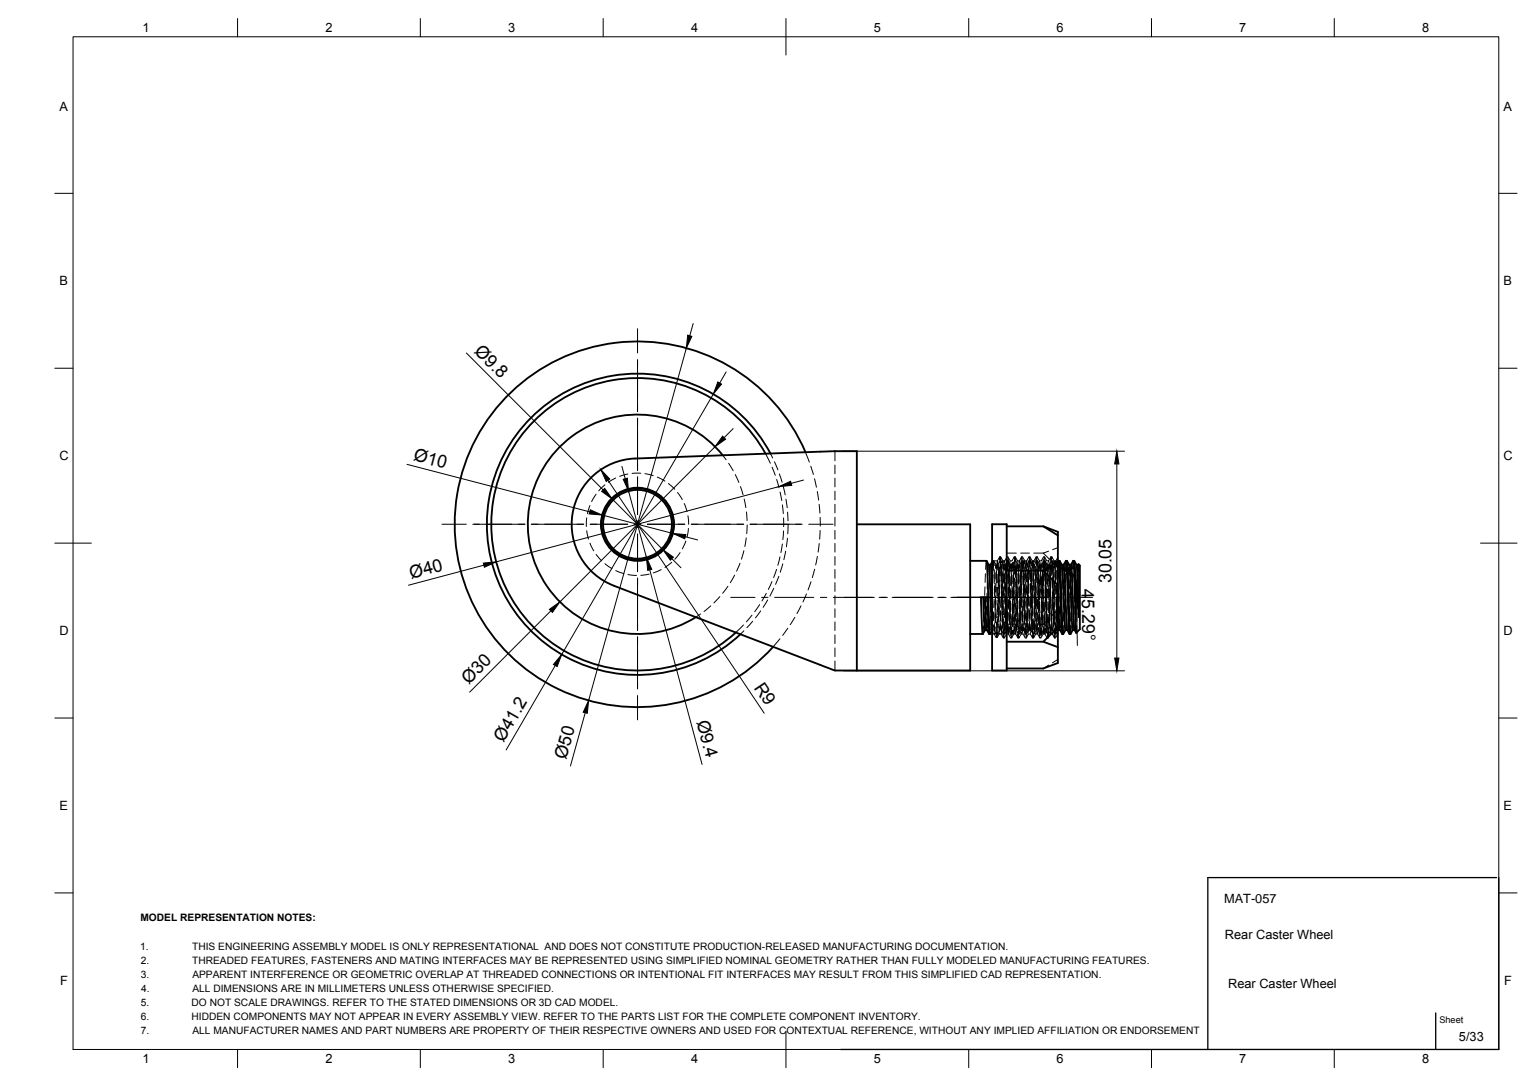
ISO-10303-21;
HEADER;
/* Generated by software containing ST-Developer
 * from STEP Tools, Inc. (www.steptools.com) 
 */

FILE_DESCRIPTION(
/* description */ ('STEP AP214', 'CAx-IF Rec.Pracs.---Representation and Presentation of Product Manufa
cturing Information (PMI)---4.0---2014-10-13'),
/* implementation_level */ '2;1');

FILE_NAME(
/* name */ 'Rear Caster Wheel.step',
/* time_stamp */ '2026-10-28T23:34:22+01:00',
/* author */ (''),
/* organization */ (''),
/* preprocessor_version */ 'ST-DEVELOPER v20.2',
/* originating_system */ 'Autodesk Translation Framework v15.17.0.0',
/* authorisation */ '');

FILE_SCHEMA (('AP242_MANAGED_MODEL_BASED_3D_ENGINEERING_MIM_LF { 1 0 10303 442 2 1 4 }'));
ENDSEC;

DATA;
#10=MECHANICAL_DESIGN_GEOMETRIC_PRESENTATION_REPRESENTATION('',(#273,#274,#275,#276),#27807);
#36=(
BOUNDED_CURVE()
B_SPLINE_CURVE(2,(#23410,#23411,#23412,#23413,#23414,#23415,#23416,#23417,
#23418),.UNSPECIFIED.,.F.,.F.)
B_SPLINE_CURVE_WITH_KNOTS((3,2,2,2,3),(0.964285714285714,0.973214285714286,
0.982142857142857,0.991071428571429,1.),.UNSPECIFIED.)
CURVE()
GEOMETRIC_REPRESENTATION_ITEM()
RATIONAL_B_SPLINE_CURVE((1.,0.923879532511287,1.,0.923879532511287,1.,0.923879532511287,
1.,0.923879532511287,1.))
REPRESENTATION_ITEM('')
);
#37=(
BOUNDED_CURVE()
B_SPLINE_CURVE(2,(#23421,#23422,#23423,#23424,#23425,#23426,#23427,#23428,
#23429),.UNSPECIFIED.,.F.,.F.)
B_SPLINE_CURVE_WITH_KNOTS((3,2,2,2,3),(0.964285714285714,0.973214285714286,
0.982142857142857,0.991071428571429,1.),.UNSPECIFIED.)
CURVE()
GEOMETRIC_REPRESENTATION_ITEM()
RATIONAL_B_SPLINE_CURVE((1.,0.923879532511287,1.,0.923879532511287,1.,0.923879532511287,
1.,0.923879532511287,1.))
REPRESENTATION_ITEM('')
);
#38=(
BOUNDED_CURVE()
B_SPLINE_CURVE(2,(#23434,#23435,#23436,#23437,#23438,#23439,#23440,#23441,
#23442,#23443,#23444,#23445,#23446,#23447,#23448,#23449,#23450),
 .UNSPECIFIED.,.F.,.F.)
B_SPLINE_CURVE_WITH_KNOTS((3,2,2,2,2,2,2,2,3),(0.892857142857143,0.901785714285714,
0.910714285714286,0.919642857142857,0.928571428571429,0.9375,0.946428571428571,
0.955357142857143,0.964285714285714),.UNSPECIFIED.)
CURVE()
GEOMETRIC_REPRESENTATION_ITEM()
RATIONAL_B_SPLINE_CURVE((1.,0.923879532511287,1.,0.923879532511287,1.,0.923879532511287,
1.,0.923879532511287,1.,0.923879532511287,1.,0.923879532511287,1.,0.923879532511287,
1.,0.923879532511287,1.))
REPRESENTATION_ITEM('')
);
#39=(
BOUNDED_CURVE()
B_SPLINE_CURVE(2,(#23451,#23452,#23453,#23454,#23455,#23456,#23457,#23458,
#23459,#23460,#23461,#23462,#23463,#23464,#23465,#23466,#23467),
 .UNSPECIFIED.,.F.,.F.)
B_SPLINE_CURVE_WITH_KNOTS((3,2,2,2,2,2,2,2,3),(0.892857142857143,0.901785714285714,
0.910714285714286,0.919642857142857,0.928571428571429,0.9375,0.946428571428571,
0.955357142857143,0.964285714285714),.UNSPECIFIED.)
CURVE()
GEOMETRIC_REPRESENTATION_ITEM()
RATIONAL_B_SPLINE_CURVE((1.,0.923879532511287,1.,0.923879532511287,1.,0.923879532511287,
1.,0.923879532511287,1.,0.923879532511287,1.,0.923879532511287,1.,0.923879532511287,
1.,0.923879532511287,1.))
REPRESENTATION_ITEM('')
);
#40=(
BOUNDED_CURVE()
B_SPLINE_CURVE(2,(#23472,#23473,#23474,#23475,#23476,#23477,#23478,#23479,
#23480,#23481,#23482,#23483,#23484,#23485,#23486,#23487,#23488),
 .UNSPECIFIED.,.F.,.F.)
B_SPLINE_CURVE_WITH_KNOTS((3,2,2,2,2,2,2,2,3),(0.821428571428571,0.830357142857143,
0.839285714285714,0.848214285714286,0.857142857142857,0.866071428571429,
0.875,0.883928571428571,0.892857142857143),.UNSPECIFIED.)
CURVE()
GEOMETRIC_REPRESENTATION_ITEM()
RATIONAL_B_SPLINE_CURVE((1.,0.923879532511287,1.,0.923879532511287,1.,0.923879532511287,
1.,0.923879532511287,1.,0.923879532511287,1.,0.923879532511287,1.,0.923879532511287,
1.,0.923879532511287,1.))
REPRESENTATION_ITEM('')
);
#41=(
BOUNDED_CURVE()
B_SPLINE_CURVE(2,(#23489,#23490,#23491,#23492,#23493,#23494,#23495,#23496,
#23497,#23498,#23499,#23500,#23501,#23502,#23503,#23504,#23505),
 .UNSPECIFIED.,.F.,.F.)
B_SPLINE_CURVE_WITH_KNOTS((3,2,2,2,2,2,2,2,3),(0.821428571428571,0.830357142857143,
0.839285714285714,0.848214285714286,0.857142857142857,0.866071428571429,
0.875,0.883928571428571,0.892857142857143),.UNSPECIFIED.)
CURVE()
GEOMETRIC_REPRESENTATION_ITEM()
RATIONAL_B_SPLINE_CURVE((1.,0.923879532511287,1.,0.923879532511287,1.,0.923879532511287,
1.,0.923879532511287,1.,0.923879532511287,1.,0.923879532511287,1.,0.923879532511287,
1.,0.923879532511287,1.))
REPRESENTATION_ITEM('')
);
#42=(
BOUNDED_CURVE()
B_SPLINE_CURVE(2,(#23510,#23511,#23512,#23513,#23514,#23515,#23516,#23517,
#23518,#23519,#23520,#23521,#23522,#23523,#23524,#23525,#23526),
 .UNSPECIFIED.,.F.,.F.)
B_SPLINE_CURVE_WITH_KNOTS((3,2,2,2,2,2,2,2,3),(0.75,0.758928571428571,0.767857142857143,
0.776785714285714,0.785714285714286,0.794642857142857,0.803571428571429,
0.8125,0.821428571428571),.UNSPECIFIED.)
CURVE()
GEOMETRIC_REPRESENTATION_ITEM()
RATIONAL_B_SPLINE_CURVE((1.,0.923879532511287,1.,0.923879532511287,1.,0.923879532511287,
1.,0.923879532511287,1.,0.923879532511287,1.,0.923879532511287,1.,0.923879532511287,
1.,0.923879532511287,1.))
REPRESENTATION_ITEM('')
);
#43=(
BOUNDED_CURVE()
B_SPLINE_CURVE(2,(#23527,#23528,#23529,#23530,#23531,#23532,#23533,#23534,
#23535,#23536,#23537,#23538,#23539,#23540,#23541,#23542,#23543),
 .UNSPECIFIED.,.F.,.F.)
B_SPLINE_CURVE_WITH_KNOTS((3,2,2,2,2,2,2,2,3),(0.75,0.758928571428571,0.767857142857143,
0.776785714285714,0.785714285714286,0.794642857142857,0.803571428571429,
0.8125,0.821428571428571),.UNSPECIFIED.)
CURVE()
GEOMETRIC_REPRESENTATION_ITEM()
RATIONAL_B_SPLINE_CURVE((1.,0.923879532511287,1.,0.923879532511287,1.,0.923879532511287,
1.,0.923879532511287,1.,0.923879532511287,1.,0.923879532511287,1.,0.923879532511287,
1.,0.923879532511287,1.))
REPRESENTATION_ITEM('')
);
#44=(
BOUNDED_CURVE()
B_SPLINE_CURVE(2,(#23548,#23549,#23550,#23551,#23552,#23553,#23554,#23555,
#23556,#23557,#23558,#23559,#23560,#23561,#23562,#23563,#23564),
 .UNSPECIFIED.,.F.,.F.)
B_SPLINE_CURVE_WITH_KNOTS((3,2,2,2,2,2,2,2,3),(0.678571428571429,0.6875,
0.696428571428571,0.705357142857143,0.714285714285714,0.723214285714286,
0.732142857142857,0.741071428571429,0.75),.UNSPECIFIED.)
CURVE()
GEOMETRIC_REPRESENTATION_ITEM()
RATIONAL_B_SPLINE_CURVE((1.,0.923879532511287,1.,0.923879532511287,1.,0.923879532511287,
1.,0.923879532511287,1.,0.923879532511287,1.,0.923879532511287,1.,0.923879532511287,
1.,0.923879532511287,1.))
REPRESENTATION_ITEM('')
);
#45=(
BOUNDED_CURVE()
B_SPLINE_CURVE(2,(#23565,#23566,#23567,#23568,#23569,#23570,#23571,#23572,
#23573,#23574,#23575,#23576,#23577,#23578,#23579,#23580,#23581),
 .UNSPECIFIED.,.F.,.F.)
B_SPLINE_CURVE_WITH_KNOTS((3,2,2,2,2,2,2,2,3),(0.678571428571428,0.6875,
0.696428571428571,0.705357142857143,0.714285714285714,0.723214285714286,
0.732142857142857,0.741071428571429,0.75),.UNSPECIFIED.)
CURVE()
GEOMETRIC_REPRESENTATION_ITEM()
RATIONAL_B_SPLINE_CURVE((1.,0.923879532511287,1.,0.923879532511287,1.,0.923879532511287,
1.,0.923879532511287,1.,0.923879532511287,1.,0.923879532511287,1.,0.923879532511287,
1.,0.923879532511287,1.))
REPRESENTATION_ITEM('')
);
#46=(
BOUNDED_CURVE()
B_SPLINE_CURVE(2,(#23586,#23587,#23588,#23589,#23590,#23591,#23592,#23593,
#23594,#23595,#23596,#23597,#23598,#23599,#23600,#23601,#23602),
 .UNSPECIFIED.,.F.,.F.)
B_SPLINE_CURVE_WITH_KNOTS((3,2,2,2,2,2,2,2,3),(0.607142857142857,0.616071428571429,
0.625,0.633928571428571,0.642857142857143,0.651785714285714,0.660714285714286,
0.669642857142857,0.678571428571429),.UNSPECIFIED.)
CURVE()
GEOMETRIC_REPRESENTATION_ITEM()
RATIONAL_B_SPLINE_CURVE((1.,0.923879532511287,1.,0.923879532511287,1.,0.923879532511287,
1.,0.923879532511287,1.,0.923879532511287,1.,0.923879532511287,1.,0.923879532511287,
1.,0.923879532511287,1.))
REPRESENTATION_ITEM('')
);
#47=(
BOUNDED_CURVE()
B_SPLINE_CURVE(2,(#23603,#23604,#23605,#23606,#23607,#23608,#23609,#23610,
#23611,#23612,#23613,#23614,#23615,#23616,#23617,#23618,#23619),
 .UNSPECIFIED.,.F.,.F.)
B_SPLINE_CURVE_WITH_KNOTS((3,2,2,2,2,2,2,2,3),(0.607142857142857,0.616071428571429,
0.625,0.633928571428571,0.642857142857143,0.651785714285714,0.660714285714286,
0.669642857142857,0.678571428571428),.UNSPECIFIED.)
CURVE()
GEOMETRIC_REPRESENTATION_ITEM()
RATIONAL_B_SPLINE_CURVE((1.,0.923879532511287,1.,0.923879532511287,1.,0.923879532511287,
1.,0.923879532511287,1.,0.923879532511287,1.,0.923879532511287,1.,0.923879532511287,
1.,0.923879532511287,1.))
REPRESENTATION_ITEM('')
);
#48=(
BOUNDED_CURVE()
B_SPLINE_CURVE(2,(#23624,#23625,#23626,#23627,#23628,#23629,#23630,#23631,
#23632,#23633,#23634,#23635,#23636,#23637,#23638,#23639,#23640),
 .UNSPECIFIED.,.F.,.F.)
B_SPLINE_CURVE_WITH_KNOTS((3,2,2,2,2,2,2,2,3),(0.535714285714286,0.544642857142857,
0.553571428571429,0.5625,0.571428571428571,0.580357142857143,0.589285714285714,
0.598214285714286,0.607142857142857),.UNSPECIFIED.)
CURVE()
GEOMETRIC_REPRESENTATION_ITEM()
RATIONAL_B_SPLINE_CURVE((1.,0.923879532511287,1.,0.923879532511287,1.,0.923879532511287,
1.,0.923879532511287,1.,0.923879532511287,1.,0.923879532511287,1.,0.923879532511287,
1.,0.923879532511287,1.))
REPRESENTATION_ITEM('')
);
#49=(
BOUNDED_CURVE()
B_SPLINE_CURVE(2,(#23641,#23642,#23643,#23644,#23645,#23646,#23647,#23648,
#23649,#23650,#23651,#23652,#23653,#23654,#23655,#23656,#23657),
 .UNSPECIFIED.,.F.,.F.)
B_SPLINE_CURVE_WITH_KNOTS((3,2,2,2,2,2,2,2,3),(0.535714285714286,0.544642857142857,
0.553571428571429,0.5625,0.571428571428571,0.580357142857143,0.589285714285714,
0.598214285714286,0.607142857142857),.UNSPECIFIED.)
CURVE()
GEOMETRIC_REPRESENTATION_ITEM()
RATIONAL_B_SPLINE_CURVE((1.,0.923879532511287,1.,0.923879532511287,1.,0.923879532511287,
1.,0.923879532511287,1.,0.923879532511287,1.,0.923879532511287,1.,0.923879532511287,
1.,0.923879532511287,1.))
REPRESENTATION_ITEM('')
);
#50=(
BOUNDED_CURVE()
B_SPLINE_CURVE(2,(#23662,#23663,#23664,#23665,#23666,#23667,#23668,#23669,
#23670,#23671,#23672,#23673,#23674,#23675,#23676,#23677,#23678),
 .UNSPECIFIED.,.F.,.F.)
B_SPLINE_CURVE_WITH_KNOTS((3,2,2,2,2,2,2,2,3),(0.464285714285714,0.473214285714286,
0.482142857142857,0.491071428571429,0.5,0.508928571428571,0.517857142857143,
0.526785714285714,0.535714285714286),.UNSPECIFIED.)
CURVE()
GEOMETRIC_REPRESENTATION_ITEM()
RATIONAL_B_SPLINE_CURVE((1.,0.923879532511287,1.,0.923879532511287,1.,0.923879532511287,
1.,0.923879532511287,1.,0.923879532511287,1.,0.923879532511287,1.,0.923879532511287,
1.,0.923879532511287,1.))
REPRESENTATION_ITEM('')
);
#51=(
BOUNDED_CURVE()
B_SPLINE_CURVE(2,(#23679,#23680,#23681,#23682,#23683,#23684,#23685,#23686,
#23687,#23688,#23689,#23690,#23691,#23692,#23693,#23694,#23695),
 .UNSPECIFIED.,.F.,.F.)
B_SPLINE_CURVE_WITH_KNOTS((3,2,2,2,2,2,2,2,3),(0.464285714285714,0.473214285714286,
0.482142857142857,0.491071428571429,0.5,0.508928571428571,0.517857142857143,
0.526785714285714,0.535714285714286),.UNSPECIFIED.)
CURVE()
GEOMETRIC_REPRESENTATION_ITEM()
RATIONAL_B_SPLINE_CURVE((1.,0.923879532511287,1.,0.923879532511287,1.,0.923879532511287,
1.,0.923879532511287,1.,0.923879532511287,1.,0.923879532511287,1.,0.923879532511287,
1.,0.923879532511287,1.))
REPRESENTATION_ITEM('')
);
#52=(
BOUNDED_CURVE()
B_SPLINE_CURVE(2,(#23700,#23701,#23702,#23703,#23704,#23705,#23706,#23707,
#23708,#23709,#23710,#23711,#23712,#23713,#23714,#23715,#23716),
 .UNSPECIFIED.,.F.,.F.)
B_SPLINE_CURVE_WITH_KNOTS((3,2,2,2,2,2,2,2,3),(0.392857142857143,0.401785714285714,
0.410714285714286,0.419642857142857,0.428571428571429,0.4375,0.446428571428571,
0.455357142857143,0.464285714285714),.UNSPECIFIED.)
CURVE()
GEOMETRIC_REPRESENTATION_ITEM()
RATIONAL_B_SPLINE_CURVE((1.,0.923879532511287,1.,0.923879532511287,1.,0.923879532511287,
1.,0.923879532511287,1.,0.923879532511287,1.,0.923879532511287,1.,0.923879532511287,
1.,0.923879532511287,1.))
REPRESENTATION_ITEM('')
);
#53=(
BOUNDED_CURVE()
B_SPLINE_CURVE(2,(#23717,#23718,#23719,#23720,#23721,#23722,#23723,#23724,
#23725,#23726,#23727,#23728,#23729,#23730,#23731,#23732,#23733),
 .UNSPECIFIED.,.F.,.F.)
B_SPLINE_CURVE_WITH_KNOTS((3,2,2,2,2,2,2,2,3),(0.392857142857143,0.401785714285714,
0.410714285714286,0.419642857142857,0.428571428571429,0.4375,0.446428571428571,
0.455357142857143,0.464285714285714),.UNSPECIFIED.)
CURVE()
GEOMETRIC_REPRESENTATION_ITEM()
RATIONAL_B_SPLINE_CURVE((1.,0.923879532511287,1.,0.923879532511287,1.,0.923879532511287,
1.,0.923879532511287,1.,0.923879532511287,1.,0.923879532511287,1.,0.923879532511287,
1.,0.923879532511287,1.))
REPRESENTATION_ITEM('')
);
#54=(
BOUNDED_CURVE()
B_SPLINE_CURVE(2,(#23738,#23739,#23740,#23741,#23742,#23743,#23744,#23745,
#23746,#23747,#23748,#23749,#23750,#23751,#23752,#23753,#23754),
 .UNSPECIFIED.,.F.,.F.)
B_SPLINE_CURVE_WITH_KNOTS((3,2,2,2,2,2,2,2,3),(0.321428571428571,0.330357142857143,
0.339285714285714,0.348214285714286,0.357142857142857,0.366071428571429,
0.375,0.383928571428571,0.392857142857143),.UNSPECIFIED.)
CURVE()
GEOMETRIC_REPRESENTATION_ITEM()
RATIONAL_B_SPLINE_CURVE((1.,0.923879532511287,1.,0.923879532511287,1.,0.923879532511287,
1.,0.923879532511287,1.,0.923879532511287,1.,0.923879532511287,1.,0.923879532511287,
1.,0.923879532511287,1.))
REPRESENTATION_ITEM('')
);
#55=(
BOUNDED_CURVE()
B_SPLINE_CURVE(2,(#23755,#23756,#23757,#23758,#23759,#23760,#23761,#23762,
#23763,#23764,#23765,#23766,#23767,#23768,#23769,#23770,#23771),
 .UNSPECIFIED.,.F.,.F.)
B_SPLINE_CURVE_WITH_KNOTS((3,2,2,2,2,2,2,2,3),(0.321428571428571,0.330357142857143,
0.339285714285714,0.348214285714286,0.357142857142857,0.366071428571429,
0.375,0.383928571428571,0.392857142857143),.UNSPECIFIED.)
CURVE()
GEOMETRIC_REPRESENTATION_ITEM()
RATIONAL_B_SPLINE_CURVE((1.,0.923879532511287,1.,0.923879532511287,1.,0.923879532511287,
1.,0.923879532511287,1.,0.923879532511287,1.,0.923879532511287,1.,0.923879532511287,
1.,0.923879532511287,1.))
REPRESENTATION_ITEM('')
);
#56=(
BOUNDED_CURVE()
B_SPLINE_CURVE(2,(#23776,#23777,#23778,#23779,#23780,#23781,#23782,#23783,
#23784,#23785,#23786,#23787,#23788,#23789,#23790,#23791,#23792),
 .UNSPECIFIED.,.F.,.F.)
B_SPLINE_CURVE_WITH_KNOTS((3,2,2,2,2,2,2,2,3),(0.25,0.258928571428571,0.267857142857143,
0.276785714285714,0.285714285714286,0.294642857142857,0.303571428571429,
0.3125,0.321428571428571),.UNSPECIFIED.)
CURVE()
GEOMETRIC_REPRESENTATION_ITEM()
RATIONAL_B_SPLINE_CURVE((1.,0.923879532511287,1.,0.923879532511287,1.,0.923879532511287,
1.,0.923879532511287,1.,0.923879532511287,1.,0.923879532511287,1.,0.923879532511287,
1.,0.923879532511287,1.))
REPRESENTATION_ITEM('')
);
#57=(
BOUNDED_CURVE()
B_SPLINE_CURVE(2,(#23793,#23794,#23795,#23796,#23797,#23798,#23799,#23800,
#23801,#23802,#23803,#23804,#23805,#23806,#23807,#23808,#23809),
 .UNSPECIFIED.,.F.,.F.)
B_SPLINE_CURVE_WITH_KNOTS((3,2,2,2,2,2,2,2,3),(0.25,0.258928571428571,0.267857142857143,
0.276785714285714,0.285714285714286,0.294642857142857,0.303571428571429,
0.3125,0.321428571428571),.UNSPECIFIED.)
CURVE()
GEOMETRIC_REPRESENTATION_ITEM()
RATIONAL_B_SPLINE_CURVE((1.,0.923879532511287,1.,0.923879532511287,1.,0.923879532511287,
1.,0.923879532511287,1.,0.923879532511287,1.,0.923879532511287,1.,0.923879532511287,
1.,0.923879532511287,1.))
REPRESENTATION_ITEM('')
);
#58=(
BOUNDED_CURVE()
B_SPLINE_CURVE(2,(#23814,#23815,#23816,#23817,#23818,#23819,#23820,#23821,
#23822,#23823,#23824,#23825,#23826,#23827,#23828,#23829,#23830),
 .UNSPECIFIED.,.F.,.F.)
B_SPLINE_CURVE_WITH_KNOTS((3,2,2,2,2,2,2,2,3),(0.178571428571429,0.1875,
0.196428571428571,0.205357142857143,0.214285714285714,0.223214285714286,
0.232142857142857,0.241071428571429,0.25),.UNSPECIFIED.)
CURVE()
GEOMETRIC_REPRESENTATION_ITEM()
RATIONAL_B_SPLINE_CURVE((1.,0.923879532511287,1.,0.923879532511287,1.,0.923879532511287,
1.,0.923879532511287,1.,0.923879532511287,1.,0.923879532511287,1.,0.923879532511287,
1.,0.923879532511287,1.))
REPRESENTATION_ITEM('')
);
#59=(
BOUNDED_CURVE()
B_SPLINE_CURVE(2,(#23831,#23832,#23833,#23834,#23835,#23836,#23837,#23838,
#23839,#23840,#23841,#23842,#23843,#23844,#23845,#23846,#23847),
 .UNSPECIFIED.,.F.,.F.)
B_SPLINE_CURVE_WITH_KNOTS((3,2,2,2,2,2,2,2,3),(0.178571428571429,0.1875,
0.196428571428571,0.205357142857143,0.214285714285714,0.223214285714286,
0.232142857142857,0.241071428571429,0.25),.UNSPECIFIED.)
CURVE()
GEOMETRIC_REPRESENTATION_ITEM()
RATIONAL_B_SPLINE_CURVE((1.,0.923879532511287,1.,0.923879532511287,1.,0.923879532511287,
1.,0.923879532511287,1.,0.923879532511287,1.,0.923879532511287,1.,0.923879532511287,
1.,0.923879532511287,1.))
REPRESENTATION_ITEM('')
);
#60=(
BOUNDED_CURVE()
B_SPLINE_CURVE(2,(#23852,#23853,#23854,#23855,#23856,#23857,#23858,#23859,
#23860,#23861,#23862,#23863,#23864,#23865,#23866,#23867,#23868),
 .UNSPECIFIED.,.F.,.F.)
B_SPLINE_CURVE_WITH_KNOTS((3,2,2,2,2,2,2,2,3),(0.107142857142857,0.116071428571429,
0.125,0.133928571428571,0.142857142857143,0.151785714285714,0.160714285714286,
0.169642857142857,0.178571428571429),.UNSPECIFIED.)
CURVE()
GEOMETRIC_REPRESENTATION_ITEM()
RATIONAL_B_SPLINE_CURVE((1.,0.923879532511287,1.,0.923879532511287,1.,0.923879532511287,
1.,0.923879532511287,1.,0.923879532511287,1.,0.923879532511287,1.,0.923879532511287,
1.,0.923879532511287,1.))
REPRESENTATION_ITEM('')
);
#61=(
BOUNDED_CURVE()
B_SPLINE_CURVE(2,(#23869,#23870,#23871,#23872,#23873,#23874,#23875,#23876,
#23877,#23878,#23879,#23880,#23881,#23882,#23883,#23884,#23885),
 .UNSPECIFIED.,.F.,.F.)
B_SPLINE_CURVE_WITH_KNOTS((3,2,2,2,2,2,2,2,3),(0.107142857142857,0.116071428571429,
0.125,0.133928571428571,0.142857142857143,0.151785714285714,0.160714285714286,
0.169642857142857,0.178571428571429),.UNSPECIFIED.)
CURVE()
GEOMETRIC_REPRESENTATION_ITEM()
RATIONAL_B_SPLINE_CURVE((1.,0.923879532511287,1.,0.923879532511287,1.,0.923879532511287,
1.,0.923879532511287,1.,0.923879532511287,1.,0.923879532511287,1.,0.923879532511287,
1.,0.923879532511287,1.))
REPRESENTATION_ITEM('')
);
#62=(
BOUNDED_CURVE()
B_SPLINE_CURVE(2,(#25481,#25482,#25483,#25484,#25485,#25486,#25487),
 .UNSPECIFIED.,.F.,.F.)
B_SPLINE_CURVE_WITH_KNOTS((3,2,2,3),(0.0819392927096003,0.0892857142857143,
0.0982142857142857,0.107142857142857),.UNSPECIFIED.)
CURVE()
GEOMETRIC_REPRESENTATION_ITEM()
RATIONAL_B_SPLINE_CURVE((0.977803170316603,0.937368138988787,1.,0.923879532511287,
1.,0.923879532511287,1.))
REPRESENTATION_ITEM('')
);
#63=(
BOUNDED_CURVE()
B_SPLINE_CURVE(2,(#25489,#25490,#25491,#25492,#25493,#25494,#25495,#25496,
#25497,#25498,#25499),.UNSPECIFIED.,.F.,.F.)
B_SPLINE_CURVE_WITH_KNOTS((3,2,2,2,2,3),(0.0640821498524563,0.0714285714285714,
0.0803571428571429,0.0892857142857143,0.0982142857142857,0.107142857142857),
 .UNSPECIFIED.)
CURVE()
GEOMETRIC_REPRESENTATION_ITEM()
RATIONAL_B_SPLINE_CURVE((0.977803170316615,0.937368138988778,1.,0.923879532511287,
1.,0.923879532511287,1.,0.923879532511287,1.,0.923879532511287,1.))
REPRESENTATION_ITEM('')
);
#64=(
BOUNDED_CURVE()
B_SPLINE_CURVE(2,(#25959,#25960,#25961,#25962,#25963,#25964,#25965,#25966,
#25967,#25968,#25969,#25970,#25971,#25972,#25973),.UNSPECIFIED.,.F.,.F.)
B_SPLINE_CURVE_WITH_KNOTS((3,2,2,2,2,2,2,3),(0.168750000131362,0.175,0.1875,
0.2,0.2125,0.225,0.2375,0.25),.UNSPECIFIED.)
CURVE()
GEOMETRIC_REPRESENTATION_ITEM()
RATIONAL_B_SPLINE_CURVE((0.961939766255643,0.961939767055589,1.,0.923879532511287,
1.,0.923879532511287,1.,0.923879532511287,1.,0.923879532511287,1.,0.923879532511287,
1.,0.923879532511287,1.))
REPRESENTATION_ITEM('')
);
#65=(
BOUNDED_CURVE()
B_SPLINE_CURVE(2,(#25976,#25977,#25978,#25979,#25980,#25981,#25982,#25983,
#25984,#25985,#25986,#25987,#25988,#25989,#25990,#25991,#25992),
 .UNSPECIFIED.,.F.,.F.)
B_SPLINE_CURVE_WITH_KNOTS((3,2,2,2,2,2,2,2,3),(0.156250000131362,0.1625,
0.175,0.1875,0.2,0.2125,0.225,0.2375,0.25),.UNSPECIFIED.)
CURVE()
GEOMETRIC_REPRESENTATION_ITEM()
RATIONAL_B_SPLINE_CURVE((0.961939766255643,0.961939767055589,1.,0.923879532511287,
1.,0.923879532511287,1.,0.923879532511287,1.,0.923879532511287,1.,0.923879532511287,
1.,0.923879532511287,1.,0.923879532511287,1.))
REPRESENTATION_ITEM('')
);
#66=(
BOUNDED_CURVE()
B_SPLINE_CURVE(2,(#25997,#25998,#25999,#26000,#26001,#26002,#26003,#26004,
#26005,#26006,#26007,#26008,#26009,#26010,#26011,#26012,#26013),
 .UNSPECIFIED.,.F.,.F.)
B_SPLINE_CURVE_WITH_KNOTS((3,2,2,2,2,2,2,2,3),(0.25,0.2625,0.275,0.2875,
0.3,0.3125,0.325,0.3375,0.35),.UNSPECIFIED.)
CURVE()
GEOMETRIC_REPRESENTATION_ITEM()
RATIONAL_B_SPLINE_CURVE((1.,0.923879532511287,1.,0.923879532511287,1.,0.923879532511287,
1.,0.923879532511287,1.,0.923879532511287,1.,0.923879532511287,1.,0.923879532511287,
1.,0.923879532511287,1.))
REPRESENTATION_ITEM('')
);
#67=(
BOUNDED_CURVE()
B_SPLINE_CURVE(2,(#26014,#26015,#26016,#26017,#26018,#26019,#26020,#26021,
#26022,#26023,#26024,#26025,#26026,#26027,#26028,#26029,#26030),
 .UNSPECIFIED.,.F.,.F.)
B_SPLINE_CURVE_WITH_KNOTS((3,2,2,2,2,2,2,2,3),(0.25,0.2625,0.275,0.2875,
0.3,0.3125,0.325,0.3375,0.35),.UNSPECIFIED.)
CURVE()
GEOMETRIC_REPRESENTATION_ITEM()
RATIONAL_B_SPLINE_CURVE((1.,0.923879532511287,1.,0.923879532511287,1.,0.923879532511287,
1.,0.923879532511287,1.,0.923879532511287,1.,0.923879532511287,1.,0.923879532511287,
1.,0.923879532511287,1.))
REPRESENTATION_ITEM('')
);
#68=(
BOUNDED_CURVE()
B_SPLINE_CURVE(2,(#26035,#26036,#26037,#26038,#26039,#26040,#26041,#26042,
#26043,#26044,#26045,#26046,#26047,#26048,#26049,#26050,#26051),
 .UNSPECIFIED.,.F.,.F.)
B_SPLINE_CURVE_WITH_KNOTS((3,2,2,2,2,2,2,2,3),(0.35,0.3625,0.375,0.3875,
0.4,0.4125,0.425,0.4375,0.45),.UNSPECIFIED.)
CURVE()
GEOMETRIC_REPRESENTATION_ITEM()
RATIONAL_B_SPLINE_CURVE((1.,0.923879532511287,1.,0.923879532511287,1.,0.923879532511287,
1.,0.923879532511287,1.,0.923879532511287,1.,0.923879532511287,1.,0.923879532511287,
1.,0.923879532511287,1.))
REPRESENTATION_ITEM('')
);
#69=(
BOUNDED_CURVE()
B_SPLINE_CURVE(2,(#26052,#26053,#26054,#26055,#26056,#26057,#26058,#26059,
#26060,#26061,#26062,#26063,#26064,#26065,#26066,#26067,#26068),
 .UNSPECIFIED.,.F.,.F.)
B_SPLINE_CURVE_WITH_KNOTS((3,2,2,2,2,2,2,2,3),(0.35,0.3625,0.375,0.3875,
0.4,0.4125,0.425,0.4375,0.45),.UNSPECIFIED.)
CURVE()
GEOMETRIC_REPRESENTATION_ITEM()
RATIONAL_B_SPLINE_CURVE((1.,0.923879532511287,1.,0.923879532511287,1.,0.923879532511287,
1.,0.923879532511287,1.,0.923879532511287,1.,0.923879532511287,1.,0.923879532511287,
1.,0.923879532511287,1.))
REPRESENTATION_ITEM('')
);
#70=(
BOUNDED_CURVE()
B_SPLINE_CURVE(2,(#26073,#26074,#26075,#26076,#26077,#26078,#26079,#26080,
#26081,#26082,#26083,#26084,#26085,#26086,#26087,#26088,#26089),
 .UNSPECIFIED.,.F.,.F.)
B_SPLINE_CURVE_WITH_KNOTS((3,2,2,2,2,2,2,2,3),(0.45,0.4625,0.475,0.4875,
0.5,0.5125,0.525,0.5375,0.55),.UNSPECIFIED.)
CURVE()
GEOMETRIC_REPRESENTATION_ITEM()
RATIONAL_B_SPLINE_CURVE((1.,0.923879532511287,1.,0.923879532511287,1.,0.923879532511287,
1.,0.923879532511287,1.,0.923879532511287,1.,0.923879532511287,1.,0.923879532511287,
1.,0.923879532511287,1.))
REPRESENTATION_ITEM('')
);
#71=(
BOUNDED_CURVE()
B_SPLINE_CURVE(2,(#26090,#26091,#26092,#26093,#26094,#26095,#26096,#26097,
#26098,#26099,#26100,#26101,#26102,#26103,#26104,#26105,#26106),
 .UNSPECIFIED.,.F.,.F.)
B_SPLINE_CURVE_WITH_KNOTS((3,2,2,2,2,2,2,2,3),(0.45,0.4625,0.475,0.4875,
0.5,0.5125,0.525,0.5375,0.55),.UNSPECIFIED.)
CURVE()
GEOMETRIC_REPRESENTATION_ITEM()
RATIONAL_B_SPLINE_CURVE((1.,0.923879532511287,1.,0.923879532511287,1.,0.923879532511287,
1.,0.923879532511287,1.,0.923879532511287,1.,0.923879532511287,1.,0.923879532511287,
1.,0.923879532511287,1.))
REPRESENTATION_ITEM('')
);
#72=(
BOUNDED_CURVE()
B_SPLINE_CURVE(2,(#26111,#26112,#26113,#26114,#26115,#26116,#26117,#26118,
#26119,#26120,#26121,#26122,#26123,#26124,#26125,#26126,#26127),
 .UNSPECIFIED.,.F.,.F.)
B_SPLINE_CURVE_WITH_KNOTS((3,2,2,2,2,2,2,2,3),(0.55,0.5625,0.575,0.5875,
0.6,0.6125,0.625,0.6375,0.65),.UNSPECIFIED.)
CURVE()
GEOMETRIC_REPRESENTATION_ITEM()
RATIONAL_B_SPLINE_CURVE((1.,0.923879532511287,1.,0.923879532511287,1.,0.923879532511287,
1.,0.923879532511287,1.,0.923879532511287,1.,0.923879532511287,1.,0.923879532511287,
1.,0.923879532511287,1.))
REPRESENTATION_ITEM('')
);
#73=(
BOUNDED_CURVE()
B_SPLINE_CURVE(2,(#26128,#26129,#26130,#26131,#26132,#26133,#26134,#26135,
#26136,#26137,#26138,#26139,#26140,#26141,#26142,#26143,#26144),
 .UNSPECIFIED.,.F.,.F.)
B_SPLINE_CURVE_WITH_KNOTS((3,2,2,2,2,2,2,2,3),(0.55,0.5625,0.575,0.5875,
0.6,0.6125,0.625,0.6375,0.65),.UNSPECIFIED.)
CURVE()
GEOMETRIC_REPRESENTATION_ITEM()
RATIONAL_B_SPLINE_CURVE((1.,0.923879532511287,1.,0.923879532511287,1.,0.923879532511287,
1.,0.923879532511287,1.,0.923879532511287,1.,0.923879532511287,1.,0.923879532511287,
1.,0.923879532511287,1.))
REPRESENTATION_ITEM('')
);
#74=(
BOUNDED_CURVE()
B_SPLINE_CURVE(2,(#26149,#26150,#26151,#26152,#26153,#26154,#26155,#26156,
#26157,#26158,#26159,#26160,#26161,#26162,#26163,#26164,#26165),
 .UNSPECIFIED.,.F.,.F.)
B_SPLINE_CURVE_WITH_KNOTS((3,2,2,2,2,2,2,2,3),(0.65,0.6625,0.675,0.6875,
0.7,0.7125,0.725,0.7375,0.75),.UNSPECIFIED.)
CURVE()
GEOMETRIC_REPRESENTATION_ITEM()
RATIONAL_B_SPLINE_CURVE((1.,0.923879532511287,1.,0.923879532511287,1.,0.923879532511287,
1.,0.923879532511287,1.,0.923879532511287,1.,0.923879532511287,1.,0.923879532511287,
1.,0.923879532511287,1.))
REPRESENTATION_ITEM('')
);
#75=(
BOUNDED_CURVE()
B_SPLINE_CURVE(2,(#26166,#26167,#26168,#26169,#26170,#26171,#26172,#26173,
#26174,#26175,#26176,#26177,#26178,#26179,#26180,#26181,#26182),
 .UNSPECIFIED.,.F.,.F.)
B_SPLINE_CURVE_WITH_KNOTS((3,2,2,2,2,2,2,2,3),(0.65,0.6625,0.675,0.6875,
0.7,0.7125,0.725,0.7375,0.75),.UNSPECIFIED.)
CURVE()
GEOMETRIC_REPRESENTATION_ITEM()
RATIONAL_B_SPLINE_CURVE((1.,0.923879532511287,1.,0.923879532511287,1.,0.923879532511287,
1.,0.923879532511287,1.,0.923879532511287,1.,0.923879532511287,1.,0.923879532511287,
1.,0.923879532511287,1.))
REPRESENTATION_ITEM('')
);
#76=(
BOUNDED_CURVE()
B_SPLINE_CURVE(2,(#26187,#26188,#26189,#26190,#26191,#26192,#26193,#26194,
#26195,#26196,#26197,#26198,#26199,#26200,#26201,#26202,#26203),
 .UNSPECIFIED.,.F.,.F.)
B_SPLINE_CURVE_WITH_KNOTS((3,2,2,2,2,2,2,2,3),(0.75,0.7625,0.775,0.7875,
0.8,0.8125,0.825,0.8375,0.85),.UNSPECIFIED.)
CURVE()
GEOMETRIC_REPRESENTATION_ITEM()
RATIONAL_B_SPLINE_CURVE((1.,0.923879532511287,1.,0.923879532511287,1.,0.923879532511287,
1.,0.923879532511287,1.,0.923879532511287,1.,0.923879532511287,1.,0.923879532511287,
1.,0.923879532511287,1.))
REPRESENTATION_ITEM('')
);
#77=(
BOUNDED_CURVE()
B_SPLINE_CURVE(2,(#26204,#26205,#26206,#26207,#26208,#26209,#26210,#26211,
#26212,#26213,#26214,#26215,#26216,#26217,#26218,#26219,#26220),
 .UNSPECIFIED.,.F.,.F.)
B_SPLINE_CURVE_WITH_KNOTS((3,2,2,2,2,2,2,2,3),(0.75,0.7625,0.775,0.7875,
0.8,0.8125,0.825,0.8375,0.85),.UNSPECIFIED.)
CURVE()
GEOMETRIC_REPRESENTATION_ITEM()
RATIONAL_B_SPLINE_CURVE((1.,0.923879532511287,1.,0.923879532511287,1.,0.923879532511287,
1.,0.923879532511287,1.,0.923879532511287,1.,0.923879532511287,1.,0.923879532511287,
1.,0.923879532511287,1.))
REPRESENTATION_ITEM('')
);
#78=(
BOUNDED_CURVE()
B_SPLINE_CURVE(2,(#26226,#26227,#26228,#26229,#26230,#26231,#26232,#26233,
#26234),.UNSPECIFIED.,.F.,.F.)
B_SPLINE_CURVE_WITH_KNOTS((3,2,2,2,3),(0.95,0.9625,0.975,0.9875,1.),
 .UNSPECIFIED.)
CURVE()
GEOMETRIC_REPRESENTATION_ITEM()
RATIONAL_B_SPLINE_CURVE((1.,0.923879532511287,1.,0.923879532511287,1.,0.923879532511287,
1.,0.923879532511287,1.))
REPRESENTATION_ITEM('')
);
#79=(
BOUNDED_CURVE()
B_SPLINE_CURVE(2,(#26237,#26238,#26239,#26240,#26241,#26242,#26243,#26244,
#26245),.UNSPECIFIED.,.F.,.F.)
B_SPLINE_CURVE_WITH_KNOTS((3,2,2,2,3),(0.95,0.9625,0.975,0.9875,1.),
 .UNSPECIFIED.)
CURVE()
GEOMETRIC_REPRESENTATION_ITEM()
RATIONAL_B_SPLINE_CURVE((1.,0.923879532511287,1.,0.923879532511287,1.,0.923879532511287,
1.,0.923879532511287,1.))
REPRESENTATION_ITEM('')
);
#80=(
BOUNDED_CURVE()
B_SPLINE_CURVE(2,(#27008,#27009,#27010,#27011,#27012,#27013,#27014,#27015,
#27016,#27017,#27018,#27019,#27020,#27021,#27022,#27023,#27024),
 .UNSPECIFIED.,.F.,.F.)
B_SPLINE_CURVE_WITH_KNOTS((3,2,2,2,2,2,2,2,3),(0.85,0.8625,0.875,0.8875,
0.9,0.9125,0.925,0.9375,0.95),.UNSPECIFIED.)
CURVE()
GEOMETRIC_REPRESENTATION_ITEM()
RATIONAL_B_SPLINE_CURVE((1.,0.923879532511287,1.,0.923879532511287,1.,0.923879532511287,
1.,0.923879532511287,1.,0.923879532511287,1.,0.923879532511287,1.,0.923879532511287,
1.,0.923879532511287,1.))
REPRESENTATION_ITEM('')
);
#81=(
BOUNDED_CURVE()
B_SPLINE_CURVE(2,(#27025,#27026,#27027,#27028,#27029,#27030,#27031,#27032,
#27033,#27034,#27035,#27036,#27037,#27038,#27039,#27040,#27041),
 .UNSPECIFIED.,.F.,.F.)
B_SPLINE_CURVE_WITH_KNOTS((3,2,2,2,2,2,2,2,3),(0.85,0.8625,0.875,0.8875,
0.9,0.9125,0.925,0.9375,0.95),.UNSPECIFIED.)
CURVE()
GEOMETRIC_REPRESENTATION_ITEM()
RATIONAL_B_SPLINE_CURVE((1.,0.923879532511287,1.,0.923879532511287,1.,0.923879532511287,
1.,0.923879532511287,1.,0.923879532511287,1.,0.923879532511287,1.,0.923879532511287,
1.,0.923879532511287,1.))
REPRESENTATION_ITEM('')
);
#225=SHAPE_REPRESENTATION_RELATIONSHIP('SRR','None',#27924,#247);
#247=ADVANCED_BREP_SHAPE_REPRESENTATION('',(#302,#303,#304,#305),#27804);
#273=STYLED_ITEM('',(#28091),#302);
#274=STYLED_ITEM('',(#28091),#303);
#275=STYLED_ITEM('',(#28091),#304);
#276=STYLED_ITEM('',(#28091),#305);
#302=MANIFOLD_SOLID_BREP('Body1',#12049);
#303=MANIFOLD_SOLID_BREP('Body2',#12050);
#304=MANIFOLD_SOLID_BREP('Body3',#12051);
#305=MANIFOLD_SOLID_BREP('Body4',#12052);
#323=(
BOUNDED_SURFACE()
B_SPLINE_SURFACE(1,2,((#25031,#25032,#25033,#25034,#25035,#25036,#25037,
#25038,#25039,#25040,#25041,#25042,#25043,#25044,#25045,#25046,#25047,#25048,
#25049,#25050,#25051,#25052,#25053,#25054,#25055,#25056,#25057,#25058,#25059,
#25060,#25061,#25062,#25063,#25064,#25065,#25066,#25067,#25068,#25069,#25070,
#25071,#25072,#25073,#25074,#25075,#25076,#25077,#25078,#25079,#25080,#25081,
#25082,#25083,#25084,#25085,#25086,#25087,#25088,#25089,#25090,#25091,#25092,
#25093,#25094,#25095,#25096,#25097,#25098,#25099,#25100,#25101,#25102,#25103,
#25104,#25105,#25106,#25107,#25108,#25109,#25110,#25111,#25112,#25113,#25114,
#25115,#25116,#25117,#25118,#25119,#25120,#25121,#25122,#25123,#25124,#25125,
#25126,#25127,#25128,#25129,#25130,#25131,#25132,#25133,#25134,#25135,#25136,
#25137,#25138,#25139,#25140,#25141,#25142,#25143,#25144,#25145,#25146,#25147,
#25148,#25149,#25150,#25151,#25152,#25153,#25154,#25155,#25156,#25157,#25158,
#25159,#25160,#25161,#25162,#25163,#25164,#25165,#25166,#25167,#25168,#25169,
#25170,#25171,#25172,#25173,#25174,#25175,#25176,#25177,#25178,#25179,#25180,
#25181,#25182,#25183,#25184,#25185,#25186,#25187,#25188,#25189,#25190,#25191,
#25192,#25193,#25194,#25195,#25196,#25197,#25198,#25199,#25200,#25201,#25202,
#25203,#25204,#25205,#25206,#25207,#25208,#25209,#25210,#25211,#25212,#25213,
#25214,#25215,#25216,#25217,#25218,#25219,#25220,#25221,#25222,#25223,#25224,
#25225,#25226,#25227,#25228,#25229,#25230,#25231,#25232,#25233,#25234,#25235,
#25236,#25237,#25238,#25239,#25240,#25241,#25242,#25243,#25244,#25245,#25246,
#25247,#25248,#25249,#25250,#25251,#25252,#25253,#25254,#25255),(#25256,
#25257,#25258,#25259,#25260,#25261,#25262,#25263,#25264,#25265,#25266,#25267,
#25268,#25269,#25270,#25271,#25272,#25273,#25274,#25275,#25276,#25277,#25278,
#25279,#25280,#25281,#25282,#25283,#25284,#25285,#25286,#25287,#25288,#25289,
#25290,#25291,#25292,#25293,#25294,#25295,#25296,#25297,#25298,#25299,#25300,
#25301,#25302,#25303,#25304,#25305,#25306,#25307,#25308,#25309,#25310,#25311,
#25312,#25313,#25314,#25315,#25316,#25317,#25318,#25319,#25320,#25321,#25322,
#25323,#25324,#25325,#25326,#25327,#25328,#25329,#25330,#25331,#25332,#25333,
#25334,#25335,#25336,#25337,#25338,#25339,#25340,#25341,#25342,#25343,#25344,
#25345,#25346,#25347,#25348,#25349,#25350,#25351,#25352,#25353,#25354,#25355,
#25356,#25357,#25358,#25359,#25360,#25361,#25362,#25363,#25364,#25365,#25366,
#25367,#25368,#25369,#25370,#25371,#25372,#25373,#25374,#25375,#25376,#25377,
#25378,#25379,#25380,#25381,#25382,#25383,#25384,#25385,#25386,#25387,#25388,
#25389,#25390,#25391,#25392,#25393,#25394,#25395,#25396,#25397,#25398,#25399,
#25400,#25401,#25402,#25403,#25404,#25405,#25406,#25407,#25408,#25409,#25410,
#25411,#25412,#25413,#25414,#25415,#25416,#25417,#25418,#25419,#25420,#25421,
#25422,#25423,#25424,#25425,#25426,#25427,#25428,#25429,#25430,#25431,#25432,
#25433,#25434,#25435,#25436,#25437,#25438,#25439,#25440,#25441,#25442,#25443,
#25444,#25445,#25446,#25447,#25448,#25449,#25450,#25451,#25452,#25453,#25454,
#25455,#25456,#25457,#25458,#25459,#25460,#25461,#25462,#25463,#25464,#25465,
#25466,#25467,#25468,#25469,#25470,#25471,#25472,#25473,#25474,#25475,#25476,
#25477,#25478,#25479,#25480)),.UNSPECIFIED.,.F.,.F.,.F.)
B_SPLINE_SURFACE_WITH_KNOTS((2,2),(3,2,2,2,2,2,2,2,2,2,2,2,2,2,2,2,2,2,
2,2,2,2,2,2,2,2,2,2,2,2,2,2,2,2,2,2,2,2,2,2,2,2,2,2,2,2,2,2,2,2,2,2,2,2,
2,2,2,2,2,2,2,2,2,2,2,2,2,2,2,2,2,2,2,2,2,2,2,2,2,2,2,2,2,2,2,2,2,2,2,2,
2,2,2,2,2,2,2,2,2,2,2,2,2,2,2,2,2,2,2,2,2,2,3),(0.,1.00000154805557),(0.,
0.00892857142857143,0.0178571428571429,0.0267857142857143,0.0357142857142857,
0.0446428571428571,0.0535714285714286,0.0625,0.0714285714285714,0.0803571428571429,
0.0892857142857143,0.0982142857142857,0.107142857142857,0.116071428571429,
0.125,0.133928571428571,0.142857142857143,0.151785714285714,0.160714285714286,
0.169642857142857,0.178571428571429,0.1875,0.196428571428571,0.205357142857143,
0.214285714285714,0.223214285714286,0.232142857142857,0.241071428571429,
0.25,0.258928571428571,0.267857142857143,0.276785714285714,0.285714285714286,
0.294642857142857,0.303571428571429,0.3125,0.321428571428571,0.330357142857143,
0.339285714285714,0.348214285714286,0.357142857142857,0.366071428571429,
0.375,0.383928571428571,0.392857142857143,0.401785714285714,0.410714285714286,
0.419642857142857,0.428571428571429,0.4375,0.446428571428571,0.455357142857143,
0.464285714285714,0.473214285714286,0.482142857142857,0.491071428571429,
0.5,0.508928571428571,0.517857142857143,0.526785714285714,0.535714285714286,
0.544642857142857,0.553571428571429,0.5625,0.571428571428571,0.580357142857143,
0.589285714285714,0.598214285714286,0.607142857142857,0.616071428571429,
0.625,0.633928571428571,0.642857142857143,0.651785714285714,0.660714285714286,
0.669642857142857,0.678571428571429,0.6875,0.696428571428571,0.705357142857143,
0.714285714285714,0.723214285714286,0.732142857142857,0.741071428571429,
0.75,0.758928571428571,0.767857142857143,0.776785714285714,0.785714285714286,
0.794642857142857,0.803571428571429,0.8125,0.821428571428571,0.830357142857143,
0.839285714285714,0.848214285714286,0.857142857142857,0.866071428571429,
0.875,0.883928571428571,0.892857142857143,0.901785714285714,0.910714285714286,
0.919642857142857,0.928571428571429,0.9375,0.946428571428571,0.955357142857143,
0.964285714285714,0.973214285714286,0.982142857142857,0.991071428571429,
1.),.UNSPECIFIED.)
GEOMETRIC_REPRESENTATION_ITEM()
RATIONAL_B_SPLINE_SURFACE(((1.,0.923879532511287,1.,0.923879532511287,1.,
0.923879532511287,1.,0.923879532511287,1.,0.923879532511287,1.,0.923879532511287,
1.,0.923879532511287,1.,0.923879532511287,1.,0.923879532511287,1.,0.923879532511287,
1.,0.923879532511287,1.,0.923879532511287,1.,0.923879532511287,1.,0.923879532511287,
1.,0.923879532511287,1.,0.923879532511287,1.,0.923879532511287,1.,0.923879532511287,
1.,0.923879532511287,1.,0.923879532511287,1.,0.923879532511287,1.,0.923879532511287,
1.,0.923879532511287,1.,0.923879532511287,1.,0.923879532511287,1.,0.923879532511287,
1.,0.923879532511287,1.,0.923879532511287,1.,0.923879532511287,1.,0.923879532511287,
1.,0.923879532511287,1.,0.923879532511287,1.,0.923879532511287,1.,0.923879532511287,
1.,0.923879532511287,1.,0.923879532511287,1.,0.923879532511287,1.,0.923879532511287,
1.,0.923879532511287,1.,0.923879532511287,1.,0.923879532511287,1.,0.923879532511287,
1.,0.923879532511287,1.,0.923879532511287,1.,0.923879532511287,1.,0.923879532511287,
1.,0.923879532511287,1.,0.923879532511287,1.,0.923879532511287,1.,0.923879532511287,
1.,0.923879532511287,1.,0.923879532511287,1.,0.923879532511287,1.,0.923879532511287,
1.,0.923879532511287,1.,0.923879532511287,1.,0.923879532511287,1.,0.923879532511287,
1.,0.923879532511287,1.,0.923879532511287,1.,0.923879532511287,1.,0.923879532511287,
1.,0.923879532511287,1.,0.923879532511287,1.,0.923879532511287,1.,0.923879532511287,
1.,0.923879532511287,1.,0.923879532511287,1.,0.923879532511287,1.,0.923879532511287,
1.,0.923879532511287,1.,0.923879532511287,1.,0.923879532511287,1.,0.923879532511287,
1.,0.923879532511287,1.,0.923879532511287,1.,0.923879532511287,1.,0.923879532511287,
1.,0.923879532511287,1.,0.923879532511287,1.,0.923879532511287,1.,0.923879532511287,
1.,0.923879532511287,1.,0.923879532511287,1.,0.923879532511287,1.,0.923879532511287,
1.,0.923879532511287,1.,0.923879532511287,1.,0.923879532511287,1.,0.923879532511287,
1.,0.923879532511287,1.,0.923879532511287,1.,0.923879532511287,1.,0.923879532511287,
1.,0.923879532511287,1.,0.923879532511287,1.,0.923879532511287,1.,0.923879532511287,
1.,0.923879532511287,1.,0.923879532511287,1.,0.923879532511287,1.,0.923879532511287,
1.,0.923879532511287,1.,0.923879532511287,1.,0.923879532511287,1.,0.923879532511287,
1.,0.923879532511287,1.,0.923879532511287,1.,0.923879532511287,1.,0.923879532511287,
1.,0.923879532511287,1.,0.923879532511287,1.),(1.,0.923879532511287,1.,
0.923879532511287,1.,0.923879532511287,1.,0.923879532511287,1.,0.923879532511287,
1.,0.923879532511287,1.,0.923879532511287,1.,0.923879532511287,1.,0.923879532511287,
1.,0.923879532511287,1.,0.923879532511287,1.,0.923879532511287,1.,0.923879532511287,
1.,0.923879532511287,1.,0.923879532511287,1.,0.923879532511287,1.,0.923879532511287,
1.,0.923879532511287,1.,0.923879532511287,1.,0.923879532511287,1.,0.923879532511287,
1.,0.923879532511287,1.,0.923879532511287,1.,0.923879532511287,1.,0.923879532511287,
1.,0.923879532511287,1.,0.923879532511287,1.,0.923879532511287,1.,0.923879532511287,
1.,0.923879532511287,1.,0.923879532511287,1.,0.923879532511287,1.,0.923879532511287,
1.,0.923879532511287,1.,0.923879532511287,1.,0.923879532511287,1.,0.923879532511287,
1.,0.923879532511287,1.,0.923879532511287,1.,0.923879532511287,1.,0.923879532511287,
1.,0.923879532511287,1.,0.923879532511287,1.,0.923879532511287,1.,0.923879532511287,
1.,0.923879532511287,1.,0.923879532511287,1.,0.923879532511287,1.,0.923879532511287,
1.,0.923879532511287,1.,0.923879532511287,1.,0.923879532511287,1.,0.923879532511287,
1.,0.923879532511287,1.,0.923879532511287,1.,0.923879532511287,1.,0.923879532511287,
1.,0.923879532511287,1.,0.923879532511287,1.,0.923879532511287,1.,0.923879532511287,
1.,0.923879532511287,1.,0.923879532511287,1.,0.923879532511287,1.,0.923879532511287,
1.,0.923879532511287,1.,0.923879532511287,1.,0.923879532511287,1.,0.923879532511287,
1.,0.923879532511287,1.,0.923879532511287,1.,0.923879532511287,1.,0.923879532511287,
1.,0.923879532511287,1.,0.923879532511287,1.,0.923879532511287,1.,0.923879532511287,
1.,0.923879532511287,1.,0.923879532511287,1.,0.923879532511287,1.,0.923879532511287,
1.,0.923879532511287,1.,0.923879532511287,1.,0.923879532511287,1.,0.923879532511287,
1.,0.923879532511287,1.,0.923879532511287,1.,0.923879532511287,1.,0.923879532511287,
1.,0.923879532511287,1.,0.923879532511287,1.,0.923879532511287,1.,0.923879532511287,
1.,0.923879532511287,1.,0.923879532511287,1.,0.923879532511287,1.,0.923879532511287,
1.,0.923879532511287,1.,0.923879532511287,1.,0.923879532511287,1.,0.923879532511287,
1.,0.923879532511287,1.,0.923879532511287,1.,0.923879532511287,1.,0.923879532511287,
1.,0.923879532511287,1.,0.923879532511287,1.,0.923879532511287,1.,0.923879532511287,
1.,0.923879532511287,1.,0.923879532511287,1.,0.923879532511287,1.)))
REPRESENTATION_ITEM('')
SURFACE()
);
#324=(
BOUNDED_SURFACE()
B_SPLINE_SURFACE(1,2,((#25500,#25501,#25502,#25503,#25504,#25505,#25506,
#25507,#25508,#25509,#25510,#25511,#25512,#25513,#25514,#25515,#25516,#25517,
#25518,#25519,#25520,#25521,#25522,#25523,#25524,#25525,#25526,#25527,#25528,
#25529,#25530,#25531,#25532,#25533,#25534,#25535,#25536,#25537,#25538,#25539,
#25540,#25541,#25542,#25543,#25544,#25545,#25546,#25547,#25548,#25549,#25550,
#25551,#25552,#25553,#25554,#25555,#25556,#25557,#25558,#25559,#25560,#25561,
#25562,#25563,#25564,#25565,#25566,#25567,#25568,#25569,#25570,#25571,#25572,
#25573,#25574,#25575,#25576,#25577,#25578,#25579,#25580,#25581,#25582,#25583,
#25584,#25585,#25586,#25587,#25588,#25589,#25590,#25591,#25592,#25593,#25594,
#25595,#25596,#25597,#25598,#25599,#25600,#25601,#25602,#25603,#25604,#25605,
#25606,#25607,#25608,#25609,#25610,#25611,#25612,#25613,#25614,#25615,#25616,
#25617,#25618,#25619,#25620,#25621,#25622,#25623,#25624,#25625,#25626,#25627,
#25628,#25629,#25630,#25631,#25632,#25633,#25634,#25635,#25636,#25637,#25638,
#25639,#25640,#25641,#25642,#25643,#25644,#25645,#25646,#25647,#25648,#25649,
#25650,#25651,#25652,#25653,#25654,#25655,#25656,#25657,#25658,#25659,#25660,
#25661,#25662,#25663,#25664,#25665,#25666,#25667,#25668,#25669,#25670,#25671,
#25672,#25673,#25674,#25675,#25676,#25677,#25678,#25679,#25680,#25681,#25682,
#25683,#25684,#25685,#25686,#25687,#25688,#25689,#25690,#25691,#25692,#25693,
#25694,#25695,#25696,#25697,#25698,#25699,#25700,#25701,#25702,#25703,#25704,
#25705,#25706,#25707,#25708,#25709,#25710,#25711,#25712,#25713,#25714,#25715,
#25716,#25717,#25718,#25719,#25720,#25721,#25722,#25723,#25724),(#25725,
#25726,#25727,#25728,#25729,#25730,#25731,#25732,#25733,#25734,#25735,#25736,
#25737,#25738,#25739,#25740,#25741,#25742,#25743,#25744,#25745,#25746,#25747,
#25748,#25749,#25750,#25751,#25752,#25753,#25754,#25755,#25756,#25757,#25758,
#25759,#25760,#25761,#25762,#25763,#25764,#25765,#25766,#25767,#25768,#25769,
#25770,#25771,#25772,#25773,#25774,#25775,#25776,#25777,#25778,#25779,#25780,
#25781,#25782,#25783,#25784,#25785,#25786,#25787,#25788,#25789,#25790,#25791,
#25792,#25793,#25794,#25795,#25796,#25797,#25798,#25799,#25800,#25801,#25802,
#25803,#25804,#25805,#25806,#25807,#25808,#25809,#25810,#25811,#25812,#25813,
#25814,#25815,#25816,#25817,#25818,#25819,#25820,#25821,#25822,#25823,#25824,
#25825,#25826,#25827,#25828,#25829,#25830,#25831,#25832,#25833,#25834,#25835,
#25836,#25837,#25838,#25839,#25840,#25841,#25842,#25843,#25844,#25845,#25846,
#25847,#25848,#25849,#25850,#25851,#25852,#25853,#25854,#25855,#25856,#25857,
#25858,#25859,#25860,#25861,#25862,#25863,#25864,#25865,#25866,#25867,#25868,
#25869,#25870,#25871,#25872,#25873,#25874,#25875,#25876,#25877,#25878,#25879,
#25880,#25881,#25882,#25883,#25884,#25885,#25886,#25887,#25888,#25889,#25890,
#25891,#25892,#25893,#25894,#25895,#25896,#25897,#25898,#25899,#25900,#25901,
#25902,#25903,#25904,#25905,#25906,#25907,#25908,#25909,#25910,#25911,#25912,
#25913,#25914,#25915,#25916,#25917,#25918,#25919,#25920,#25921,#25922,#25923,
#25924,#25925,#25926,#25927,#25928,#25929,#25930,#25931,#25932,#25933,#25934,
#25935,#25936,#25937,#25938,#25939,#25940,#25941,#25942,#25943,#25944,#25945,
#25946,#25947,#25948,#25949)),.UNSPECIFIED.,.F.,.F.,.F.)
B_SPLINE_SURFACE_WITH_KNOTS((2,2),(3,2,2,2,2,2,2,2,2,2,2,2,2,2,2,2,2,2,
2,2,2,2,2,2,2,2,2,2,2,2,2,2,2,2,2,2,2,2,2,2,2,2,2,2,2,2,2,2,2,2,2,2,2,2,
2,2,2,2,2,2,2,2,2,2,2,2,2,2,2,2,2,2,2,2,2,2,2,2,2,2,2,2,2,2,2,2,2,2,2,2,
2,2,2,2,2,2,2,2,2,2,2,2,2,2,2,2,2,2,2,2,2,2,3),(0.,1.),(0.,0.00892857142857143,
0.0178571428571429,0.0267857142857143,0.0357142857142857,0.0446428571428571,
0.0535714285714286,0.0625,0.0714285714285714,0.0803571428571429,0.0892857142857143,
0.0982142857142857,0.107142857142857,0.116071428571429,0.125,0.133928571428571,
0.142857142857143,0.151785714285714,0.160714285714286,0.169642857142857,
0.178571428571429,0.1875,0.196428571428571,0.205357142857143,0.214285714285714,
0.223214285714286,0.232142857142857,0.241071428571429,0.25,0.258928571428571,
0.267857142857143,0.276785714285714,0.285714285714286,0.294642857142857,
0.303571428571429,0.3125,0.321428571428571,0.330357142857143,0.339285714285714,
0.348214285714286,0.357142857142857,0.366071428571429,0.375,0.383928571428571,
0.392857142857143,0.401785714285714,0.410714285714286,0.419642857142857,
0.428571428571429,0.4375,0.446428571428571,0.455357142857143,0.464285714285714,
0.473214285714286,0.482142857142857,0.491071428571429,0.5,0.508928571428571,
0.517857142857143,0.526785714285714,0.535714285714286,0.544642857142857,
0.553571428571429,0.5625,0.571428571428571,0.580357142857143,0.589285714285714,
0.598214285714286,0.607142857142857,0.616071428571429,0.625,0.633928571428571,
0.642857142857143,0.651785714285714,0.660714285714286,0.669642857142857,
0.678571428571429,0.6875,0.696428571428571,0.705357142857143,0.714285714285714,
0.723214285714286,0.732142857142857,0.741071428571429,0.75,0.758928571428571,
0.767857142857143,0.776785714285714,0.785714285714286,0.794642857142857,
0.803571428571429,0.8125,0.821428571428571,0.830357142857143,0.839285714285714,
0.848214285714286,0.857142857142857,0.866071428571429,0.875,0.883928571428571,
0.892857142857143,0.901785714285714,0.910714285714286,0.919642857142857,
0.928571428571429,0.9375,0.946428571428571,0.955357142857143,0.964285714285714,
0.973214285714286,0.982142857142857,0.991071428571429,1.),.UNSPECIFIED.)
GEOMETRIC_REPRESENTATION_ITEM()
RATIONAL_B_SPLINE_SURFACE(((1.,0.923879532511287,1.,0.923879532511287,1.,
0.923879532511287,1.,0.923879532511287,1.,0.923879532511287,1.,0.923879532511287,
1.,0.923879532511287,1.,0.923879532511287,1.,0.923879532511287,1.,0.923879532511287,
1.,0.923879532511287,1.,0.923879532511287,1.,0.923879532511287,1.,0.923879532511287,
1.,0.923879532511287,1.,0.923879532511287,1.,0.923879532511287,1.,0.923879532511287,
1.,0.923879532511287,1.,0.923879532511287,1.,0.923879532511287,1.,0.923879532511287,
1.,0.923879532511287,1.,0.923879532511287,1.,0.923879532511287,1.,0.923879532511287,
1.,0.923879532511287,1.,0.923879532511287,1.,0.923879532511287,1.,0.923879532511287,
1.,0.923879532511287,1.,0.923879532511287,1.,0.923879532511287,1.,0.923879532511287,
1.,0.923879532511287,1.,0.923879532511287,1.,0.923879532511287,1.,0.923879532511287,
1.,0.923879532511287,1.,0.923879532511287,1.,0.923879532511287,1.,0.923879532511287,
1.,0.923879532511287,1.,0.923879532511287,1.,0.923879532511287,1.,0.923879532511287,
1.,0.923879532511287,1.,0.923879532511287,1.,0.923879532511287,1.,0.923879532511287,
1.,0.923879532511287,1.,0.923879532511287,1.,0.923879532511287,1.,0.923879532511287,
1.,0.923879532511287,1.,0.923879532511287,1.,0.923879532511287,1.,0.923879532511287,
1.,0.923879532511287,1.,0.923879532511287,1.,0.923879532511287,1.,0.923879532511287,
1.,0.923879532511287,1.,0.923879532511287,1.,0.923879532511287,1.,0.923879532511287,
1.,0.923879532511287,1.,0.923879532511287,1.,0.923879532511287,1.,0.923879532511287,
1.,0.923879532511287,1.,0.923879532511287,1.,0.923879532511287,1.,0.923879532511287,
1.,0.923879532511287,1.,0.923879532511287,1.,0.923879532511287,1.,0.923879532511287,
1.,0.923879532511287,1.,0.923879532511287,1.,0.923879532511287,1.,0.923879532511287,
1.,0.923879532511287,1.,0.923879532511287,1.,0.923879532511287,1.,0.923879532511287,
1.,0.923879532511287,1.,0.923879532511287,1.,0.923879532511287,1.,0.923879532511287,
1.,0.923879532511287,1.,0.923879532511287,1.,0.923879532511287,1.,0.923879532511287,
1.,0.923879532511287,1.,0.923879532511287,1.,0.923879532511287,1.,0.923879532511287,
1.,0.923879532511287,1.,0.923879532511287,1.,0.923879532511287,1.,0.923879532511287,
1.,0.923879532511287,1.,0.923879532511287,1.,0.923879532511287,1.,0.923879532511287,
1.,0.923879532511287,1.,0.923879532511287,1.,0.923879532511287,1.,0.923879532511287,
1.,0.923879532511287,1.,0.923879532511287,1.),(1.,0.923879532511287,1.,
0.923879532511287,1.,0.923879532511287,1.,0.923879532511287,1.,0.923879532511287,
1.,0.923879532511287,1.,0.923879532511287,1.,0.923879532511287,1.,0.923879532511287,
1.,0.923879532511287,1.,0.923879532511287,1.,0.923879532511287,1.,0.923879532511287,
1.,0.923879532511287,1.,0.923879532511287,1.,0.923879532511287,1.,0.923879532511287,
1.,0.923879532511287,1.,0.923879532511287,1.,0.923879532511287,1.,0.923879532511287,
1.,0.923879532511287,1.,0.923879532511287,1.,0.923879532511287,1.,0.923879532511287,
1.,0.923879532511287,1.,0.923879532511287,1.,0.923879532511287,1.,0.923879532511287,
1.,0.923879532511287,1.,0.923879532511287,1.,0.923879532511287,1.,0.923879532511287,
1.,0.923879532511287,1.,0.923879532511287,1.,0.923879532511287,1.,0.923879532511287,
1.,0.923879532511287,1.,0.923879532511287,1.,0.923879532511287,1.,0.923879532511287,
1.,0.923879532511287,1.,0.923879532511287,1.,0.923879532511287,1.,0.923879532511287,
1.,0.923879532511287,1.,0.923879532511287,1.,0.923879532511287,1.,0.923879532511287,
1.,0.923879532511287,1.,0.923879532511287,1.,0.923879532511287,1.,0.923879532511287,
1.,0.923879532511287,1.,0.923879532511287,1.,0.923879532511287,1.,0.923879532511287,
1.,0.923879532511287,1.,0.923879532511287,1.,0.923879532511287,1.,0.923879532511287,
1.,0.923879532511287,1.,0.923879532511287,1.,0.923879532511287,1.,0.923879532511287,
1.,0.923879532511287,1.,0.923879532511287,1.,0.923879532511287,1.,0.923879532511287,
1.,0.923879532511287,1.,0.923879532511287,1.,0.923879532511287,1.,0.923879532511287,
1.,0.923879532511287,1.,0.923879532511287,1.,0.923879532511287,1.,0.923879532511287,
1.,0.923879532511287,1.,0.923879532511287,1.,0.923879532511287,1.,0.923879532511287,
1.,0.923879532511287,1.,0.923879532511287,1.,0.923879532511287,1.,0.923879532511287,
1.,0.923879532511287,1.,0.923879532511287,1.,0.923879532511287,1.,0.923879532511287,
1.,0.923879532511287,1.,0.923879532511287,1.,0.923879532511287,1.,0.923879532511287,
1.,0.923879532511287,1.,0.923879532511287,1.,0.923879532511287,1.,0.923879532511287,
1.,0.923879532511287,1.,0.923879532511287,1.,0.923879532511287,1.,0.923879532511287,
1.,0.923879532511287,1.,0.923879532511287,1.,0.923879532511287,1.,0.923879532511287,
1.,0.923879532511287,1.,0.923879532511287,1.,0.923879532511287,1.,0.923879532511287,
1.,0.923879532511287,1.,0.923879532511287,1.,0.923879532511287,1.)))
REPRESENTATION_ITEM('')
SURFACE()
);
#325=(
BOUNDED_SURFACE()
B_SPLINE_SURFACE(1,2,((#27042,#27043,#27044,#27045,#27046,#27047,#27048,
#27049,#27050,#27051,#27052,#27053,#27054,#27055,#27056,#27057,#27058,#27059,
#27060,#27061,#27062,#27063,#27064,#27065,#27066,#27067,#27068,#27069,#27070,
#27071,#27072,#27073,#27074,#27075,#27076,#27077,#27078,#27079,#27080,#27081,
#27082,#27083,#27084,#27085,#27086,#27087,#27088,#27089,#27090,#27091,#27092,
#27093,#27094,#27095,#27096,#27097,#27098,#27099,#27100,#27101,#27102,#27103,
#27104,#27105,#27106,#27107,#27108,#27109,#27110,#27111,#27112,#27113,#27114,
#27115,#27116,#27117,#27118,#27119,#27120,#27121,#27122,#27123,#27124,#27125,
#27126,#27127,#27128,#27129,#27130,#27131,#27132,#27133,#27134,#27135,#27136,
#27137,#27138,#27139,#27140,#27141,#27142,#27143,#27144,#27145,#27146,#27147,
#27148,#27149,#27150,#27151,#27152,#27153,#27154,#27155,#27156,#27157,#27158,
#27159,#27160,#27161,#27162,#27163,#27164,#27165,#27166,#27167,#27168,#27169,
#27170,#27171,#27172,#27173,#27174,#27175,#27176,#27177,#27178,#27179,#27180,
#27181,#27182,#27183,#27184,#27185,#27186,#27187,#27188,#27189,#27190,#27191,
#27192,#27193,#27194,#27195,#27196,#27197,#27198,#27199,#27200,#27201,#27202),
(#27203,#27204,#27205,#27206,#27207,#27208,#27209,#27210,#27211,#27212,
#27213,#27214,#27215,#27216,#27217,#27218,#27219,#27220,#27221,#27222,#27223,
#27224,#27225,#27226,#27227,#27228,#27229,#27230,#27231,#27232,#27233,#27234,
#27235,#27236,#27237,#27238,#27239,#27240,#27241,#27242,#27243,#27244,#27245,
#27246,#27247,#27248,#27249,#27250,#27251,#27252,#27253,#27254,#27255,#27256,
#27257,#27258,#27259,#27260,#27261,#27262,#27263,#27264,#27265,#27266,#27267,
#27268,#27269,#27270,#27271,#27272,#27273,#27274,#27275,#27276,#27277,#27278,
#27279,#27280,#27281,#27282,#27283,#27284,#27285,#27286,#27287,#27288,#27289,
#27290,#27291,#27292,#27293,#27294,#27295,#27296,#27297,#27298,#27299,#27300,
#27301,#27302,#27303,#27304,#27305,#27306,#27307,#27308,#27309,#27310,#27311,
#27312,#27313,#27314,#27315,#27316,#27317,#27318,#27319,#27320,#27321,#27322,
#27323,#27324,#27325,#27326,#27327,#27328,#27329,#27330,#27331,#27332,#27333,
#27334,#27335,#27336,#27337,#27338,#27339,#27340,#27341,#27342,#27343,#27344,
#27345,#27346,#27347,#27348,#27349,#27350,#27351,#27352,#27353,#27354,#27355,
#27356,#27357,#27358,#27359,#27360,#27361,#27362,#27363)),.UNSPECIFIED.,
 .F.,.F.,.F.)
B_SPLINE_SURFACE_WITH_KNOTS((2,2),(3,2,2,2,2,2,2,2,2,2,2,2,2,2,2,2,2,2,
2,2,2,2,2,2,2,2,2,2,2,2,2,2,2,2,2,2,2,2,2,2,2,2,2,2,2,2,2,2,2,2,2,2,2,2,
2,2,2,2,2,2,2,2,2,2,2,2,2,2,2,2,2,2,2,2,2,2,2,2,2,2,3),(0.,1.),(0.,0.0125,
0.025,0.0375,0.05,0.0625,0.075,0.0875,0.1,0.1125,0.125,0.1375,0.15,0.1625,
0.175,0.1875,0.2,0.2125,0.225,0.2375,0.25,0.2625,0.275,0.2875,0.3,0.3125,
0.325,0.3375,0.35,0.3625,0.375,0.3875,0.4,0.4125,0.425,0.4375,0.45,0.4625,
0.475,0.4875,0.5,0.5125,0.525,0.5375,0.55,0.5625,0.575,0.5875,0.6,0.6125,
0.625,0.6375,0.65,0.6625,0.675,0.6875,0.7,0.7125,0.725,0.7375,0.75,0.7625,
0.775,0.7875,0.8,0.8125,0.825,0.8375,0.85,0.8625,0.875,0.8875,0.9,0.9125,
0.925,0.9375,0.95,0.9625,0.975,0.9875,1.),.UNSPECIFIED.)
GEOMETRIC_REPRESENTATION_ITEM()
RATIONAL_B_SPLINE_SURFACE(((1.,0.923879532511287,1.,0.923879532511287,1.,
0.923879532511287,1.,0.923879532511287,1.,0.923879532511287,1.,0.923879532511287,
1.,0.923879532511287,1.,0.923879532511287,1.,0.923879532511287,1.,0.923879532511287,
1.,0.923879532511287,1.,0.923879532511287,1.,0.923879532511287,1.,0.923879532511287,
1.,0.923879532511287,1.,0.923879532511287,1.,0.923879532511287,1.,0.923879532511287,
1.,0.923879532511287,1.,0.923879532511287,1.,0.923879532511287,1.,0.923879532511287,
1.,0.923879532511287,1.,0.923879532511287,1.,0.923879532511287,1.,0.923879532511287,
1.,0.923879532511287,1.,0.923879532511287,1.,0.923879532511287,1.,0.923879532511287,
1.,0.923879532511287,1.,0.923879532511287,1.,0.923879532511287,1.,0.923879532511287,
1.,0.923879532511287,1.,0.923879532511287,1.,0.923879532511287,1.,0.923879532511287,
1.,0.923879532511287,1.,0.923879532511287,1.,0.923879532511287,1.,0.923879532511287,
1.,0.923879532511287,1.,0.923879532511287,1.,0.923879532511287,1.,0.923879532511287,
1.,0.923879532511287,1.,0.923879532511287,1.,0.923879532511287,1.,0.923879532511287,
1.,0.923879532511287,1.,0.923879532511287,1.,0.923879532511287,1.,0.923879532511287,
1.,0.923879532511287,1.,0.923879532511287,1.,0.923879532511287,1.,0.923879532511287,
1.,0.923879532511287,1.,0.923879532511287,1.,0.923879532511287,1.,0.923879532511287,
1.,0.923879532511287,1.,0.923879532511287,1.,0.923879532511287,1.,0.923879532511287,
1.,0.923879532511287,1.,0.923879532511287,1.,0.923879532511287,1.,0.923879532511287,
1.,0.923879532511287,1.,0.923879532511287,1.,0.923879532511287,1.,0.923879532511287,
1.,0.923879532511287,1.,0.923879532511287,1.,0.923879532511287,1.,0.923879532511287,
1.,0.923879532511287,1.,0.923879532511287,1.),(1.,0.923879532511287,1.,
0.923879532511287,1.,0.923879532511287,1.,0.923879532511287,1.,0.923879532511287,
1.,0.923879532511287,1.,0.923879532511287,1.,0.923879532511287,1.,0.923879532511287,
1.,0.923879532511287,1.,0.923879532511287,1.,0.923879532511287,1.,0.923879532511287,
1.,0.923879532511287,1.,0.923879532511287,1.,0.923879532511287,1.,0.923879532511287,
1.,0.923879532511287,1.,0.923879532511287,1.,0.923879532511287,1.,0.923879532511287,
1.,0.923879532511287,1.,0.923879532511287,1.,0.923879532511287,1.,0.923879532511287,
1.,0.923879532511287,1.,0.923879532511287,1.,0.923879532511287,1.,0.923879532511287,
1.,0.923879532511287,1.,0.923879532511287,1.,0.923879532511287,1.,0.923879532511287,
1.,0.923879532511287,1.,0.923879532511287,1.,0.923879532511287,1.,0.923879532511287,
1.,0.923879532511287,1.,0.923879532511287,1.,0.923879532511287,1.,0.923879532511287,
1.,0.923879532511287,1.,0.923879532511287,1.,0.923879532511287,1.,0.923879532511287,
1.,0.923879532511287,1.,0.923879532511287,1.,0.923879532511287,1.,0.923879532511287,
1.,0.923879532511287,1.,0.923879532511287,1.,0.923879532511287,1.,0.923879532511287,
1.,0.923879532511287,1.,0.923879532511287,1.,0.923879532511287,1.,0.923879532511287,
1.,0.923879532511287,1.,0.923879532511287,1.,0.923879532511287,1.,0.923879532511287,
1.,0.923879532511287,1.,0.923879532511287,1.,0.923879532511287,1.,0.923879532511287,
1.,0.923879532511287,1.,0.923879532511287,1.,0.923879532511287,1.,0.923879532511287,
1.,0.923879532511287,1.,0.923879532511287,1.,0.923879532511287,1.,0.923879532511287,
1.,0.923879532511287,1.,0.923879532511287,1.,0.923879532511287,1.,0.923879532511287,
1.,0.923879532511287,1.,0.923879532511287,1.,0.923879532511287,1.)))
REPRESENTATION_ITEM('')
SURFACE()
);
#326=(
BOUNDED_SURFACE()
B_SPLINE_SURFACE(1,2,((#27364,#27365,#27366,#27367,#27368,#27369,#27370,
#27371,#27372,#27373,#27374,#27375,#27376,#27377,#27378,#27379,#27380,#27381,
#27382,#27383,#27384,#27385,#27386,#27387,#27388,#27389,#27390,#27391,#27392,
#27393,#27394,#27395,#27396,#27397,#27398,#27399,#27400,#27401,#27402,#27403,
#27404,#27405,#27406,#27407,#27408,#27409,#27410,#27411,#27412,#27413,#27414,
#27415,#27416,#27417,#27418,#27419,#27420,#27421,#27422,#27423,#27424,#27425,
#27426,#27427,#27428,#27429,#27430,#27431,#27432,#27433,#27434,#27435,#27436,
#27437,#27438,#27439,#27440,#27441,#27442,#27443,#27444,#27445,#27446,#27447,
#27448,#27449,#27450,#27451,#27452,#27453,#27454,#27455,#27456,#27457,#27458,
#27459,#27460,#27461,#27462,#27463,#27464,#27465,#27466,#27467,#27468,#27469,
#27470,#27471,#27472,#27473,#27474,#27475,#27476,#27477,#27478,#27479,#27480,
#27481,#27482,#27483,#27484,#27485,#27486,#27487,#27488,#27489,#27490,#27491,
#27492,#27493,#27494,#27495,#27496,#27497,#27498,#27499,#27500,#27501,#27502,
#27503,#27504,#27505,#27506,#27507,#27508,#27509,#27510,#27511,#27512,#27513,
#27514,#27515,#27516,#27517,#27518,#27519,#27520,#27521,#27522,#27523,#27524),
(#27525,#27526,#27527,#27528,#27529,#27530,#27531,#27532,#27533,#27534,
#27535,#27536,#27537,#27538,#27539,#27540,#27541,#27542,#27543,#27544,#27545,
#27546,#27547,#27548,#27549,#27550,#27551,#27552,#27553,#27554,#27555,#27556,
#27557,#27558,#27559,#27560,#27561,#27562,#27563,#27564,#27565,#27566,#27567,
#27568,#27569,#27570,#27571,#27572,#27573,#27574,#27575,#27576,#27577,#27578,
#27579,#27580,#27581,#27582,#27583,#27584,#27585,#27586,#27587,#27588,#27589,
#27590,#27591,#27592,#27593,#27594,#27595,#27596,#27597,#27598,#27599,#27600,
#27601,#27602,#27603,#27604,#27605,#27606,#27607,#27608,#27609,#27610,#27611,
#27612,#27613,#27614,#27615,#27616,#27617,#27618,#27619,#27620,#27621,#27622,
#27623,#27624,#27625,#27626,#27627,#27628,#27629,#27630,#27631,#27632,#27633,
#27634,#27635,#27636,#27637,#27638,#27639,#27640,#27641,#27642,#27643,#27644,
#27645,#27646,#27647,#27648,#27649,#27650,#27651,#27652,#27653,#27654,#27655,
#27656,#27657,#27658,#27659,#27660,#27661,#27662,#27663,#27664,#27665,#27666,
#27667,#27668,#27669,#27670,#27671,#27672,#27673,#27674,#27675,#27676,#27677,
#27678,#27679,#27680,#27681,#27682,#27683,#27684,#27685)),.UNSPECIFIED.,
 .F.,.F.,.F.)
B_SPLINE_SURFACE_WITH_KNOTS((2,2),(3,2,2,2,2,2,2,2,2,2,2,2,2,2,2,2,2,2,
2,2,2,2,2,2,2,2,2,2,2,2,2,2,2,2,2,2,2,2,2,2,2,2,2,2,2,2,2,2,2,2,2,2,2,2,
2,2,2,2,2,2,2,2,2,2,2,2,2,2,2,2,2,2,2,2,2,2,2,2,2,2,3),(0.,1.),(0.,0.0125,
0.025,0.0375,0.05,0.0625,0.075,0.0875,0.1,0.1125,0.125,0.1375,0.15,0.1625,
0.175,0.1875,0.2,0.2125,0.225,0.2375,0.25,0.2625,0.275,0.2875,0.3,0.3125,
0.325,0.3375,0.35,0.3625,0.375,0.3875,0.4,0.4125,0.425,0.4375,0.45,0.4625,
0.475,0.4875,0.5,0.5125,0.525,0.5375,0.55,0.5625,0.575,0.5875,0.6,0.6125,
0.625,0.6375,0.65,0.6625,0.675,0.6875,0.7,0.7125,0.725,0.7375,0.75,0.7625,
0.775,0.7875,0.8,0.8125,0.825,0.8375,0.85,0.8625,0.875,0.8875,0.9,0.9125,
0.925,0.9375,0.95,0.9625,0.975,0.9875,1.),.UNSPECIFIED.)
GEOMETRIC_REPRESENTATION_ITEM()
RATIONAL_B_SPLINE_SURFACE(((1.,0.923879532511287,1.,0.923879532511287,1.,
0.923879532511287,1.,0.923879532511287,1.,0.923879532511287,1.,0.923879532511287,
1.,0.923879532511287,1.,0.923879532511287,1.,0.923879532511287,1.,0.923879532511287,
1.,0.923879532511287,1.,0.923879532511287,1.,0.923879532511287,1.,0.923879532511287,
1.,0.923879532511287,1.,0.923879532511287,1.,0.923879532511287,1.,0.923879532511287,
1.,0.923879532511287,1.,0.923879532511287,1.,0.923879532511287,1.,0.923879532511287,
1.,0.923879532511287,1.,0.923879532511287,1.,0.923879532511287,1.,0.923879532511287,
1.,0.923879532511287,1.,0.923879532511287,1.,0.923879532511287,1.,0.923879532511287,
1.,0.923879532511287,1.,0.923879532511287,1.,0.923879532511287,1.,0.923879532511287,
1.,0.923879532511287,1.,0.923879532511287,1.,0.923879532511287,1.,0.923879532511287,
1.,0.923879532511287,1.,0.923879532511287,1.,0.923879532511287,1.,0.923879532511287,
1.,0.923879532511287,1.,0.923879532511287,1.,0.923879532511287,1.,0.923879532511287,
1.,0.923879532511287,1.,0.923879532511287,1.,0.923879532511287,1.,0.923879532511287,
1.,0.923879532511287,1.,0.923879532511287,1.,0.923879532511287,1.,0.923879532511287,
1.,0.923879532511287,1.,0.923879532511287,1.,0.923879532511287,1.,0.923879532511287,
1.,0.923879532511287,1.,0.923879532511287,1.,0.923879532511287,1.,0.923879532511287,
1.,0.923879532511287,1.,0.923879532511287,1.,0.923879532511287,1.,0.923879532511287,
1.,0.923879532511287,1.,0.923879532511287,1.,0.923879532511287,1.,0.923879532511287,
1.,0.923879532511287,1.,0.923879532511287,1.,0.923879532511287,1.,0.923879532511287,
1.,0.923879532511287,1.,0.923879532511287,1.,0.923879532511287,1.,0.923879532511287,
1.,0.923879532511287,1.,0.923879532511287,1.),(1.,0.923879532511287,1.,
0.923879532511287,1.,0.923879532511287,1.,0.923879532511287,1.,0.923879532511287,
1.,0.923879532511287,1.,0.923879532511287,1.,0.923879532511287,1.,0.923879532511287,
1.,0.923879532511287,1.,0.923879532511287,1.,0.923879532511287,1.,0.923879532511287,
1.,0.923879532511287,1.,0.923879532511287,1.,0.923879532511287,1.,0.923879532511287,
1.,0.923879532511287,1.,0.923879532511287,1.,0.923879532511287,1.,0.923879532511287,
1.,0.923879532511287,1.,0.923879532511287,1.,0.923879532511287,1.,0.923879532511287,
1.,0.923879532511287,1.,0.923879532511287,1.,0.923879532511287,1.,0.923879532511287,
1.,0.923879532511287,1.,0.923879532511287,1.,0.923879532511287,1.,0.923879532511287,
1.,0.923879532511287,1.,0.923879532511287,1.,0.923879532511287,1.,0.923879532511287,
1.,0.923879532511287,1.,0.923879532511287,1.,0.923879532511287,1.,0.923879532511287,
1.,0.923879532511287,1.,0.923879532511287,1.,0.923879532511287,1.,0.923879532511287,
1.,0.923879532511287,1.,0.923879532511287,1.,0.923879532511287,1.,0.923879532511287,
1.,0.923879532511287,1.,0.923879532511287,1.,0.923879532511287,1.,0.923879532511287,
1.,0.923879532511287,1.,0.923879532511287,1.,0.923879532511287,1.,0.923879532511287,
1.,0.923879532511287,1.,0.923879532511287,1.,0.923879532511287,1.,0.923879532511287,
1.,0.923879532511287,1.,0.923879532511287,1.,0.923879532511287,1.,0.923879532511287,
1.,0.923879532511287,1.,0.923879532511287,1.,0.923879532511287,1.,0.923879532511287,
1.,0.923879532511287,1.,0.923879532511287,1.,0.923879532511287,1.,0.923879532511287,
1.,0.923879532511287,1.,0.923879532511287,1.,0.923879532511287,1.,0.923879532511287,
1.,0.923879532511287,1.,0.923879532511287,1.,0.923879532511287,1.)))
REPRESENTATION_ITEM('')
SURFACE()
);
#433=FACE_BOUND('',#2624,.T.);
#434=FACE_BOUND('',#2626,.T.);
#435=FACE_BOUND('',#2628,.T.);
#436=FACE_BOUND('',#2630,.T.);
#437=FACE_BOUND('',#2632,.T.);
#438=FACE_BOUND('',#2634,.T.);
#439=FACE_BOUND('',#2673,.T.);
#440=FACE_BOUND('',#2675,.T.);
#441=FACE_BOUND('',#2678,.T.);
#442=FACE_BOUND('',#2680,.T.);
#443=FACE_BOUND('',#2691,.T.);
#444=FACE_BOUND('',#2720,.T.);
#445=FACE_BOUND('',#2722,.T.);
#446=FACE_BOUND('',#2724,.T.);
#701=PLANE('',#13554);
#702=PLANE('',#13555);
#703=PLANE('',#13556);
#704=PLANE('',#13557);
#705=PLANE('',#13558);
#706=PLANE('',#13559);
#707=PLANE('',#13568);
#708=PLANE('',#13569);
#709=PLANE('',#13613);
#710=PLANE('',#13614);
#711=PLANE('',#13615);
#712=PLANE('',#13617);
#713=PLANE('',#13619);
#714=PLANE('',#13620);
#715=PLANE('',#13622);
#716=PLANE('',#13624);
#717=PLANE('',#13625);
#718=PLANE('',#13628);
#719=PLANE('',#13631);
#720=PLANE('',#13634);
#721=PLANE('',#13639);
#722=PLANE('',#13642);
#723=PLANE('',#13645);
#724=PLANE('',#13646);
#725=PLANE('',#13647);
#726=PLANE('',#13676);
#727=PLANE('',#13677);
#728=PLANE('',#13678);
#729=PLANE('',#13679);
#730=PLANE('',#13680);
#731=PLANE('',#13681);
#732=PLANE('',#13682);
#733=PLANE('',#13683);
#734=PLANE('',#13684);
#735=PLANE('',#13685);
#736=PLANE('',#13687);
#737=PLANE('',#13688);
#738=PLANE('',#13689);
#739=PLANE('',#13690);
#740=PLANE('',#13691);
#741=PLANE('',#13692);
#803=ELLIPSE('',#13632,5.35545030114693,4.99999999989344);
#804=ELLIPSE('',#13633,2.14218012048347,1.99999999999931);
#805=ELLIPSE('',#13635,5.00338652687943,4.99999999999998);
#806=ELLIPSE('',#13636,2.00135461075165,1.99999999999923);
#807=ELLIPSE('',#13640,5.00338652687943,4.99999999999998);
#808=ELLIPSE('',#13641,2.0013546107478,1.99999999999585);
#809=ELLIPSE('',#13643,5.3554503002225,4.99999999823902);
#810=ELLIPSE('',#13644,2.14218012048814,2.00000000000341);
#846=TOROIDAL_SURFACE('',#13523,23.,2.);
#847=TOROIDAL_SURFACE('',#13528,18.,2.);
#848=TOROIDAL_SURFACE('',#13532,23.,2.);
#849=TOROIDAL_SURFACE('',#13537,18.,2.);
#924=B_SPLINE_CURVE_WITH_KNOTS('',3,(#23891,#23892,#23893,#23894,#23895,
#23896,#23897,#23898,#23899,#23900,#23901,#23902,#23903,#23904,#23905,#23906,
#23907,#23908,#23909,#23910,#23911,#23912,#23913,#23914,#23915,#23916,#23917,
#23918,#23919,#23920,#23921,#23922,#23923,#23924,#23925,#23926),
 .UNSPECIFIED.,.F.,.F.,(4,2,2,2,2,2,2,2,2,2,2,2,2,2,2,2,2,4),(-5.52282176378171,
-5.32896740108138,-5.13535365951528,-4.93516142497304,-4.74154376120979,
-4.5415111268812,-4.34788553839797,-4.14801905426253,-3.95438131120499,
-3.75468774664587,-3.56103338796945,-3.36151970744337,-3.16784403857256,
-2.96851737109845,-2.77481546338195,-2.57568306526669,-2.38194975752097,
-2.3652150082907),.UNSPECIFIED.);
#925=B_SPLINE_CURVE_WITH_KNOTS('',3,(#23931,#23932,#23933,#23934,#23935,
#23936,#23937,#23938,#23939,#23940,#23941,#23942,#23943,#23944,#23945,#23946,
#23947,#23948,#23949,#23950,#23951,#23952,#23953,#23954,#23955,#23956,#23957,
#23958),.UNSPECIFIED.,.F.,.F.,(4,2,2,2,2,2,2,2,2,2,2,2,2,4),(-2.3652150082907,
-2.18301896778156,-1.98924887022321,-1.79052705823713,-1.59671455911293,
-1.39820906413684,-1.20434833935788,-1.00606640169784,-0.812151427768874,
-0.614100111573574,-0.420124682089828,-0.222310789965957,-0.110086721669281,
0.),.UNSPECIFIED.);
#926=B_SPLINE_CURVE_WITH_KNOTS('',3,(#23961,#23962,#23963,#23964,#23965,
#23966,#23967,#23968,#23969,#23970,#23971,#23972,#23973,#23974,#23975,#23976,
#23977,#23978,#23979,#23980,#23981,#23982,#23983,#23984,#23985,#23986,#23987,
#23988),.UNSPECIFIED.,.F.,.F.,(4,2,2,2,2,2,2,2,2,2,2,2,2,4),(-37.8682594959783,
-37.6786133520927,-37.4884259218183,-37.2957524665574,-37.0955311656665,
-36.9029287229397,-36.7028085078848,-36.5102760181044,-36.3102600197474,
-36.1177960120006,-35.9178874964689,-35.7254900298269,-35.5256923919229,
-35.5016722138548),.UNSPECIFIED.);
#927=B_SPLINE_CURVE_WITH_KNOTS('',3,(#23993,#23994,#23995,#23996,#23997,
#23998,#23999,#24000,#24001,#24002,#24003,#24004,#24005,#24006,#24007,#24008,
#24009,#24010,#24011,#24012,#24013,#24014,#24015,#24016,#24017,#24018,#24019,
#24020,#24021,#24022,#24023,#24024,#24025,#24026,#24027,#24028),
 .UNSPECIFIED.,.F.,.F.,(4,2,2,2,2,2,2,2,2,2,2,2,2,2,2,2,2,4),(-8.68543777224221,
-8.48472687974919,-8.29102562860789,-8.08976190515885,-7.89608135036397,
-7.69493407611858,-7.50127178683154,-7.30024542791767,-7.10659880541962,
-6.90569808926309,-6.71206435832943,-6.51129427837733,-6.31767047872643,
-6.11703629724468,-5.92341927516968,-5.72292652370587,-5.52931292401888,
-5.52282176378171),.UNSPECIFIED.);
#928=B_SPLINE_CURVE_WITH_KNOTS('',3,(#24029,#24030,#24031,#24032,#24033,
#24034,#24035,#24036,#24037,#24038,#24039,#24040,#24041,#24042,#24043,#24044,
#24045,#24046,#24047,#24048,#24049,#24050,#24051,#24052,#24053,#24054,#24055,
#24056,#24057,#24058,#24059,#24060,#24061,#24062,#24063,#24064),
 .UNSPECIFIED.,.F.,.F.,(4,2,2,2,2,2,2,2,2,2,2,2,2,2,2,2,2,4),(-35.5016722138548,
-35.3333589938397,-35.1336757480503,-34.9414033507716,-34.74183811963,-34.5496229958028,
-34.3501794953646,-34.1580171943271,-33.958699216547,-33.7665845030627,
-33.5673958948966,-33.3753226923794,-33.1762673314815,-32.9842286719963,
-32.7853104389487,-32.5932984224679,-32.3945211695547,-32.3486283723407),
 .UNSPECIFIED.);
#929=B_SPLINE_CURVE_WITH_KNOTS('',3,(#24069,#24070,#24071,#24072,#24073,
#24074,#24075,#24076,#24077,#24078,#24079,#24080,#24081,#24082,#24083,#24084,
#24085,#24086,#24087,#24088,#24089,#24090,#24091,#24092,#24093,#24094,#24095,
#24096,#24097,#24098,#24099,#24100,#24101,#24102,#24103,#24104,#24105,#24106),
 .UNSPECIFIED.,.F.,.F.,(4,2,2,2,2,2,2,2,2,2,2,2,2,2,2,2,2,2,4),(-11.8499565270215,
-11.8453602865149,-11.6442887880003,-11.4509185840308,-11.2497702173852,
-11.0563312257612,-10.8551076078354,-10.6616005804636,-10.4603032196308,
-10.2667289211856,-10.0653592228549,-9.87171842016381,-9.6702776922814,
-9.47657114566235,-9.27506060415086,-9.08131129636344,-8.87982706034636,
-8.68610284128992,-8.68543777224221),.UNSPECIFIED.);
#930=B_SPLINE_CURVE_WITH_KNOTS('',3,(#24107,#24108,#24109,#24110,#24111,
#24112,#24113,#24114,#24115,#24116,#24117,#24118,#24119,#24120,#24121,#24122,
#24123,#24124,#24125,#24126,#24127,#24128,#24129,#24130,#24131,#24132,#24133,
#24134,#24135,#24136,#24137,#24138,#24139,#24140,#24141,#24142),
 .UNSPECIFIED.,.F.,.F.,(4,2,2,2,2,2,2,2,2,2,2,2,2,2,2,2,2,4),(-32.3486283723407,
-32.2025269350576,-32.003894451693,-31.8119081627106,-31.6134241377314,
-31.4214349848199,-31.2231029659801,-31.0310991883577,-30.8329225394816,
-30.6408914676505,-30.4428733240406,-30.2508014446613,-30.0529446674791,
-29.8608177110558,-29.6631248415205,-29.4709278926409,-29.2734011069936,
-29.1971185456898),.UNSPECIFIED.);
#931=B_SPLINE_CURVE_WITH_KNOTS('',3,(#24147,#24148,#24149,#24150,#24151,
#24152,#24153,#24154,#24155,#24156,#24157,#24158,#24159,#24160,#24161,#24162,
#24163,#24164,#24165,#24166,#24167,#24168,#24169,#24170,#24171,#24172,#24173,
#24174,#24175,#24176,#24177,#24178,#24179,#24180,#24181,#24182),
 .UNSPECIFIED.,.F.,.F.,(4,2,2,2,2,2,2,2,2,2,2,2,2,2,2,2,2,4),(-15.009441259603,
-14.9953430620414,-14.7949594260182,-14.6021595264654,-14.4016815810857,
-14.2088094808993,-14.0082398828457,-13.8152955212959,-13.6146367850036,
-13.4216203037066,-13.2208748034208,-13.0277865097912,-12.8269564825509,
-12.633796817441,-12.4328843668124,-12.2396538761215,-12.0386609765248,
-11.8499565270215),.UNSPECIFIED.);
#932=B_SPLINE_CURVE_WITH_KNOTS('',3,(#24183,#24184,#24185,#24186,#24187,
#24188,#24189,#24190,#24191,#24192,#24193,#24194,#24195,#24196,#24197,#24198,
#24199,#24200,#24201,#24202,#24203,#24204,#24205,#24206,#24207,#24208,#24209,
#24210,#24211,#24212,#24213,#24214,#24215,#24216,#24217,#24218),
 .UNSPECIFIED.,.F.,.F.,(4,2,2,2,2,2,2,2,2,2,2,2,2,2,2,2,2,4),(-29.1971185456898,
-29.0811187359594,-28.883759802215,-28.6913762159564,-28.4941864535241,
-28.301685662787,-28.1046659060324,-27.9120319049695,-27.7151824717669,
-27.5223994253904,-27.3257200916267,-27.1327724566436,-26.9362624291837,
-26.7431351555522,-26.5467930764249,-26.3534719618308,-26.1572958989704,
-26.0460294638091),.UNSPECIFIED.);
#933=B_SPLINE_CURVE_WITH_KNOTS('',3,(#24223,#24224,#24225,#24226,#24227,
#24228,#24229,#24230,#24231,#24232,#24233,#24234,#24235,#24236,#24237,#24238,
#24239,#24240,#24241,#24242,#24243,#24244,#24245,#24246,#24247,#24248,#24249,
#24250,#24251,#24252,#24253,#24254,#24255,#24256,#24257,#24258),
 .UNSPECIFIED.,.F.,.F.,(4,2,2,2,2,2,2,2,2,2,2,2,2,2,2,2,2,4),(-18.1648534816952,
-18.1345623064237,-17.9350454383078,-17.7427812309514,-17.5431439069863,
-17.3508210506561,-17.1510669569855,-16.9586819589623,-16.7588146828344,
-16.5663646878438,-16.3663877041066,-16.1738704300427,-15.9737870904475,
-15.7812007653394,-15.5810142904072,-15.3883575917231,-15.1880710649215,
-15.009441259603),.UNSPECIFIED.);
#934=B_SPLINE_CURVE_WITH_KNOTS('',3,(#24259,#24260,#24261,#24262,#24263,
#24264,#24265,#24266,#24267,#24268,#24269,#24270,#24271,#24272,#24273,#24274,
#24275,#24276,#24277,#24278,#24279,#24280,#24281,#24282,#24283,#24284,#24285,
#24286,#24287,#24288,#24289,#24290,#24291,#24292,#24293,#24294),
 .UNSPECIFIED.,.F.,.F.,(4,2,2,2,2,2,2,2,2,2,2,2,2,2,2,2,2,4),(-26.0460294638091,
-25.9637676321335,-25.7677550828262,-25.5740073934036,-25.3781552970517,
-25.1841770843524,-24.9884818430204,-24.7942632805341,-24.5987207867594,
-24.4042534004878,-24.2088590716305,-24.0141357912462,-23.8188846094804,
-23.6238997923439,-23.4287863492596,-23.2335357782769,-23.0385543229855,
-22.894653858858),.UNSPECIFIED.);
#935=B_SPLINE_CURVE_WITH_KNOTS('',3,(#24299,#24300,#24301,#24302,#24303,
#24304,#24305,#24306,#24307,#24308,#24309,#24310,#24311,#24312,#24313,#24314,
#24315,#24316,#24317,#24318,#24319,#24320,#24321,#24322,#24323,#24324,#24325,
#24326,#24327,#24328,#24329,#24330,#24331,#24332,#24333,#24334),
 .UNSPECIFIED.,.F.,.F.,(4,2,2,2,2,2,2,2,2,2,2,2,2,2,2,2,2,4),(-21.3177166421035,
-21.2625812719389,-21.064165629947,-20.8721490272244,-20.673582562973,-20.4815649801061,
-20.2828512953899,-20.0908222560601,-19.8919650794903,-19.6999150834194,
-19.5009182308336,-19.3088387501402,-19.1097060879411,-18.9175895474012,
-18.7183249591171,-18.5261647028704,-18.3267720591113,-18.1648534816952),
 .UNSPECIFIED.);
#936=B_SPLINE_CURVE_WITH_KNOTS('',3,(#24335,#24336,#24337,#24338,#24339,
#24340,#24341,#24342,#24343,#24344,#24345,#24346,#24347,#24348,#24349,#24350,
#24351,#24352,#24353,#24354,#24355,#24356,#24357,#24358,#24359,#24360,#24361,
#24362,#24363,#24364,#24365,#24366,#24367,#24368,#24369,#24370),
 .UNSPECIFIED.,.F.,.F.,(4,2,2,2,2,2,2,2,2,2,2,2,2,2,2,2,2,4),(-22.894653858858,
-22.8430351800972,-22.6481796696925,-22.4523904874596,-22.2576546387054,
-22.0615952329455,-21.8669725741083,-21.6706439608552,-21.4761278826948,
-21.2795321828928,-21.0851159879305,-20.8882563232672,-20.6939332725896,
-20.4968136557196,-20.3025770127114,-20.1052022348834,-19.911045305434,
-19.7420141160744),.UNSPECIFIED.);
#937=B_SPLINE_CURVE_WITH_KNOTS('',3,(#24375,#24376,#24377,#24378,#24379,
#24380,#24381,#24382,#24383,#24384,#24385,#24386,#24387,#24388,#24389,#24390,
#24391,#24392,#24393,#24394,#24395,#24396,#24397,#24398,#24399,#24400,#24401,
#24402,#24403,#24404,#24405,#24406,#24407,#24408,#24409,#24410),
 .UNSPECIFIED.,.F.,.F.,(4,2,2,2,2,2,2,2,2,2,2,2,2,2,2,2,2,4),(-24.4694816405073,
-24.3817664053116,-24.184657336375,-23.9921690598734,-23.7948901903441,
-23.6025135998707,-23.4050659356891,-23.2127850875403,-23.0151701076872,
-22.8229693137646,-22.625188932334,-22.4330529221295,-22.2351094468282,
-22.0430235119941,-21.84491960015,-21.6528697189484,-21.4546083320897,-21.3177166421035),
 .UNSPECIFIED.);
#938=B_SPLINE_CURVE_WITH_KNOTS('',3,(#24411,#24412,#24413,#24414,#24415,
#24416,#24417,#24418,#24419,#24420,#24421,#24422,#24423,#24424,#24425,#24426,
#24427,#24428,#24429,#24430,#24431,#24432,#24433,#24434,#24435,#24436,#24437,
#24438,#24439,#24440,#24441,#24442,#24443,#24444,#24445,#24446),
 .UNSPECIFIED.,.F.,.F.,(4,2,2,2,2,2,2,2,2,2,2,2,2,2,2,2,2,4),(-19.7420141160744,
-19.7134208241997,-19.5193369930586,-19.3214688202648,-19.1217779356284,
-18.9294364317553,-18.7296310935017,-18.5372255598661,-18.3373092864661,
-18.1448372418786,-17.9448134301776,-17.7522729260411,-17.5521448443219,
-17.3595344029897,-17.1593051843462,-16.9666237403786,-16.7662963782371,
-16.5866685152428),.UNSPECIFIED.);
#939=B_SPLINE_CURVE_WITH_KNOTS('',3,(#24451,#24452,#24453,#24454,#24455,
#24456,#24457,#24458,#24459,#24460,#24461,#24462,#24463,#24464,#24465,#24466,
#24467,#24468,#24469,#24470,#24471,#24472,#24473,#24474,#24475,#24476,#24477,
#24478,#24479,#24480,#24481,#24482,#24483,#24484,#24485,#24486),
 .UNSPECIFIED.,.F.,.F.,(4,2,2,2,2,2,2,2,2,2,2,2,2,2,2,2,2,4),(-27.6210776549999,
-27.4991473095919,-27.3015146936668,-27.1092429712434,-26.9117774887184,
-26.7194116960812,-26.5221148737608,-26.3296390861027,-26.1325119815572,
-25.9399101751814,-25.7429533429172,-25.5502095797723,-25.353423042936,
-25.1605216602857,-24.9639048847822,-24.770830509061,-24.57438239134,-24.4694816405073),
 .UNSPECIFIED.);
#940=B_SPLINE_CURVE_WITH_KNOTS('',3,(#24487,#24488,#24489,#24490,#24491,
#24492,#24493,#24494,#24495,#24496,#24497,#24498,#24499,#24500,#24501,#24502,
#24503,#24504,#24505,#24506,#24507,#24508,#24509,#24510,#24511,#24512,#24513,
#24514,#24515,#24516,#24517,#24518,#24519,#24520,#24521,#24522),
 .UNSPECIFIED.,.F.,.F.,(4,2,2,2,2,2,2,2,2,2,2,2,2,2,2,2,2,4),(-16.5866685152428,
-16.5735432232291,-16.3731205687638,-16.1802953001972,-15.979780061394,
-15.7868825357782,-15.5862772779135,-15.39330756832,-15.1926147156369,-14.9995730736048,
-14.7987949119831,-14.6056817336746,-14.4048204141143,-14.2116362105224,
-14.0106937532715,-13.8174391242358,-13.6164174234198,-13.4271423741323),
 .UNSPECIFIED.);
#941=B_SPLINE_CURVE_WITH_KNOTS('',3,(#24527,#24528,#24529,#24530,#24531,
#24532,#24533,#24534,#24535,#24536,#24537,#24538,#24539,#24540,#24541,#24542,
#24543,#24544,#24545,#24546,#24547,#24548,#24549,#24550,#24551,#24552,#24553,
#24554,#24555,#24556,#24557,#24558,#24559,#24560,#24561,#24562),
 .UNSPECIFIED.,.F.,.F.,(4,2,2,2,2,2,2,2,2,2,2,2,2,2,2,2,2,4),(-30.7732540162916,
-30.6224625534038,-30.4235903739139,-30.2315594873663,-30.0328304001711,
-29.8408120197825,-29.6422297645305,-29.4502135167174,-29.2517817105492,
-29.0597562579787,-28.8614783536651,-28.6694314282219,-28.4713106702696,
-28.2792291277839,-28.0812685071763,-27.8891384048115,-27.6913406131706,
-27.6210776549999),.UNSPECIFIED.);
#942=B_SPLINE_CURVE_WITH_KNOTS('',3,(#24563,#24564,#24565,#24566,#24567,
#24568,#24569,#24570,#24571,#24572,#24573,#24574,#24575,#24576,#24577,#24578,
#24579,#24580,#24581,#24582,#24583,#24584,#24585,#24586,#24587,#24588,#24589,
#24590,#24591,#24592,#24593,#24594,#24595,#24596,#24597,#24598,#24599,#24600),
 .UNSPECIFIED.,.F.,.F.,(4,2,2,2,2,2,2,2,2,2,2,2,2,2,2,2,2,2,4),(-13.4271423741323,
-13.4230930351638,-13.2219938637853,-13.0286004296796,-12.827425444877,
-12.6339637091196,-12.4327144575865,-12.2391851814991,-12.0378631049865,
-11.8442670556327,-11.6428734964602,-11.4492114373098,-11.2477476438319,
-11.0540203272119,-10.8524874591921,-10.6587180709674,-10.457263865068,
-10.2635182555291,-10.262509796578),.UNSPECIFIED.);
#943=B_SPLINE_CURVE_WITH_KNOTS('',3,(#24605,#24606,#24607,#24608,#24609,
#24610,#24611,#24612,#24613,#24614,#24615,#24616,#24617,#24618,#24619,#24620,
#24621,#24622,#24623,#24624,#24625,#24626,#24627,#24628,#24629,#24630,#24631,
#24632,#24633,#24634,#24635,#24636,#24637,#24638,#24639,#24640),
 .UNSPECIFIED.,.F.,.F.,(4,2,2,2,2,2,2,2,2,2,2,2,2,2,2,2,2,4),(-33.9272264020338,
-33.7557592376309,-33.5558801431226,-33.3634883384545,-33.1637220538787,
-32.9713927215123,-32.7717428228324,-32.5794725404251,-32.3799427040667,
-32.1877273544111,-31.9883213410583,-31.7961560494673,-31.5968776846587,
-31.4047567598856,-31.2056099112557,-31.0135267921333,-30.814515343206,
-30.7732540162916),.UNSPECIFIED.);
#944=B_SPLINE_CURVE_WITH_KNOTS('',3,(#24641,#24642,#24643,#24644,#24645,
#24646,#24647,#24648,#24649,#24650,#24651,#24652,#24653,#24654,#24655,#24656,
#24657,#24658,#24659,#24660,#24661,#24662,#24663,#24664,#24665,#24666,#24667,
#24668,#24669,#24670,#24671,#24672,#24673,#24674,#24675,#24676),
 .UNSPECIFIED.,.F.,.F.,(4,2,2,2,2,2,2,2,2,2,2,2,2,2,2,2,2,4),(-10.262509796578,
-10.0621748049494,-9.86845075919977,-9.66722218278625,-9.47351732981415,
-9.27240799880696,-9.07871980290119,-8.87773434771368,-8.68406009983074,
-8.48320341539374,-8.28954022456674,-8.08881747388833,-7.89516225877231,
-7.69457887431953,-7.5009283550059,-7.30049003747721,-7.10684072770255,
-7.09973172643055),.UNSPECIFIED.);
#945=B_SPLINE_CURVE_WITH_KNOTS('',3,(#24681,#24682,#24683,#24684,#24685,
#24686,#24687,#24688,#24689,#24690,#24691,#24692,#24693,#24694,#24695,#24696,
#24697,#24698,#24699,#24700,#24701,#24702,#24703,#24704,#24705,#24706,#24707,
#24708,#24709,#24710,#24711,#24712,#24713,#24714,#24715,#24716),
 .UNSPECIFIED.,.F.,.F.,(4,2,2,2,2,2,2,2,2,2,2,2,2,2,2,2,2,4),(-37.0845565341341,
-36.9000799964494,-36.6994119173651,-36.5064598623789,-36.3058806641965,
-36.1130008645257,-35.9125130467586,-35.719705464902,-35.5193116691429,
-35.3265760288943,-35.1262790398785,-34.9336147815065,-34.7334175268641,
-34.540823757936,-34.3407293064061,-34.1482047484434,-33.948216306308,-33.9272264020338),
 .UNSPECIFIED.);
#946=B_SPLINE_CURVE_WITH_KNOTS('',3,(#24717,#24718,#24719,#24720,#24721,
#24722,#24723,#24724,#24725,#24726,#24727,#24728,#24729,#24730,#24731,#24732,
#24733,#24734,#24735,#24736,#24737,#24738,#24739,#24740,#24741,#24742,#24743,
#24744,#24745,#24746,#24747,#24748,#24749,#24750,#24751,#24752),
 .UNSPECIFIED.,.F.,.F.,(4,2,2,2,2,2,2,2,2,2,2,2,2,2,2,2,2,4),(-7.09973172643055,
-6.90655344170533,-6.71290164162491,-6.51277160774573,-6.31911339745019,
-6.11914708016145,-5.92547831414216,-5.72568240496176,-5.53199870774885,
-5.33238010304901,-5.13867686627481,-4.93924263913638,-4.74551502028898,
-4.54627238580402,-4.3525153089586,-4.15347158241934,-3.9596797412452,-3.94188496449128),
 .UNSPECIFIED.);
#947=B_SPLINE_CURVE_WITH_KNOTS('',3,(#24757,#24758,#24759,#24760,#24761,
#24762,#24763,#24764,#24765,#24766,#24767,#24768,#24769,#24770,#24771,#24772,
#24773,#24774,#24775,#24776,#24777,#24778,#24779,#24780,#24781,#24782,#24783,
#24784,#24785,#24786,#24787,#24788,#24789,#24790,#24791,#24792),
 .UNSPECIFIED.,.F.,.F.,(4,2,2,2,2,2,2,2,2,2,2,2,2,2,2,2,2,4),(-40.2466139348711,
-40.0545403932037,-39.8532352583116,-39.6597210230983,-39.4584894779182,
-39.2650431981048,-39.063886739874,-38.8705091692816,-38.6694294031336,
-38.4761212714501,-38.2751199158824,-38.0818819135985,-37.8809608058188,
-37.687793566387,-37.4869546674465,-37.2938587463589,-37.0931041459699,
-37.0845565341341),.UNSPECIFIED.);
#948=B_SPLINE_CURVE_WITH_KNOTS('',3,(#24793,#24794,#24795,#24796,#24797,
#24798,#24799,#24800,#24801,#24802,#24803,#24804,#24805,#24806,#24807,#24808,
#24809,#24810,#24811,#24812,#24813,#24814,#24815,#24816,#24817,#24818,#24819,
#24820,#24821,#24822,#24823,#24824,#24825,#24826,#24827,#24828),
 .UNSPECIFIED.,.F.,.F.,(4,2,2,2,2,2,2,2,2,2,2,2,2,2,2,2,2,4),(-3.94188496449128,
-3.76084228872693,-3.56701015207919,-3.36838633300804,-3.17450815341289,
-2.97610525484641,-2.7821750801714,-2.58400024268388,-2.39001193128194,
-2.19207206656769,-1.99801930613313,-1.80032100669122,-1.60619733703843,
-1.40874677861415,-1.21454561850871,-1.01734845629544,-0.823063134397515,
-0.787742139522384),.UNSPECIFIED.);
#949=B_SPLINE_CURVE_WITH_KNOTS('',3,(#24831,#24832,#24833,#24834,#24835,
#24836,#24837,#24838,#24839,#24840,#24841,#24842),.UNSPECIFIED.,.F.,.F.,
(4,2,2,2,2,4),(-0.787742139522384,-0.626124599551191,-0.43174863618738,
-0.235072853109506,-0.116437106936023,-9.99999992812306E-7),
 .UNSPECIFIED.);
#950=B_SPLINE_CURVE_WITH_KNOTS('',3,(#24845,#24846,#24847,#24848,#24849,
#24850,#24851,#24852),.UNSPECIFIED.,.F.,.F.,(4,2,2,4),(-40.6422236169032,
-40.4452026475075,-40.2481218184496,-40.2466139348711),.UNSPECIFIED.);
#951=B_SPLINE_CURVE_WITH_KNOTS('',3,(#24879,#24880,#24881,#24882,#24883,
#24884,#24885,#24886,#24887,#24888,#24889,#24890),.UNSPECIFIED.,.F.,.F.,
(4,2,2,2,2,4),(-2.81763482151145,-2.66615582776095,-2.46478441849091,-2.19827513744825,
-1.9545528152173,-1.82223598960404),.UNSPECIFIED.);
#952=B_SPLINE_CURVE_WITH_KNOTS('',3,(#24895,#24896,#24897,#24898,#24899,
#24900,#24901,#24902,#24903,#24904,#24905,#24906,#24907,#24908,#24909,#24910,
#24911,#24912,#24913,#24914,#24915,#24916,#24917,#24918,#24919,#24920),
 .UNSPECIFIED.,.F.,.F.,(4,2,2,2,2,2,2,2,2,2,2,2,4),(-1.82223598960404,-1.7229258160528,
-1.51102009351715,-1.30997005387127,-1.21842619461754,-1.04088214590786,
-0.861129971477336,-0.676603178308848,-0.585954297377947,-0.411830214191357,
-0.231403986438724,-0.115329226334212,0.),.UNSPECIFIED.);
#953=B_SPLINE_CURVE_WITH_KNOTS('',3,(#24923,#24924,#24925,#24926,#24927,
#24928,#24929,#24930,#24931,#24932,#24933,#24934),.UNSPECIFIED.,.F.,.F.,
(4,2,2,2,2,4),(-0.353981642318911,-0.271813414514787,-0.183870482640077,
-0.100406136832525,-0.0580770708076673,0.),.UNSPECIFIED.);
#954=B_SPLINE_CURVE_WITH_KNOTS('',3,(#26251,#26252,#26253,#26254,#26255,
#26256,#26257,#26258,#26259,#26260,#26261,#26262,#26263,#26264,#26265,#26266,
#26267,#26268),.UNSPECIFIED.,.F.,.F.,(4,2,2,2,2,2,2,2,4),(23.6688063208097,
23.8680016439259,24.0616943144381,24.2627278650596,24.4564054848417,24.6573122520947,
24.8509776384353,25.0517525666804,25.2503481109993),.UNSPECIFIED.);
#955=B_SPLINE_CURVE_WITH_KNOTS('',3,(#26272,#26273,#26274,#26275,#26276,
#26277,#26278,#26279,#26280,#26281,#26282,#26283,#26284,#26285,#26286,#26287,
#26288,#26289,#26290,#26291),.UNSPECIFIED.,.F.,.F.,(4,2,2,2,2,2,2,2,2,4),
(0.,0.192309890628632,0.392950131878038,0.585822092254251,0.786391070426237,
0.979196478715363,1.17969285299266,1.37243094502364,1.57285327532948,1.5761150882838),
 .UNSPECIFIED.);
#956=B_SPLINE_CURVE_WITH_KNOTS('',3,(#26295,#26296,#26297,#26298,#26299,
#26300,#26301,#26302,#26303,#26304,#26305,#26306,#26307,#26308,#26309,#26310,
#26311,#26312,#26313,#26314,#26315,#26316,#26317,#26318,#26319,#26320,#26321,
#26322,#26323,#26324,#26325,#26326,#26327,#26328,#26329,#26330),
 .UNSPECIFIED.,.F.,.F.,(4,2,2,2,2,2,2,2,2,2,2,2,2,2,2,2,2,4),(1.5761150882838,
1.76552329302677,1.96587003453306,2.15847123733424,2.35874073498249,2.55127241358088,
2.75146289668655,2.94392438938976,3.1440339664105,3.33642467841756,3.53645133198428,
3.72877075788602,3.92871234020673,4.12096009000703,4.32081431877349,4.51299014771225,
4.71275460265744,4.72444996915763),.UNSPECIFIED.);
#957=B_SPLINE_CURVE_WITH_KNOTS('',3,(#26335,#26336,#26337,#26338,#26339,
#26340,#26341,#26342,#26343,#26344,#26345,#26346,#26347,#26348,#26349,#26350,
#26351,#26352,#26353,#26354,#26355,#26356,#26357,#26358,#26359,#26360,#26361,
#26362,#26363,#26364,#26365,#26366,#26367,#26368,#26369,#26370,#26371,#26372),
 .UNSPECIFIED.,.F.,.F.,(4,2,2,2,2,2,2,2,2,2,2,2,2,2,2,2,2,2,4),(20.5033787905061,
20.506181756931,20.707436476315,20.9009725341327,21.1023006757468,21.2959038362448,
21.4973040170517,21.6909735141241,21.8924444473212,22.0861795230845,22.2877200126867,
22.4814976181688,22.6829930094403,22.8767459939412,23.0781322065223,23.2718627249666,
23.4731357386561,23.6668460986838,23.6688063208097),.UNSPECIFIED.);
#958=B_SPLINE_CURVE_WITH_KNOTS('',3,(#26373,#26374,#26375,#26376,#26377,
#26378,#26379,#26380,#26381,#26382,#26383,#26384,#26385,#26386,#26387,#26388,
#26389,#26390,#26391,#26392,#26393,#26394,#26395,#26396,#26397,#26398,#26399,
#26400,#26401,#26402,#26403,#26404,#26405,#26406,#26407,#26408),
 .UNSPECIFIED.,.F.,.F.,(4,2,2,2,2,2,2,2,2,2,2,2,2,2,2,2,2,4),(4.72444996915763,
4.90485844507989,5.10453056535011,5.2965625728159,5.49613965534028,5.68810023909005,
5.88757943815145,6.0794693159494,6.27884764417189,6.47066789141356,6.66994222240167,
6.86169432721906,7.06086140009344,7.25254732199799,7.4516037480787,7.64322597946192,
7.8421682513544,7.86845984801116),.UNSPECIFIED.);
#959=B_SPLINE_CURVE_WITH_KNOTS('',3,(#26413,#26414,#26415,#26416,#26417,
#26418,#26419,#26420,#26421,#26422,#26423,#26424,#26425,#26426,#26427,#26428,
#26429,#26430,#26431,#26432,#26433,#26434,#26435,#26436,#26437,#26438,#26439,
#26440,#26441,#26442,#26443,#26444,#26445,#26446,#26447,#26448),
 .UNSPECIFIED.,.F.,.F.,(4,2,2,2,2,2,2,2,2,2,2,2,2,2,2,2,2,4),(17.3423091084718,
17.3532026119064,17.5538068254068,17.7467812232279,17.9474740334127,18.1405205000154,
18.341299563721,18.5344177588769,18.7352808693728,18.9284703261504,19.1294154092585,
19.3226755615564,19.5237006712113,19.7170308776452,19.9181341910316,20.1115337554729,
20.3127135678619,20.5033787905061),.UNSPECIFIED.);
#960=B_SPLINE_CURVE_WITH_KNOTS('',3,(#26449,#26450,#26451,#26452,#26453,
#26454,#26455,#26456,#26457,#26458,#26459,#26460,#26461,#26462,#26463,#26464,
#26465,#26466,#26467,#26468,#26469,#26470,#26471,#26472,#26473,#26474,#26475,
#26476,#26477,#26478,#26479,#26480,#26481,#26482,#26483,#26484),
 .UNSPECIFIED.,.F.,.F.,(4,2,2,2,2,2,2,2,2,2,2,2,2,2,2,2,2,4),(7.86845984801116,
8.03372988091695,8.23255438425071,8.4240591611593,8.62276218921183,8.81421458649587,
9.00793068521309,9.20384682448228,9.39766192439471,9.59331213805431,9.78723291767305,
9.98261501021267,10.1766480638836,10.3717609328959,10.5659127218738,10.7607564538351,
10.9550332555806,11.0096450714467),.UNSPECIFIED.);
#961=B_SPLINE_CURVE_WITH_KNOTS('',3,(#26489,#26490,#26491,#26492,#26493,
#26494,#26495,#26496,#26497,#26498,#26499,#26500,#26501,#26502,#26503,#26504,
#26505,#26506,#26507,#26508,#26509,#26510,#26511,#26512,#26513,#26514,#26515,
#26516,#26517,#26518,#26519,#26520,#26521,#26522,#26523,#26524),
 .UNSPECIFIED.,.F.,.F.,(4,2,2,2,2,2,2,2,2,2,2,2,2,2,2,2,2,4),(14.1856813666801,
14.2106556084505,14.4104497800149,14.602862920382,14.8027694881212,14.9952481928414,
15.1952637085973,15.387810139388,15.5879312801588,15.7805471024998,15.9807706780298,
16.1734571212125,16.3737800793295,16.5665379931835,16.7669574231372,16.9597873308951,
17.1603004649466,17.3423091084718),.UNSPECIFIED.);
#962=B_SPLINE_CURVE_WITH_KNOTS('',3,(#26525,#26526,#26527,#26528,#26529,
#26530,#26531,#26532,#26533,#26534,#26535,#26536,#26537,#26538,#26539,#26540,
#26541,#26542,#26543,#26544,#26545,#26546,#26547,#26548,#26549,#26550,#26551,
#26552,#26553,#26554,#26555,#26556,#26557,#26558,#26559,#26560),
 .UNSPECIFIED.,.F.,.F.,(4,2,2,2,2,2,2,2,2,2,2,2,2,2,2,2,2,4),(11.0096450714467,
11.1496092096788,11.3440170662402,11.5383279428451,11.7328726093068,11.926922499806,
12.1216093938707,12.3154038088951,12.5102379627232,12.7037838362626,12.8987698517158,
13.0920755192803,13.287217527673,13.4802926774533,13.6755943048501,13.8684499017687,
14.0639142407318,14.1497226382099),.UNSPECIFIED.);
#963=B_SPLINE_CURVE_WITH_KNOTS('',3,(#26565,#26566,#26567,#26568,#26569,
#26570,#26571,#26572,#26573,#26574,#26575,#26576,#26577,#26578,#26579,#26580,
#26581,#26582,#26583,#26584,#26585,#26586,#26587,#26588,#26589,#26590,#26591,
#26592,#26593,#26594,#26595,#26596,#26597,#26598,#26599,#26600),
 .UNSPECIFIED.,.F.,.F.,(4,2,2,2,2,2,2,2,2,2,2,2,2,2,2,2,2,4),(11.032043594273,
11.0791330610422,11.2738662174345,11.470065184074,11.6646875517819,11.8611551219302,
12.0601971336175,12.2522980304616,12.4514749854863,12.6436145256115,12.8429225405824,
13.0351071786466,13.2345423893918,13.4267777160951,13.6263363034536,13.8186270997122,
14.0183053118855,14.1856813666801),.UNSPECIFIED.);
#964=B_SPLINE_CURVE_WITH_KNOTS('',3,(#26601,#26602,#26603,#26604,#26605,
#26606,#26607,#26608,#26609,#26610,#26611,#26612,#26613,#26614,#26615,#26616,
#26617,#26618,#26619,#26620,#26621,#26622,#26623,#26624,#26625,#26626,#26627,
#26628,#26629,#26630,#26631,#26632,#26633,#26634,#26635,#26636),
 .UNSPECIFIED.,.F.,.F.,(4,2,2,2,2,2,2,2,2,2,2,2,2,2,2,2,2,4),(14.1497226382099,
14.2565624242763,14.452192012803,14.644645970566,14.8404427787485,15.0327165985864,
15.2286820237912,15.4207906366718,15.6169255143855,15.8088843871035,16.0051889839162,
16.1970138736636,16.3934879143908,16.5851947634573,16.7818374560417,16.9734422046251,
17.1702522710418,17.2895966666142),.UNSPECIFIED.);
#965=B_SPLINE_CURVE_WITH_KNOTS('',3,(#26641,#26642,#26643,#26644,#26645,
#26646,#26647,#26648,#26649,#26650,#26651,#26652,#26653,#26654,#26655,#26656,
#26657,#26658,#26659,#26660,#26661,#26662,#26663,#26664,#26665,#26666,#26667,
#26668,#26669,#26670,#26671,#26672,#26673,#26674,#26675,#26676),
 .UNSPECIFIED.,.F.,.F.,(4,2,2,2,2,2,2,2,2,2,2,2,2,2,2,2,2,4),(7.8798925984307,
7.95653091972942,8.1523647619255,8.34647021357625,8.54214862603429,8.73649776288571,
8.93202503348979,9.12662581805227,9.32200669581487,9.51686567465596,9.71210532789297,
9.90722761742384,10.1023315877192,10.2977208855736,10.4926950386617,10.6883536586088,
10.8832041333213,11.032043594273),.UNSPECIFIED.);
#966=B_SPLINE_CURVE_WITH_KNOTS('',3,(#26677,#26678,#26679,#26680,#26681,
#26682,#26683,#26684,#26685,#26686,#26687,#26688,#26689,#26690,#26691,#26692,
#26693,#26694,#26695,#26696,#26697,#26698,#26699,#26700,#26701,#26702,#26703,
#26704,#26705,#26706,#26707,#26708,#26709,#26710,#26711,#26712),
 .UNSPECIFIED.,.F.,.F.,(4,2,2,2,2,2,2,2,2,2,2,2,2,2,2,2,2,4),(17.2895966666142,
17.3617706775084,17.5587463897173,17.7501938628928,17.9473330828076,18.1387245302062,
18.336024752601,18.527374447667,18.7248328449502,18.9161543154852,19.1137677833141,
19.3050737223178,19.5028389250998,19.6941411243536,19.8920545397888,20.0833638456821,
20.2814218076159,20.4299877360611),.UNSPECIFIED.);
#967=B_SPLINE_CURVE_WITH_KNOTS('',3,(#26717,#26718,#26719,#26720,#26721,
#26722,#26723,#26724,#26725,#26726,#26727,#26728,#26729,#26730,#26731,#26732,
#26733,#26734,#26735,#26736,#26737,#26738,#26739,#26740,#26741,#26742,#26743,
#26744,#26745,#26746,#26747,#26748,#26749,#26750,#26751,#26752),
 .UNSPECIFIED.,.F.,.F.,(4,2,2,2,2,2,2,2,2,2,2,2,2,2,2,2,2,4),(4.72815874405663,
4.8384872813078,5.03565472956953,5.22824215554031,5.42523938450227,5.61796591852915,
5.81479280753122,6.00767417677815,6.20433115727545,6.39738279865264,6.59387087295077,
6.78710752149101,6.98342825882622,7.17686380974204,7.37301935402876,7.56666675378859,
7.762659815928,7.8798925984307),.UNSPECIFIED.);
#968=B_SPLINE_CURVE_WITH_KNOTS('',3,(#26753,#26754,#26755,#26756,#26757,
#26758,#26759,#26760,#26761,#26762,#26763,#26764,#26765,#26766,#26767,#26768,
#26769,#26770,#26771,#26772,#26773,#26774,#26775,#26776,#26777,#26778,#26779,
#26780,#26781,#26782,#26783,#26784,#26785,#26786,#26787,#26788),
 .UNSPECIFIED.,.F.,.F.,(4,2,2,2,2,2,2,2,2,2,2,2,2,2,2,2,2,4),(20.4299877360611,
20.472748098005,20.6709468369917,20.8622990173113,21.0606346984189,21.2520207148496,
21.4504894723635,21.6419163395927,21.8405143083974,22.0319881493852,22.2307114929069,
22.4222375880747,22.621082522768,22.8126653661272,23.0116281825616,23.2032715424857,
23.4023486231547,23.5720713493618),.UNSPECIFIED.);
#969=B_SPLINE_CURVE_WITH_KNOTS('',3,(#26794,#26795,#26796,#26797,#26798,
#26799,#26800,#26801,#26802,#26803,#26804,#26805),.UNSPECIFIED.,.F.,.F.,
(4,2,2,2,2,4),(26.717398205925,26.7265409725364,26.9265040240299,27.1188444098408,
27.31889260268,27.5043317305357),.UNSPECIFIED.);
#970=B_SPLINE_CURVE_WITH_KNOTS('',3,(#26808,#26809,#26810,#26811,#26812,
#26813,#26814,#26815,#26816,#26817,#26818,#26819,#26820,#26821,#26822,#26823,
#26824,#26825,#26826,#26827),.UNSPECIFIED.,.F.,.F.,(4,2,2,2,2,2,2,2,2,4),
(0.,0.175931162978202,0.353160743648948,0.545227872409306,0.74413522592968,
0.936178861517958,1.13494379915102,1.32697316334426,1.52559192745073,1.57613829627577),
 .UNSPECIFIED.);
#971=B_SPLINE_CURVE_WITH_KNOTS('',3,(#26829,#26830,#26831,#26832,#26833,
#26834,#26835,#26836,#26837,#26838,#26839,#26840,#26841,#26842,#26843,#26844,
#26845,#26846,#26847,#26848,#26849,#26850,#26851,#26852,#26853,#26854,#26855,
#26856,#26857,#26858,#26859,#26860,#26861,#26862,#26863,#26864),
 .UNSPECIFIED.,.F.,.F.,(4,2,2,2,2,2,2,2,2,2,2,2,2,2,2,2,2,4),(1.57613829627577,
1.71761721885756,1.91608616703187,2.10811855179259,2.30643419830044,2.4984857808909,
2.69664484024402,2.88872861275038,3.08672804477878,3.27885781362127,3.47669486927162,
3.6688851591046,3.86655742608426,4.05882336145931,4.25632880874467,4.44868597504655,
4.64602299520801,4.72815874405663),.UNSPECIFIED.);
#972=B_SPLINE_CURVE_WITH_KNOTS('',3,(#26865,#26866,#26867,#26868,#26869,
#26870,#26871,#26872,#26873,#26874,#26875,#26876,#26877,#26878,#26879,#26880,
#26881,#26882,#26883,#26884,#26885,#26886,#26887,#26888,#26889,#26890,#26891,
#26892,#26893,#26894,#26895,#26896,#26897,#26898,#26899,#26900),
 .UNSPECIFIED.,.F.,.F.,(4,2,2,2,2,2,2,2,2,2,2,2,2,2,2,2,2,4),(23.5720713493618,
23.5940556057397,23.7932434397696,23.9850165529989,24.184311747963,24.3761529651803,
24.5755522562542,24.767463077738,24.9669633344463,25.1589448461464,25.3585430769529,
25.550596005705,25.7502893607003,25.9424141254523,26.1421998973837,26.3343966561616,
26.5342722800385,26.717398205925),.UNSPECIFIED.);
#973=B_SPLINE_CURVE_WITH_KNOTS('',3,(#26932,#26933,#26934,#26935,#26936,
#26937,#26938,#26939,#26940,#26941,#26942,#26943,#26944,#26945),
 .UNSPECIFIED.,.F.,.F.,(4,2,2,2,2,2,4),(-1.09561114978705,-0.811392982779186,
-0.600348101262501,-0.377067356850475,-0.216075223113698,-0.119074012181648,
0.),.UNSPECIFIED.);
#974=B_SPLINE_CURVE_WITH_KNOTS('',3,(#26946,#26947,#26948,#26949,#26950,
#26951,#26952,#26953,#26954,#26955,#26956,#26957,#26958,#26959),
 .UNSPECIFIED.,.F.,.F.,(4,2,2,2,2,2,4),(-0.920708721485626,-0.810769067465036,
-0.701870911977783,-0.530236332505368,-0.314467713567416,-0.153407050270327,
0.),.UNSPECIFIED.);
#1184=CYLINDRICAL_SURFACE('',#13542,5.00000000000001);
#1185=CYLINDRICAL_SURFACE('',#13548,20.);
#1186=CYLINDRICAL_SURFACE('',#13552,20.);
#1187=CYLINDRICAL_SURFACE('',#13553,25.);
#1188=CYLINDRICAL_SURFACE('',#13567,4.90000000000001);
#1189=CYLINDRICAL_SURFACE('',#13570,4.45873412499923);
#1190=CYLINDRICAL_SURFACE('',#13571,4.45873412499923);
#1191=CYLINDRICAL_SURFACE('',#13572,4.45873412499923);
#1192=CYLINDRICAL_SURFACE('',#13573,4.45873412499923);
#1193=CYLINDRICAL_SURFACE('',#13574,4.45873412499923);
#1194=CYLINDRICAL_SURFACE('',#13575,4.45873412499923);
#1195=CYLINDRICAL_SURFACE('',#13576,4.45873412499923);
#1196=CYLINDRICAL_SURFACE('',#13577,4.45873412499923);
#1197=CYLINDRICAL_SURFACE('',#13578,4.45873412499923);
#1198=CYLINDRICAL_SURFACE('',#13579,4.45873412499923);
#1199=CYLINDRICAL_SURFACE('',#13580,4.45873412499923);
#1200=CYLINDRICAL_SURFACE('',#13581,4.45873412499923);
#1201=CYLINDRICAL_SURFACE('',#13582,4.45873412499923);
#1202=CYLINDRICAL_SURFACE('',#13583,5.00000000000001);
#1203=CYLINDRICAL_SURFACE('',#13585,5.00000000000001);
#1204=CYLINDRICAL_SURFACE('',#13586,5.00000000000001);
#1205=CYLINDRICAL_SURFACE('',#13587,5.00000000000001);
#1206=CYLINDRICAL_SURFACE('',#13588,5.00000000000001);
#1207=CYLINDRICAL_SURFACE('',#13589,5.00000000000001);
#1208=CYLINDRICAL_SURFACE('',#13590,5.00000000000001);
#1209=CYLINDRICAL_SURFACE('',#13591,5.00000000000001);
#1210=CYLINDRICAL_SURFACE('',#13592,5.00000000000001);
#1211=CYLINDRICAL_SURFACE('',#13593,5.00000000000001);
#1212=CYLINDRICAL_SURFACE('',#13594,5.00000000000001);
#1213=CYLINDRICAL_SURFACE('',#13595,5.00000000000001);
#1214=CYLINDRICAL_SURFACE('',#13596,5.00000000000001);
#1215=CYLINDRICAL_SURFACE('',#13598,9.99999999999999);
#1216=CYLINDRICAL_SURFACE('',#13604,5.);
#1217=CYLINDRICAL_SURFACE('',#13607,5.);
#1218=CYLINDRICAL_SURFACE('',#13637,9.);
#1219=CYLINDRICAL_SURFACE('',#13638,9.);
#1220=CYLINDRICAL_SURFACE('',#13648,4.45873412499923);
#1221=CYLINDRICAL_SURFACE('',#13649,4.99999999999998);
#1222=CYLINDRICAL_SURFACE('',#13650,4.99999999999998);
#1223=CYLINDRICAL_SURFACE('',#13651,2.00000000000001);
#1224=CYLINDRICAL_SURFACE('',#13652,2.00000000000001);
#1225=CYLINDRICAL_SURFACE('',#13653,5.54126587500002);
#1226=CYLINDRICAL_SURFACE('',#13655,5.54126587500002);
#1227=CYLINDRICAL_SURFACE('',#13656,5.54126587500002);
#1228=CYLINDRICAL_SURFACE('',#13657,5.54126587500002);
#1229=CYLINDRICAL_SURFACE('',#13658,5.54126587500002);
#1230=CYLINDRICAL_SURFACE('',#13659,5.54126587500002);
#1231=CYLINDRICAL_SURFACE('',#13660,5.54126587500002);
#1232=CYLINDRICAL_SURFACE('',#13661,5.54126587500002);
#1233=CYLINDRICAL_SURFACE('',#13662,5.);
#1234=CYLINDRICAL_SURFACE('',#13664,5.);
#1235=CYLINDRICAL_SURFACE('',#13665,5.);
#1236=CYLINDRICAL_SURFACE('',#13666,5.);
#1237=CYLINDRICAL_SURFACE('',#13667,5.);
#1238=CYLINDRICAL_SURFACE('',#13668,5.);
#1239=CYLINDRICAL_SURFACE('',#13669,5.);
#1240=CYLINDRICAL_SURFACE('',#13670,5.);
#1241=CYLINDRICAL_SURFACE('',#13672,5.);
#1242=CYLINDRICAL_SURFACE('',#13673,9.99999999999999);
#1243=CYLINDRICAL_SURFACE('',#13686,5.54126587500002);
#1816=FACE_OUTER_BOUND('',#2611,.T.);
#1817=FACE_OUTER_BOUND('',#2612,.T.);
#1818=FACE_OUTER_BOUND('',#2613,.T.);
#1819=FACE_OUTER_BOUND('',#2614,.T.);
#1820=FACE_OUTER_BOUND('',#2615,.T.);
#1821=FACE_OUTER_BOUND('',#2616,.T.);
#1822=FACE_OUTER_BOUND('',#2617,.T.);
#1823=FACE_OUTER_BOUND('',#2618,.T.);
#1824=FACE_OUTER_BOUND('',#2619,.T.);
#1825=FACE_OUTER_BOUND('',#2620,.T.);
#1826=FACE_OUTER_BOUND('',#2621,.T.);
#1827=FACE_OUTER_BOUND('',#2622,.T.);
#1828=FACE_OUTER_BOUND('',#2623,.T.);
#1829=FACE_OUTER_BOUND('',#2625,.T.);
#1830=FACE_OUTER_BOUND('',#2627,.T.);
#1831=FACE_OUTER_BOUND('',#2629,.T.);
#1832=FACE_OUTER_BOUND('',#2631,.T.);
#1833=FACE_OUTER_BOUND('',#2633,.T.);
#1834=FACE_OUTER_BOUND('',#2635,.T.);
#1835=FACE_OUTER_BOUND('',#2636,.T.);
#1836=FACE_OUTER_BOUND('',#2637,.T.);
#1837=FACE_OUTER_BOUND('',#2638,.T.);
#1838=FACE_OUTER_BOUND('',#2639,.T.);
#1839=FACE_OUTER_BOUND('',#2640,.T.);
#1840=FACE_OUTER_BOUND('',#2641,.T.);
#1841=FACE_OUTER_BOUND('',#2642,.T.);
#1842=FACE_OUTER_BOUND('',#2643,.T.);
#1843=FACE_OUTER_BOUND('',#2644,.T.);
#1844=FACE_OUTER_BOUND('',#2645,.T.);
#1845=FACE_OUTER_BOUND('',#2646,.T.);
#1846=FACE_OUTER_BOUND('',#2647,.T.);
#1847=FACE_OUTER_BOUND('',#2648,.T.);
#1848=FACE_OUTER_BOUND('',#2649,.T.);
#1849=FACE_OUTER_BOUND('',#2650,.T.);
#1850=FACE_OUTER_BOUND('',#2651,.T.);
#1851=FACE_OUTER_BOUND('',#2652,.T.);
#1852=FACE_OUTER_BOUND('',#2653,.T.);
#1853=FACE_OUTER_BOUND('',#2654,.T.);
#1854=FACE_OUTER_BOUND('',#2655,.T.);
#1855=FACE_OUTER_BOUND('',#2656,.T.);
#1856=FACE_OUTER_BOUND('',#2657,.T.);
#1857=FACE_OUTER_BOUND('',#2658,.T.);
#1858=FACE_OUTER_BOUND('',#2659,.T.);
#1859=FACE_OUTER_BOUND('',#2660,.T.);
#1860=FACE_OUTER_BOUND('',#2661,.T.);
#1861=FACE_OUTER_BOUND('',#2662,.T.);
#1862=FACE_OUTER_BOUND('',#2663,.T.);
#1863=FACE_OUTER_BOUND('',#2664,.T.);
#1864=FACE_OUTER_BOUND('',#2665,.T.);
#1865=FACE_OUTER_BOUND('',#2666,.T.);
#1866=FACE_OUTER_BOUND('',#2667,.T.);
#1867=FACE_OUTER_BOUND('',#2668,.T.);
#1868=FACE_OUTER_BOUND('',#2669,.T.);
#1869=FACE_OUTER_BOUND('',#2670,.T.);
#1870=FACE_OUTER_BOUND('',#2671,.T.);
#1871=FACE_OUTER_BOUND('',#2672,.T.);
#1872=FACE_OUTER_BOUND('',#2674,.T.);
#1873=FACE_OUTER_BOUND('',#2676,.T.);
#1874=FACE_OUTER_BOUND('',#2677,.T.);
#1875=FACE_OUTER_BOUND('',#2679,.T.);
#1876=FACE_OUTER_BOUND('',#2681,.T.);
#1877=FACE_OUTER_BOUND('',#2682,.T.);
#1878=FACE_OUTER_BOUND('',#2683,.T.);
#1879=FACE_OUTER_BOUND('',#2684,.T.);
#1880=FACE_OUTER_BOUND('',#2685,.T.);
#1881=FACE_OUTER_BOUND('',#2686,.T.);
#1882=FACE_OUTER_BOUND('',#2687,.T.);
#1883=FACE_OUTER_BOUND('',#2688,.T.);
#1884=FACE_OUTER_BOUND('',#2689,.T.);
#1885=FACE_OUTER_BOUND('',#2690,.T.);
#1886=FACE_OUTER_BOUND('',#2692,.T.);
#1887=FACE_OUTER_BOUND('',#2693,.T.);
#1888=FACE_OUTER_BOUND('',#2694,.T.);
#1889=FACE_OUTER_BOUND('',#2695,.T.);
#1890=FACE_OUTER_BOUND('',#2696,.T.);
#1891=FACE_OUTER_BOUND('',#2697,.T.);
#1892=FACE_OUTER_BOUND('',#2698,.T.);
#1893=FACE_OUTER_BOUND('',#2699,.T.);
#1894=FACE_OUTER_BOUND('',#2700,.T.);
#1895=FACE_OUTER_BOUND('',#2701,.T.);
#1896=FACE_OUTER_BOUND('',#2702,.T.);
#1897=FACE_OUTER_BOUND('',#2703,.T.);
#1898=FACE_OUTER_BOUND('',#2704,.T.);
#1899=FACE_OUTER_BOUND('',#2705,.T.);
#1900=FACE_OUTER_BOUND('',#2706,.T.);
#1901=FACE_OUTER_BOUND('',#2707,.T.);
#1902=FACE_OUTER_BOUND('',#2708,.T.);
#1903=FACE_OUTER_BOUND('',#2709,.T.);
#1904=FACE_OUTER_BOUND('',#2710,.T.);
#1905=FACE_OUTER_BOUND('',#2711,.T.);
#1906=FACE_OUTER_BOUND('',#2712,.T.);
#1907=FACE_OUTER_BOUND('',#2713,.T.);
#1908=FACE_OUTER_BOUND('',#2714,.T.);
#1909=FACE_OUTER_BOUND('',#2715,.T.);
#1910=FACE_OUTER_BOUND('',#2716,.T.);
#1911=FACE_OUTER_BOUND('',#2717,.T.);
#1912=FACE_OUTER_BOUND('',#2718,.T.);
#1913=FACE_OUTER_BOUND('',#2719,.T.);
#1914=FACE_OUTER_BOUND('',#2721,.T.);
#1915=FACE_OUTER_BOUND('',#2723,.T.);
#1916=FACE_OUTER_BOUND('',#2725,.T.);
#1917=FACE_OUTER_BOUND('',#2726,.T.);
#1918=FACE_OUTER_BOUND('',#2727,.T.);
#1919=FACE_OUTER_BOUND('',#2728,.T.);
#1920=FACE_OUTER_BOUND('',#2729,.T.);
#1921=FACE_OUTER_BOUND('',#2730,.T.);
#1922=FACE_OUTER_BOUND('',#2731,.T.);
#1923=FACE_OUTER_BOUND('',#2732,.T.);
#1924=FACE_OUTER_BOUND('',#2733,.T.);
#1925=FACE_OUTER_BOUND('',#2734,.T.);
#1926=FACE_OUTER_BOUND('',#2735,.T.);
#1927=FACE_OUTER_BOUND('',#2736,.T.);
#1928=FACE_OUTER_BOUND('',#2737,.T.);
#1929=FACE_OUTER_BOUND('',#2738,.T.);
#1930=FACE_OUTER_BOUND('',#2739,.T.);
#1931=FACE_OUTER_BOUND('',#2740,.T.);
#2611=EDGE_LOOP('',(#10647,#10648,#10649,#10650,#10651));
#2612=EDGE_LOOP('',(#10652,#10653,#10654,#10655));
#2613=EDGE_LOOP('',(#10656,#10657,#10658,#10659,#10660));
#2614=EDGE_LOOP('',(#10661,#10662,#10663,#10664));
#2615=EDGE_LOOP('',(#10665,#10666,#10667,#10668,#10669));
#2616=EDGE_LOOP('',(#10670,#10671,#10672,#10673,#10674));
#2617=EDGE_LOOP('',(#10675,#10676,#10677,#10678));
#2618=EDGE_LOOP('',(#10679,#10680,#10681,#10682));
#2619=EDGE_LOOP('',(#10683,#10684,#10685,#10686));
#2620=EDGE_LOOP('',(#10687,#10688,#10689,#10690));
#2621=EDGE_LOOP('',(#10691,#10692,#10693,#10694,#10695,#10696));
#2622=EDGE_LOOP('',(#10697,#10698,#10699,#10700,#10701,#10702));
#2623=EDGE_LOOP('',(#10703));
#2624=EDGE_LOOP('',(#10704));
#2625=EDGE_LOOP('',(#10705));
#2626=EDGE_LOOP('',(#10706));
#2627=EDGE_LOOP('',(#10707));
#2628=EDGE_LOOP('',(#10708));
#2629=EDGE_LOOP('',(#10709));
#2630=EDGE_LOOP('',(#10710));
#2631=EDGE_LOOP('',(#10711));
#2632=EDGE_LOOP('',(#10712));
#2633=EDGE_LOOP('',(#10713));
#2634=EDGE_LOOP('',(#10714));
#2635=EDGE_LOOP('',(#10715,#10716,#10717,#10718));
#2636=EDGE_LOOP('',(#10719,#10720,#10721,#10722,#10723));
#2637=EDGE_LOOP('',(#10724,#10725,#10726,#10727,#10728));
#2638=EDGE_LOOP('',(#10729));
#2639=EDGE_LOOP('',(#10730));
#2640=EDGE_LOOP('',(#10731,#10732,#10733,#10734));
#2641=EDGE_LOOP('',(#10735,#10736,#10737,#10738));
#2642=EDGE_LOOP('',(#10739,#10740,#10741,#10742));
#2643=EDGE_LOOP('',(#10743,#10744,#10745,#10746));
#2644=EDGE_LOOP('',(#10747,#10748,#10749,#10750));
#2645=EDGE_LOOP('',(#10751,#10752,#10753,#10754));
#2646=EDGE_LOOP('',(#10755,#10756,#10757,#10758));
#2647=EDGE_LOOP('',(#10759,#10760,#10761,#10762));
#2648=EDGE_LOOP('',(#10763,#10764,#10765,#10766));
#2649=EDGE_LOOP('',(#10767,#10768,#10769,#10770));
#2650=EDGE_LOOP('',(#10771,#10772,#10773,#10774));
#2651=EDGE_LOOP('',(#10775,#10776,#10777,#10778));
#2652=EDGE_LOOP('',(#10779,#10780,#10781,#10782));
#2653=EDGE_LOOP('',(#10783,#10784,#10785,#10786,#10787,#10788,#10789,#10790));
#2654=EDGE_LOOP('',(#10791,#10792,#10793,#10794));
#2655=EDGE_LOOP('',(#10795,#10796,#10797,#10798));
#2656=EDGE_LOOP('',(#10799,#10800,#10801,#10802));
#2657=EDGE_LOOP('',(#10803,#10804,#10805,#10806));
#2658=EDGE_LOOP('',(#10807,#10808,#10809,#10810));
#2659=EDGE_LOOP('',(#10811,#10812,#10813,#10814));
#2660=EDGE_LOOP('',(#10815,#10816,#10817,#10818));
#2661=EDGE_LOOP('',(#10819,#10820,#10821,#10822));
#2662=EDGE_LOOP('',(#10823,#10824,#10825,#10826));
#2663=EDGE_LOOP('',(#10827,#10828,#10829,#10830));
#2664=EDGE_LOOP('',(#10831,#10832,#10833,#10834));
#2665=EDGE_LOOP('',(#10835,#10836,#10837,#10838));
#2666=EDGE_LOOP('',(#10839,#10840,#10841,#10842,#10843,#10844,#10845));
#2667=EDGE_LOOP('',(#10846,#10847,#10848,#10849));
#2668=EDGE_LOOP('',(#10850,#10851,#10852,#10853));
#2669=EDGE_LOOP('',(#10854,#10855,#10856,#10857,#10858,#10859,#10860,#10861));
#2670=EDGE_LOOP('',(#10862,#10863,#10864,#10865,#10866));
#2671=EDGE_LOOP('',(#10867,#10868,#10869));
#2672=EDGE_LOOP('',(#10870,#10871,#10872,#10873));
#2673=EDGE_LOOP('',(#10874));
#2674=EDGE_LOOP('',(#10875,#10876,#10877,#10878));
#2675=EDGE_LOOP('',(#10879));
#2676=EDGE_LOOP('',(#10880,#10881,#10882));
#2677=EDGE_LOOP('',(#10883,#10884,#10885,#10886));
#2678=EDGE_LOOP('',(#10887));
#2679=EDGE_LOOP('',(#10888,#10889,#10890,#10891));
#2680=EDGE_LOOP('',(#10892));
#2681=EDGE_LOOP('',(#10893,#10894,#10895,#10896));
#2682=EDGE_LOOP('',(#10897,#10898,#10899,#10900,#10901,#10902));
#2683=EDGE_LOOP('',(#10903,#10904,#10905,#10906,#10907,#10908,#10909));
#2684=EDGE_LOOP('',(#10910,#10911,#10912,#10913,#10914,#10915));
#2685=EDGE_LOOP('',(#10916,#10917,#10918,#10919,#10920,#10921));
#2686=EDGE_LOOP('',(#10922,#10923,#10924,#10925));
#2687=EDGE_LOOP('',(#10926,#10927,#10928,#10929));
#2688=EDGE_LOOP('',(#10930,#10931,#10932,#10933,#10934,#10935));
#2689=EDGE_LOOP('',(#10936,#10937,#10938,#10939,#10940,#10941));
#2690=EDGE_LOOP('',(#10942));
#2691=EDGE_LOOP('',(#10943));
#2692=EDGE_LOOP('',(#10944));
#2693=EDGE_LOOP('',(#10945,#10946,#10947,#10948));
#2694=EDGE_LOOP('',(#10949,#10950,#10951,#10952,#10953,#10954,#10955,#10956,
#10957,#10958,#10959,#10960,#10961,#10962,#10963,#10964,#10965,#10966,#10967,
#10968,#10969,#10970,#10971,#10972,#10973,#10974,#10975,#10976,#10977,#10978));
#2695=EDGE_LOOP('',(#10979,#10980,#10981,#10982));
#2696=EDGE_LOOP('',(#10983,#10984,#10985,#10986,#10987,#10988,#10989,#10990,
#10991,#10992,#10993,#10994,#10995,#10996,#10997,#10998,#10999,#11000,#11001,
#11002,#11003,#11004,#11005,#11006,#11007,#11008,#11009,#11010,#11011,#11012));
#2697=EDGE_LOOP('',(#11013,#11014,#11015,#11016,#11017,#11018,#11019));
#2698=EDGE_LOOP('',(#11020,#11021,#11022,#11023,#11024,#11025,#11026));
#2699=EDGE_LOOP('',(#11027,#11028,#11029,#11030));
#2700=EDGE_LOOP('',(#11031,#11032,#11033,#11034));
#2701=EDGE_LOOP('',(#11035,#11036,#11037,#11038));
#2702=EDGE_LOOP('',(#11039,#11040,#11041,#11042));
#2703=EDGE_LOOP('',(#11043,#11044,#11045,#11046));
#2704=EDGE_LOOP('',(#11047,#11048,#11049,#11050));
#2705=EDGE_LOOP('',(#11051,#11052,#11053,#11054));
#2706=EDGE_LOOP('',(#11055,#11056,#11057,#11058));
#2707=EDGE_LOOP('',(#11059,#11060,#11061,#11062));
#2708=EDGE_LOOP('',(#11063,#11064,#11065,#11066));
#2709=EDGE_LOOP('',(#11067,#11068,#11069,#11070,#11071,#11072,#11073,#11074));
#2710=EDGE_LOOP('',(#11075,#11076,#11077,#11078));
#2711=EDGE_LOOP('',(#11079,#11080,#11081,#11082));
#2712=EDGE_LOOP('',(#11083,#11084,#11085,#11086));
#2713=EDGE_LOOP('',(#11087,#11088,#11089,#11090));
#2714=EDGE_LOOP('',(#11091,#11092,#11093,#11094));
#2715=EDGE_LOOP('',(#11095,#11096,#11097,#11098));
#2716=EDGE_LOOP('',(#11099,#11100,#11101,#11102));
#2717=EDGE_LOOP('',(#11103,#11104,#11105,#11106));
#2718=EDGE_LOOP('',(#11107,#11108,#11109,#11110));
#2719=EDGE_LOOP('',(#11111,#11112,#11113,#11114,#11115,#11116,#11117,#11118,
#11119,#11120,#11121,#11122));
#2720=EDGE_LOOP('',(#11123,#11124,#11125,#11126));
#2721=EDGE_LOOP('',(#11127));
#2722=EDGE_LOOP('',(#11128,#11129,#11130,#11131,#11132,#11133));
#2723=EDGE_LOOP('',(#11134));
#2724=EDGE_LOOP('',(#11135));
#2725=EDGE_LOOP('',(#11136,#11137,#11138,#11139,#11140,#11141));
#2726=EDGE_LOOP('',(#11142,#11143,#11144,#11145,#11146,#11147));
#2727=EDGE_LOOP('',(#11148,#11149,#11150,#11151,#11152,#11153));
#2728=EDGE_LOOP('',(#11154,#11155,#11156,#11157,#11158,#11159));
#2729=EDGE_LOOP('',(#11160,#11161,#11162,#11163,#11164,#11165));
#2730=EDGE_LOOP('',(#11166,#11167,#11168,#11169,#11170,#11171));
#2731=EDGE_LOOP('',(#11172,#11173,#11174,#11175));
#2732=EDGE_LOOP('',(#11176,#11177,#11178,#11179));
#2733=EDGE_LOOP('',(#11180,#11181,#11182,#11183,#11184,#11185,#11186,#11187,
#11188,#11189,#11190,#11191,#11192,#11193,#11194,#11195,#11196,#11197,#11198,
#11199));
#2734=EDGE_LOOP('',(#11200,#11201,#11202,#11203,#11204,#11205,#11206,#11207,
#11208,#11209,#11210,#11211,#11212,#11213,#11214,#11215,#11216,#11217,#11218,
#11219,#11220));
#2735=EDGE_LOOP('',(#11221,#11222,#11223));
#2736=EDGE_LOOP('',(#11224,#11225,#11226));
#2737=EDGE_LOOP('',(#11227,#11228,#11229));
#2738=EDGE_LOOP('',(#11230,#11231,#11232));
#2739=EDGE_LOOP('',(#11233,#11234,#11235));
#2740=EDGE_LOOP('',(#11236,#11237,#11238));
#3433=LINE('',#23319,#4253);
#3434=LINE('',#23325,#4254);
#3435=LINE('',#23361,#4255);
#3436=LINE('',#23367,#4256);
#3437=LINE('',#23370,#4257);
#3438=LINE('',#23375,#4258);
#3439=LINE('',#23378,#4259);
#3440=LINE('',#23380,#4260);
#3441=LINE('',#23391,#4261);
#3442=LINE('',#23399,#4262);
#3443=LINE('',#23402,#4263);
#3444=LINE('',#23408,#4264);
#3445=LINE('',#23420,#4265);
#3446=LINE('',#23433,#4266);
#3447=LINE('',#23471,#4267);
#3448=LINE('',#23509,#4268);
#3449=LINE('',#23547,#4269);
#3450=LINE('',#23585,#4270);
#3451=LINE('',#23623,#4271);
#3452=LINE('',#23661,#4272);
#3453=LINE('',#23699,#4273);
#3454=LINE('',#23737,#4274);
#3455=LINE('',#23775,#4275);
#3456=LINE('',#23813,#4276);
#3457=LINE('',#23851,#4277);
#3458=LINE('',#23889,#4278);
#3459=LINE('',#23928,#4279);
#3460=LINE('',#23960,#4280);
#3461=LINE('',#23992,#4281);
#3462=LINE('',#24068,#4282);
#3463=LINE('',#24146,#4283);
#3464=LINE('',#24222,#4284);
#3465=LINE('',#24298,#4285);
#3466=LINE('',#24374,#4286);
#3467=LINE('',#24450,#4287);
#3468=LINE('',#24526,#4288);
#3469=LINE('',#24604,#4289);
#3470=LINE('',#24680,#4290);
#3471=LINE('',#24756,#4291);
#3472=LINE('',#24857,#4292);
#3473=LINE('',#24869,#4293);
#3474=LINE('',#24875,#4294);
#3475=LINE('',#24892,#4295);
#3476=LINE('',#24938,#4296);
#3477=LINE('',#24939,#4297);
#3478=LINE('',#24940,#4298);
#3479=LINE('',#24943,#4299);
#3480=LINE('',#24944,#4300);
#3481=LINE('',#24948,#4301);
#3482=LINE('',#24950,#4302);
#3483=LINE('',#24952,#4303);
#3484=LINE('',#24957,#4304);
#3485=LINE('',#24959,#4305);
#3486=LINE('',#24961,#4306);
#3487=LINE('',#24965,#4307);
#3488=LINE('',#24966,#4308);
#3489=LINE('',#24970,#4309);
#3490=LINE('',#24972,#4310);
#3491=LINE('',#24974,#4311);
#3492=LINE('',#24979,#4312);
#3493=LINE('',#24981,#4313);
#3494=LINE('',#24983,#4314);
#3495=LINE('',#24988,#4315);
#3496=LINE('',#24990,#4316);
#3497=LINE('',#24992,#4317);
#3498=LINE('',#24993,#4318);
#3499=LINE('',#24996,#4319);
#3500=LINE('',#25000,#4320);
#3501=LINE('',#25004,#4321);
#3502=LINE('',#25006,#4322);
#3503=LINE('',#25011,#4323);
#3504=LINE('',#25014,#4324);
#3505=LINE('',#25018,#4325);
#3506=LINE('',#25019,#4326);
#3507=LINE('',#25029,#4327);
#3508=LINE('',#25030,#4328);
#3509=LINE('',#25957,#4329);
#3510=LINE('',#25996,#4330);
#3511=LINE('',#26034,#4331);
#3512=LINE('',#26072,#4332);
#3513=LINE('',#26110,#4333);
#3514=LINE('',#26148,#4334);
#3515=LINE('',#26186,#4335);
#3516=LINE('',#26224,#4336);
#3517=LINE('',#26236,#4337);
#3518=LINE('',#26249,#4338);
#3519=LINE('',#26270,#4339);
#3520=LINE('',#26293,#4340);
#3521=LINE('',#26334,#4341);
#3522=LINE('',#26412,#4342);
#3523=LINE('',#26488,#4343);
#3524=LINE('',#26564,#4344);
#3525=LINE('',#26640,#4345);
#3526=LINE('',#26716,#4346);
#3527=LINE('',#26792,#4347);
#3528=LINE('',#26905,#4348);
#3529=LINE('',#26910,#4349);
#3530=LINE('',#26912,#4350);
#3531=LINE('',#26914,#4351);
#3532=LINE('',#26916,#4352);
#3533=LINE('',#26918,#4353);
#3534=LINE('',#26920,#4354);
#3535=LINE('',#26922,#4355);
#3536=LINE('',#26924,#4356);
#3537=LINE('',#26926,#4357);
#3538=LINE('',#26928,#4358);
#3539=LINE('',#26930,#4359);
#3540=LINE('',#26931,#4360);
#3541=LINE('',#26963,#4361);
#3542=LINE('',#26965,#4362);
#3543=LINE('',#26967,#4363);
#3544=LINE('',#26969,#4364);
#3545=LINE('',#26971,#4365);
#3546=LINE('',#26972,#4366);
#3547=LINE('',#26976,#4367);
#3548=LINE('',#26978,#4368);
#3549=LINE('',#26979,#4369);
#3550=LINE('',#26980,#4370);
#3551=LINE('',#26982,#4371);
#3552=LINE('',#26984,#4372);
#3553=LINE('',#26985,#4373);
#3554=LINE('',#26988,#4374);
#3555=LINE('',#26989,#4375);
#3556=LINE('',#26990,#4376);
#3557=LINE('',#26992,#4377);
#3558=LINE('',#26994,#4378);
#3559=LINE('',#26995,#4379);
#3560=LINE('',#26998,#4380);
#3561=LINE('',#26999,#4381);
#3562=LINE('',#27000,#4382);
#3563=LINE('',#27002,#4383);
#3564=LINE('',#27003,#4384);
#3565=LINE('',#27005,#4385);
#3566=LINE('',#27006,#4386);
#4253=VECTOR('',#16853,20.6);
#4254=VECTOR('',#16860,20.);
#4255=VECTOR('',#16905,5.00000000000001);
#4256=VECTOR('',#16912,7.);
#4257=VECTOR('',#16917,20.);
#4258=VECTOR('',#16922,15.);
#4259=VECTOR('',#16927,20.);
#4260=VECTOR('',#16930,25.);
#4261=VECTOR('',#16947,4.90000000000001);
#4262=VECTOR('',#16956,4.7);
#4263=VECTOR('',#16961,4.90000000000001);
#4264=VECTOR('',#16968,4.45873412499923);
#4265=VECTOR('',#16969,1000.);
#4266=VECTOR('',#16972,4.45873412499923);
#4267=VECTOR('',#16975,4.45873412499923);
#4268=VECTOR('',#16978,4.45873412499923);
#4269=VECTOR('',#16981,4.45873412499923);
#4270=VECTOR('',#16984,4.45873412499923);
#4271=VECTOR('',#16987,4.45873412499923);
#4272=VECTOR('',#16990,4.45873412499923);
#4273=VECTOR('',#16993,4.45873412499923);
#4274=VECTOR('',#16996,4.45873412499923);
#4275=VECTOR('',#16999,4.45873412499923);
#4276=VECTOR('',#17002,4.45873412499923);
#4277=VECTOR('',#17005,4.45873412499923);
#4278=VECTOR('',#17008,5.00000000000001);
#4279=VECTOR('',#17009,5.00000000000001);
#4280=VECTOR('',#17012,1000.);
#4281=VECTOR('',#17015,5.00000000000001);
#4282=VECTOR('',#17018,5.00000000000001);
#4283=VECTOR('',#17021,5.00000000000001);
#4284=VECTOR('',#17024,5.00000000000001);
#4285=VECTOR('',#17027,5.00000000000001);
#4286=VECTOR('',#17030,5.00000000000001);
#4287=VECTOR('',#17033,5.00000000000001);
#4288=VECTOR('',#17036,5.00000000000001);
#4289=VECTOR('',#17039,5.00000000000001);
#4290=VECTOR('',#17042,5.00000000000001);
#4291=VECTOR('',#17045,5.00000000000001);
#4292=VECTOR('',#17054,9.99999999999999);
#4293=VECTOR('',#17067,5.);
#4294=VECTOR('',#17074,5.);
#4295=VECTOR('',#17079,4.35000000000001);
#4296=VECTOR('',#17086,1000.);
#4297=VECTOR('',#17087,1000.);
#4298=VECTOR('',#17088,1000.);
#4299=VECTOR('',#17091,1000.);
#4300=VECTOR('',#17092,1000.);
#4301=VECTOR('',#17095,1000.);
#4302=VECTOR('',#17096,1000.);
#4303=VECTOR('',#17097,1000.);
#4304=VECTOR('',#17102,1000.);
#4305=VECTOR('',#17103,1000.);
#4306=VECTOR('',#17104,1000.);
#4307=VECTOR('',#17109,1000.);
#4308=VECTOR('',#17110,1000.);
#4309=VECTOR('',#17113,1000.);
#4310=VECTOR('',#17114,1000.);
#4311=VECTOR('',#17115,1000.);
#4312=VECTOR('',#17120,1000.);
#4313=VECTOR('',#17121,1000.);
#4314=VECTOR('',#17122,1000.);
#4315=VECTOR('',#17127,1000.);
#4316=VECTOR('',#17128,1000.);
#4317=VECTOR('',#17129,1000.);
#4318=VECTOR('',#17130,1000.);
#4319=VECTOR('',#17133,1000.);
#4320=VECTOR('',#17138,1000.);
#4321=VECTOR('',#17143,1000.);
#4322=VECTOR('',#17144,1000.);
#4323=VECTOR('',#17153,1000.);
#4324=VECTOR('',#17158,1000.);
#4325=VECTOR('',#17165,1000.);
#4326=VECTOR('',#17166,1000.);
#4327=VECTOR('',#17185,1000.);
#4328=VECTOR('',#17186,1000.);
#4329=VECTOR('',#17199,5.54126587500002);
#4330=VECTOR('',#17204,5.54126587500002);
#4331=VECTOR('',#17207,5.54126587500002);
#4332=VECTOR('',#17210,5.54126587500002);
#4333=VECTOR('',#17213,5.54126587500002);
#4334=VECTOR('',#17216,5.54126587500002);
#4335=VECTOR('',#17219,5.54126587500002);
#4336=VECTOR('',#17222,5.54126587500002);
#4337=VECTOR('',#17223,1000.);
#4338=VECTOR('',#17226,5.);
#4339=VECTOR('',#17227,1000.);
#4340=VECTOR('',#17228,5.);
#4341=VECTOR('',#17233,5.);
#4342=VECTOR('',#17236,5.);
#4343=VECTOR('',#17239,5.);
#4344=VECTOR('',#17242,5.);
#4345=VECTOR('',#17245,5.);
#4346=VECTOR('',#17248,5.);
#4347=VECTOR('',#17251,5.);
#4348=VECTOR('',#17260,9.99999999999999);
#4349=VECTOR('',#17265,1000.);
#4350=VECTOR('',#17266,1000.);
#4351=VECTOR('',#17267,1000.);
#4352=VECTOR('',#17268,1000.);
#4353=VECTOR('',#17269,1000.);
#4354=VECTOR('',#17270,1000.);
#4355=VECTOR('',#17271,1000.);
#4356=VECTOR('',#17272,1000.);
#4357=VECTOR('',#17273,1000.);
#4358=VECTOR('',#17274,1000.);
#4359=VECTOR('',#17275,1000.);
#4360=VECTOR('',#17276,1000.);
#4361=VECTOR('',#17279,1000.);
#4362=VECTOR('',#17280,1000.);
#4363=VECTOR('',#17281,1000.);
#4364=VECTOR('',#17282,1000.);
#4365=VECTOR('',#17283,1000.);
#4366=VECTOR('',#17284,1000.);
#4367=VECTOR('',#17289,1000.);
#4368=VECTOR('',#17290,1000.);
#4369=VECTOR('',#17291,1000.);
#4370=VECTOR('',#17292,1000.);
#4371=VECTOR('',#17295,1000.);
#4372=VECTOR('',#17296,1000.);
#4373=VECTOR('',#17297,1000.);
#4374=VECTOR('',#17300,1000.);
#4375=VECTOR('',#17301,1000.);
#4376=VECTOR('',#17302,1000.);
#4377=VECTOR('',#17305,1000.);
#4378=VECTOR('',#17306,1000.);
#4379=VECTOR('',#17307,1000.);
#4380=VECTOR('',#17310,1000.);
#4381=VECTOR('',#17311,1000.);
#4382=VECTOR('',#17312,1000.);
#4383=VECTOR('',#17315,1000.);
#4384=VECTOR('',#17316,1000.);
#4385=VECTOR('',#17319,1000.);
#4386=VECTOR('',#17320,1000.);
#4966=CIRCLE('',#13517,20.);
#4967=CIRCLE('',#13518,20.);
#4968=CIRCLE('',#13519,20.6);
#4969=CIRCLE('',#13521,20.);
#4970=CIRCLE('',#13522,20.6);
#4971=CIRCLE('',#13524,23.);
#4972=CIRCLE('',#13525,2.);
#4973=CIRCLE('',#13526,25.);
#4974=CIRCLE('',#13527,25.);
#4975=CIRCLE('',#13529,18.);
#4976=CIRCLE('',#13530,2.);
#4977=CIRCLE('',#13531,20.);
#4978=CIRCLE('',#13533,25.);
#4979=CIRCLE('',#13534,25.);
#4980=CIRCLE('',#13535,2.);
#4981=CIRCLE('',#13536,23.);
#4982=CIRCLE('',#13538,18.);
#4983=CIRCLE('',#13539,2.);
#4984=CIRCLE('',#13540,20.);
#4985=CIRCLE('',#13541,20.);
#4986=CIRCLE('',#13543,5.00000000000001);
#4987=CIRCLE('',#13544,5.00000000000001);
#4988=CIRCLE('',#13546,15.);
#4989=CIRCLE('',#13547,7.);
#4990=CIRCLE('',#13550,15.);
#4991=CIRCLE('',#13551,7.);
#4992=CIRCLE('',#13561,4.90000000000001);
#4993=CIRCLE('',#13562,4.70000000000039);
#4994=CIRCLE('',#13564,4.90000000000002);
#4995=CIRCLE('',#13565,4.90000000000002);
#4996=CIRCLE('',#13566,4.70000000000003);
#4997=CIRCLE('',#13584,5.00000000000001);
#4998=CIRCLE('',#13597,5.00000000000001);
#4999=CIRCLE('',#13599,9.99999999999999);
#5000=CIRCLE('',#13600,10.);
#5001=CIRCLE('',#13601,10.);
#5002=CIRCLE('',#13602,10.);
#5003=CIRCLE('',#13603,10.);
#5004=CIRCLE('',#13605,5.);
#5005=CIRCLE('',#13606,5.);
#5006=CIRCLE('',#13608,5.);
#5007=CIRCLE('',#13609,5.);
#5008=CIRCLE('',#13611,4.35000000000001);
#5009=CIRCLE('',#13612,4.45873412500005);
#5010=CIRCLE('',#13616,9.);
#5011=CIRCLE('',#13618,9.);
#5012=CIRCLE('',#13621,9.);
#5013=CIRCLE('',#13623,9.);
#5014=CIRCLE('',#13626,4.99999999999998);
#5015=CIRCLE('',#13627,4.99999999999998);
#5016=CIRCLE('',#13629,4.99999999999998);
#5017=CIRCLE('',#13630,4.99999999999998);
#5018=CIRCLE('',#13654,5.5412658750012);
#5019=CIRCLE('',#13663,5.);
#5020=CIRCLE('',#13671,5.);
#5021=CIRCLE('',#13674,9.99999999999999);
#5022=CIRCLE('',#13675,9.99999999999999);
#5932=VERTEX_POINT('',#23314);
#5933=VERTEX_POINT('',#23315);
#5934=VERTEX_POINT('',#23318);
#5935=VERTEX_POINT('',#23322);
#5936=VERTEX_POINT('',#23324);
#5937=VERTEX_POINT('',#23328);
#5938=VERTEX_POINT('',#23330);
#5939=VERTEX_POINT('',#23332);
#5940=VERTEX_POINT('',#23336);
#5941=VERTEX_POINT('',#23338);
#5942=VERTEX_POINT('',#23342);
#5943=VERTEX_POINT('',#23343);
#5944=VERTEX_POINT('',#23346);
#5945=VERTEX_POINT('',#23350);
#5946=VERTEX_POINT('',#23352);
#5947=VERTEX_POINT('',#23354);
#5948=VERTEX_POINT('',#23358);
#5949=VERTEX_POINT('',#23360);
#5950=VERTEX_POINT('',#23364);
#5951=VERTEX_POINT('',#23366);
#5952=VERTEX_POINT('',#23372);
#5953=VERTEX_POINT('',#23374);
#5954=VERTEX_POINT('',#23388);
#5955=VERTEX_POINT('',#23390);
#5956=VERTEX_POINT('',#23394);
#5957=VERTEX_POINT('',#23395);
#5958=VERTEX_POINT('',#23398);
#5959=VERTEX_POINT('',#23406);
#5960=VERTEX_POINT('',#23407);
#5961=VERTEX_POINT('',#23409);
#5962=VERTEX_POINT('',#23419);
#5963=VERTEX_POINT('',#23431);
#5964=VERTEX_POINT('',#23432);
#5965=VERTEX_POINT('',#23469);
#5966=VERTEX_POINT('',#23470);
#5967=VERTEX_POINT('',#23507);
#5968=VERTEX_POINT('',#23508);
#5969=VERTEX_POINT('',#23545);
#5970=VERTEX_POINT('',#23546);
#5971=VERTEX_POINT('',#23583);
#5972=VERTEX_POINT('',#23584);
#5973=VERTEX_POINT('',#23621);
#5974=VERTEX_POINT('',#23622);
#5975=VERTEX_POINT('',#23659);
#5976=VERTEX_POINT('',#23660);
#5977=VERTEX_POINT('',#23697);
#5978=VERTEX_POINT('',#23698);
#5979=VERTEX_POINT('',#23735);
#5980=VERTEX_POINT('',#23736);
#5981=VERTEX_POINT('',#23773);
#5982=VERTEX_POINT('',#23774);
#5983=VERTEX_POINT('',#23811);
#5984=VERTEX_POINT('',#23812);
#5985=VERTEX_POINT('',#23849);
#5986=VERTEX_POINT('',#23850);
#5987=VERTEX_POINT('',#23887);
#5988=VERTEX_POINT('',#23888);
#5989=VERTEX_POINT('',#23890);
#5990=VERTEX_POINT('',#23927);
#5991=VERTEX_POINT('',#23930);
#5992=VERTEX_POINT('',#23959);
#5993=VERTEX_POINT('',#23990);
#5994=VERTEX_POINT('',#23991);
#5995=VERTEX_POINT('',#24066);
#5996=VERTEX_POINT('',#24067);
#5997=VERTEX_POINT('',#24144);
#5998=VERTEX_POINT('',#24145);
#5999=VERTEX_POINT('',#24220);
#6000=VERTEX_POINT('',#24221);
#6001=VERTEX_POINT('',#24296);
#6002=VERTEX_POINT('',#24297);
#6003=VERTEX_POINT('',#24372);
#6004=VERTEX_POINT('',#24373);
#6005=VERTEX_POINT('',#24448);
#6006=VERTEX_POINT('',#24449);
#6007=VERTEX_POINT('',#24524);
#6008=VERTEX_POINT('',#24525);
#6009=VERTEX_POINT('',#24602);
#6010=VERTEX_POINT('',#24603);
#6011=VERTEX_POINT('',#24678);
#6012=VERTEX_POINT('',#24679);
#6013=VERTEX_POINT('',#24754);
#6014=VERTEX_POINT('',#24755);
#6015=VERTEX_POINT('',#24830);
#6016=VERTEX_POINT('',#24843);
#6017=VERTEX_POINT('',#24854);
#6018=VERTEX_POINT('',#24856);
#6019=VERTEX_POINT('',#24858);
#6020=VERTEX_POINT('',#24860);
#6021=VERTEX_POINT('',#24862);
#6022=VERTEX_POINT('',#24866);
#6023=VERTEX_POINT('',#24868);
#6024=VERTEX_POINT('',#24872);
#6025=VERTEX_POINT('',#24874);
#6026=VERTEX_POINT('',#24878);
#6027=VERTEX_POINT('',#24891);
#6028=VERTEX_POINT('',#24894);
#6029=VERTEX_POINT('',#24921);
#6030=VERTEX_POINT('',#24936);
#6031=VERTEX_POINT('',#24937);
#6032=VERTEX_POINT('',#24942);
#6033=VERTEX_POINT('',#24946);
#6034=VERTEX_POINT('',#24947);
#6035=VERTEX_POINT('',#24949);
#6036=VERTEX_POINT('',#24951);
#6037=VERTEX_POINT('',#24955);
#6038=VERTEX_POINT('',#24956);
#6039=VERTEX_POINT('',#24958);
#6040=VERTEX_POINT('',#24960);
#6041=VERTEX_POINT('',#24964);
#6042=VERTEX_POINT('',#24968);
#6043=VERTEX_POINT('',#24969);
#6044=VERTEX_POINT('',#24971);
#6045=VERTEX_POINT('',#24973);
#6046=VERTEX_POINT('',#24977);
#6047=VERTEX_POINT('',#24978);
#6048=VERTEX_POINT('',#24980);
#6049=VERTEX_POINT('',#24982);
#6050=VERTEX_POINT('',#24986);
#6051=VERTEX_POINT('',#24987);
#6052=VERTEX_POINT('',#24989);
#6053=VERTEX_POINT('',#24991);
#6054=VERTEX_POINT('',#24995);
#6055=VERTEX_POINT('',#24998);
#6056=VERTEX_POINT('',#25002);
#6057=VERTEX_POINT('',#25005);
#6058=VERTEX_POINT('',#25955);
#6059=VERTEX_POINT('',#25956);
#6060=VERTEX_POINT('',#25958);
#6061=VERTEX_POINT('',#25974);
#6062=VERTEX_POINT('',#25994);
#6063=VERTEX_POINT('',#25995);
#6064=VERTEX_POINT('',#26032);
#6065=VERTEX_POINT('',#26033);
#6066=VERTEX_POINT('',#26070);
#6067=VERTEX_POINT('',#26071);
#6068=VERTEX_POINT('',#26108);
#6069=VERTEX_POINT('',#26109);
#6070=VERTEX_POINT('',#26146);
#6071=VERTEX_POINT('',#26147);
#6072=VERTEX_POINT('',#26184);
#6073=VERTEX_POINT('',#26185);
#6074=VERTEX_POINT('',#26222);
#6075=VERTEX_POINT('',#26223);
#6076=VERTEX_POINT('',#26225);
#6077=VERTEX_POINT('',#26235);
#6078=VERTEX_POINT('',#26247);
#6079=VERTEX_POINT('',#26248);
#6080=VERTEX_POINT('',#26250);
#6081=VERTEX_POINT('',#26269);
#6082=VERTEX_POINT('',#26271);
#6083=VERTEX_POINT('',#26292);
#6084=VERTEX_POINT('',#26332);
#6085=VERTEX_POINT('',#26333);
#6086=VERTEX_POINT('',#26410);
#6087=VERTEX_POINT('',#26411);
#6088=VERTEX_POINT('',#26486);
#6089=VERTEX_POINT('',#26487);
#6090=VERTEX_POINT('',#26562);
#6091=VERTEX_POINT('',#26563);
#6092=VERTEX_POINT('',#26638);
#6093=VERTEX_POINT('',#26639);
#6094=VERTEX_POINT('',#26714);
#6095=VERTEX_POINT('',#26715);
#6096=VERTEX_POINT('',#26790);
#6097=VERTEX_POINT('',#26791);
#6098=VERTEX_POINT('',#26793);
#6099=VERTEX_POINT('',#26806);
#6100=VERTEX_POINT('',#26902);
#6101=VERTEX_POINT('',#26904);
#6102=VERTEX_POINT('',#26908);
#6103=VERTEX_POINT('',#26909);
#6104=VERTEX_POINT('',#26911);
#6105=VERTEX_POINT('',#26913);
#6106=VERTEX_POINT('',#26915);
#6107=VERTEX_POINT('',#26917);
#6108=VERTEX_POINT('',#26919);
#6109=VERTEX_POINT('',#26921);
#6110=VERTEX_POINT('',#26923);
#6111=VERTEX_POINT('',#26925);
#6112=VERTEX_POINT('',#26927);
#6113=VERTEX_POINT('',#26929);
#6114=VERTEX_POINT('',#26961);
#6115=VERTEX_POINT('',#26962);
#6116=VERTEX_POINT('',#26964);
#6117=VERTEX_POINT('',#26966);
#6118=VERTEX_POINT('',#26968);
#6119=VERTEX_POINT('',#26970);
#6120=VERTEX_POINT('',#26975);
#6121=VERTEX_POINT('',#26977);
#6122=VERTEX_POINT('',#26983);
#6123=VERTEX_POINT('',#26987);
#6124=VERTEX_POINT('',#26993);
#6125=VERTEX_POINT('',#26997);
#7536=EDGE_CURVE('',#5932,#5933,#4966,.T.);
#7537=EDGE_CURVE('',#5933,#5932,#4967,.T.);
#7538=EDGE_CURVE('',#5933,#5934,#3433,.T.);
#7539=EDGE_CURVE('',#5934,#5934,#4968,.T.);
#7540=EDGE_CURVE('',#5935,#5935,#4969,.T.);
#7541=EDGE_CURVE('',#5935,#5936,#3434,.T.);
#7542=EDGE_CURVE('',#5936,#5936,#4970,.T.);
#7543=EDGE_CURVE('',#5937,#5937,#4971,.T.);
#7544=EDGE_CURVE('',#5937,#5938,#4972,.T.);
#7545=EDGE_CURVE('',#5939,#5938,#4973,.T.);
#7546=EDGE_CURVE('',#5938,#5939,#4974,.T.);
#7547=EDGE_CURVE('',#5940,#5940,#4975,.T.);
#7548=EDGE_CURVE('',#5940,#5941,#4976,.T.);
#7549=EDGE_CURVE('',#5941,#5941,#4977,.T.);
#7550=EDGE_CURVE('',#5942,#5943,#4978,.T.);
#7551=EDGE_CURVE('',#5943,#5942,#4979,.T.);
#7552=EDGE_CURVE('',#5943,#5944,#4980,.T.);
#7553=EDGE_CURVE('',#5944,#5944,#4981,.T.);
#7554=EDGE_CURVE('',#5945,#5945,#4982,.T.);
#7555=EDGE_CURVE('',#5945,#5946,#4983,.T.);
#7556=EDGE_CURVE('',#5947,#5946,#4984,.T.);
#7557=EDGE_CURVE('',#5946,#5947,#4985,.T.);
#7558=EDGE_CURVE('',#5948,#5948,#4986,.T.);
#7559=EDGE_CURVE('',#5948,#5949,#3435,.T.);
#7560=EDGE_CURVE('',#5949,#5949,#4987,.T.);
#7561=EDGE_CURVE('',#5950,#5950,#4988,.T.);
#7562=EDGE_CURVE('',#5950,#5951,#3436,.T.);
#7563=EDGE_CURVE('',#5951,#5951,#4989,.T.);
#7564=EDGE_CURVE('',#5941,#5935,#3437,.T.);
#7565=EDGE_CURVE('',#5952,#5952,#4990,.T.);
#7566=EDGE_CURVE('',#5952,#5953,#3438,.T.);
#7567=EDGE_CURVE('',#5953,#5953,#4991,.T.);
#7568=EDGE_CURVE('',#5932,#5947,#3439,.T.);
#7569=EDGE_CURVE('',#5942,#5939,#3440,.T.);
#7570=EDGE_CURVE('',#5954,#5954,#4992,.T.);
#7571=EDGE_CURVE('',#5954,#5955,#3441,.T.);
#7572=EDGE_CURVE('',#5955,#5955,#4993,.T.);
#7573=EDGE_CURVE('',#5956,#5957,#4994,.T.);
#7574=EDGE_CURVE('',#5957,#5956,#4995,.T.);
#7575=EDGE_CURVE('',#5957,#5958,#3442,.T.);
#7576=EDGE_CURVE('',#5958,#5958,#4996,.T.);
#7577=EDGE_CURVE('',#5956,#5954,#3443,.T.);
#7578=EDGE_CURVE('',#5959,#5960,#3444,.T.);
#7579=EDGE_CURVE('',#5959,#5961,#36,.T.);
#7580=EDGE_CURVE('',#5961,#5962,#3445,.T.);
#7581=EDGE_CURVE('',#5960,#5962,#37,.T.);
#7582=EDGE_CURVE('',#5963,#5964,#3446,.T.);
#7583=EDGE_CURVE('',#5963,#5959,#38,.T.);
#7584=EDGE_CURVE('',#5964,#5960,#39,.T.);
#7585=EDGE_CURVE('',#5965,#5966,#3447,.T.);
#7586=EDGE_CURVE('',#5965,#5963,#40,.T.);
#7587=EDGE_CURVE('',#5966,#5964,#41,.T.);
#7588=EDGE_CURVE('',#5967,#5968,#3448,.T.);
#7589=EDGE_CURVE('',#5967,#5965,#42,.T.);
#7590=EDGE_CURVE('',#5968,#5966,#43,.T.);
#7591=EDGE_CURVE('',#5969,#5970,#3449,.T.);
#7592=EDGE_CURVE('',#5969,#5967,#44,.T.);
#7593=EDGE_CURVE('',#5970,#5968,#45,.T.);
#7594=EDGE_CURVE('',#5971,#5972,#3450,.T.);
#7595=EDGE_CURVE('',#5971,#5969,#46,.T.);
#7596=EDGE_CURVE('',#5972,#5970,#47,.T.);
#7597=EDGE_CURVE('',#5973,#5974,#3451,.T.);
#7598=EDGE_CURVE('',#5973,#5971,#48,.T.);
#7599=EDGE_CURVE('',#5974,#5972,#49,.T.);
#7600=EDGE_CURVE('',#5975,#5976,#3452,.T.);
#7601=EDGE_CURVE('',#5975,#5973,#50,.T.);
#7602=EDGE_CURVE('',#5976,#5974,#51,.T.);
#7603=EDGE_CURVE('',#5977,#5978,#3453,.T.);
#7604=EDGE_CURVE('',#5977,#5975,#52,.T.);
#7605=EDGE_CURVE('',#5978,#5976,#53,.T.);
#7606=EDGE_CURVE('',#5979,#5980,#3454,.T.);
#7607=EDGE_CURVE('',#5979,#5977,#54,.T.);
#7608=EDGE_CURVE('',#5980,#5978,#55,.T.);
#7609=EDGE_CURVE('',#5981,#5982,#3455,.T.);
#7610=EDGE_CURVE('',#5981,#5979,#56,.T.);
#7611=EDGE_CURVE('',#5982,#5980,#57,.T.);
#7612=EDGE_CURVE('',#5983,#5984,#3456,.T.);
#7613=EDGE_CURVE('',#5983,#5981,#58,.T.);
#7614=EDGE_CURVE('',#5984,#5982,#59,.T.);
#7615=EDGE_CURVE('',#5985,#5986,#3457,.T.);
#7616=EDGE_CURVE('',#5985,#5983,#60,.T.);
#7617=EDGE_CURVE('',#5986,#5984,#61,.T.);
#7618=EDGE_CURVE('',#5987,#5988,#3458,.T.);
#7619=EDGE_CURVE('',#5987,#5989,#924,.T.);
#7620=EDGE_CURVE('',#5989,#5990,#3459,.T.);
#7621=EDGE_CURVE('',#5990,#5990,#4997,.T.);
#7622=EDGE_CURVE('',#5989,#5991,#925,.T.);
#7623=EDGE_CURVE('',#5991,#5992,#3460,.T.);
#7624=EDGE_CURVE('',#5988,#5992,#926,.F.);
#7625=EDGE_CURVE('',#5993,#5994,#3461,.T.);
#7626=EDGE_CURVE('',#5993,#5987,#927,.T.);
#7627=EDGE_CURVE('',#5994,#5988,#928,.F.);
#7628=EDGE_CURVE('',#5995,#5996,#3462,.T.);
#7629=EDGE_CURVE('',#5995,#5993,#929,.T.);
#7630=EDGE_CURVE('',#5996,#5994,#930,.F.);
#7631=EDGE_CURVE('',#5997,#5998,#3463,.T.);
#7632=EDGE_CURVE('',#5997,#5995,#931,.T.);
#7633=EDGE_CURVE('',#5998,#5996,#932,.F.);
#7634=EDGE_CURVE('',#5999,#6000,#3464,.T.);
#7635=EDGE_CURVE('',#5999,#5997,#933,.T.);
#7636=EDGE_CURVE('',#6000,#5998,#934,.F.);
#7637=EDGE_CURVE('',#6001,#6002,#3465,.T.);
#7638=EDGE_CURVE('',#6001,#5999,#935,.T.);
#7639=EDGE_CURVE('',#6002,#6000,#936,.F.);
#7640=EDGE_CURVE('',#6003,#6004,#3466,.T.);
#7641=EDGE_CURVE('',#6003,#6001,#937,.T.);
#7642=EDGE_CURVE('',#6004,#6002,#938,.F.);
#7643=EDGE_CURVE('',#6005,#6006,#3467,.T.);
#7644=EDGE_CURVE('',#6005,#6003,#939,.T.);
#7645=EDGE_CURVE('',#6006,#6004,#940,.F.);
#7646=EDGE_CURVE('',#6007,#6008,#3468,.T.);
#7647=EDGE_CURVE('',#6007,#6005,#941,.T.);
#7648=EDGE_CURVE('',#6008,#6006,#942,.F.);
#7649=EDGE_CURVE('',#6009,#6010,#3469,.T.);
#7650=EDGE_CURVE('',#6009,#6007,#943,.T.);
#7651=EDGE_CURVE('',#6010,#6008,#944,.F.);
#7652=EDGE_CURVE('',#6011,#6012,#3470,.T.);
#7653=EDGE_CURVE('',#6011,#6009,#945,.T.);
#7654=EDGE_CURVE('',#6012,#6010,#946,.F.);
#7655=EDGE_CURVE('',#6013,#6014,#3471,.T.);
#7656=EDGE_CURVE('',#6013,#6011,#947,.T.);
#7657=EDGE_CURVE('',#6014,#6012,#948,.F.);
#7658=EDGE_CURVE('',#6015,#6014,#949,.F.);
#7659=EDGE_CURVE('',#6015,#6016,#4998,.T.);
#7660=EDGE_CURVE('',#6016,#6013,#950,.T.);
#7661=EDGE_CURVE('',#6017,#6017,#4999,.T.);
#7662=EDGE_CURVE('',#6017,#6018,#3472,.T.);
#7663=EDGE_CURVE('',#6018,#6019,#5000,.T.);
#7664=EDGE_CURVE('',#6019,#6020,#5001,.T.);
#7665=EDGE_CURVE('',#6020,#6021,#5002,.T.);
#7666=EDGE_CURVE('',#6021,#6018,#5003,.T.);
#7667=EDGE_CURVE('',#6022,#6022,#5004,.T.);
#7668=EDGE_CURVE('',#6022,#6023,#3473,.T.);
#7669=EDGE_CURVE('',#6023,#6023,#5005,.T.);
#7670=EDGE_CURVE('',#6024,#6024,#5006,.T.);
#7671=EDGE_CURVE('',#6024,#6025,#3474,.T.);
#7672=EDGE_CURVE('',#6025,#6025,#5007,.T.);
#7673=EDGE_CURVE('',#6015,#6026,#951,.T.);
#7674=EDGE_CURVE('',#6026,#6027,#3475,.T.);
#7675=EDGE_CURVE('',#6027,#6027,#5008,.T.);
#7676=EDGE_CURVE('',#6026,#6028,#952,.T.);
#7677=EDGE_CURVE('',#6028,#6029,#5009,.T.);
#7678=EDGE_CURVE('',#6029,#6016,#953,.T.);
#7679=EDGE_CURVE('',#6030,#6031,#3476,.T.);
#7680=EDGE_CURVE('',#6031,#6019,#3477,.T.);
#7681=EDGE_CURVE('',#6021,#6030,#3478,.T.);
#7682=EDGE_CURVE('',#6032,#6020,#3479,.T.);
#7683=EDGE_CURVE('',#6032,#6021,#3480,.T.);
#7684=EDGE_CURVE('',#6033,#6034,#3481,.T.);
#7685=EDGE_CURVE('',#6033,#6035,#3482,.T.);
#7686=EDGE_CURVE('',#6036,#6035,#3483,.T.);
#7687=EDGE_CURVE('',#6034,#6036,#5010,.T.);
#7688=EDGE_CURVE('',#6037,#6038,#3484,.T.);
#7689=EDGE_CURVE('',#6038,#6039,#3485,.T.);
#7690=EDGE_CURVE('',#6039,#6040,#3486,.T.);
#7691=EDGE_CURVE('',#6040,#6037,#5011,.T.);
#7692=EDGE_CURVE('',#6019,#6041,#3487,.T.);
#7693=EDGE_CURVE('',#6020,#6041,#3488,.T.);
#7694=EDGE_CURVE('',#6042,#6043,#3489,.T.);
#7695=EDGE_CURVE('',#6042,#6044,#3490,.T.);
#7696=EDGE_CURVE('',#6045,#6044,#3491,.T.);
#7697=EDGE_CURVE('',#6043,#6045,#5012,.T.);
#7698=EDGE_CURVE('',#6046,#6047,#3492,.T.);
#7699=EDGE_CURVE('',#6046,#6048,#3493,.T.);
#7700=EDGE_CURVE('',#6049,#6048,#3494,.T.);
#7701=EDGE_CURVE('',#6047,#6049,#5013,.T.);
#7702=EDGE_CURVE('',#6050,#6051,#3495,.T.);
#7703=EDGE_CURVE('',#6051,#6052,#3496,.T.);
#7704=EDGE_CURVE('',#6053,#6052,#3497,.T.);
#7705=EDGE_CURVE('',#6053,#6050,#3498,.T.);
#7706=EDGE_CURVE('',#6054,#6050,#3499,.T.);
#7707=EDGE_CURVE('',#6054,#6031,#5014,.T.);
#7708=EDGE_CURVE('',#6030,#6055,#5015,.T.);
#7709=EDGE_CURVE('',#6051,#6055,#3500,.T.);
#7710=EDGE_CURVE('',#6041,#6056,#5016,.T.);
#7711=EDGE_CURVE('',#6056,#6053,#3501,.T.);
#7712=EDGE_CURVE('',#6052,#6057,#3502,.T.);
#7713=EDGE_CURVE('',#6057,#6032,#5017,.T.);
#7714=EDGE_CURVE('',#6044,#6057,#803,.T.);
#7715=EDGE_CURVE('',#6052,#6046,#804,.T.);
#7716=EDGE_CURVE('',#6047,#6045,#3503,.T.);
#7717=EDGE_CURVE('',#6055,#6042,#805,.T.);
#7718=EDGE_CURVE('',#6049,#6043,#3504,.T.);
#7719=EDGE_CURVE('',#6048,#6051,#806,.T.);
#7720=EDGE_CURVE('',#6037,#6036,#3505,.T.);
#7721=EDGE_CURVE('',#6040,#6034,#3506,.T.);
#7722=EDGE_CURVE('',#6039,#6054,#807,.T.);
#7723=EDGE_CURVE('',#6050,#6033,#808,.T.);
#7724=EDGE_CURVE('',#6056,#6038,#809,.T.);
#7725=EDGE_CURVE('',#6035,#6053,#810,.T.);
#7726=EDGE_CURVE('',#5992,#5961,#3507,.T.);
#7727=EDGE_CURVE('',#5962,#5991,#3508,.T.);
#7728=EDGE_CURVE('',#6028,#5985,#62,.T.);
#7729=EDGE_CURVE('',#6029,#5986,#63,.T.);
#7730=EDGE_CURVE('',#6058,#6059,#3509,.T.);
#7731=EDGE_CURVE('',#6060,#6059,#64,.T.);
#7732=EDGE_CURVE('',#6061,#6060,#5018,.T.);
#7733=EDGE_CURVE('',#6061,#6058,#65,.T.);
#7734=EDGE_CURVE('',#6062,#6063,#3510,.T.);
#7735=EDGE_CURVE('',#6059,#6063,#66,.T.);
#7736=EDGE_CURVE('',#6058,#6062,#67,.T.);
#7737=EDGE_CURVE('',#6064,#6065,#3511,.T.);
#7738=EDGE_CURVE('',#6063,#6065,#68,.T.);
#7739=EDGE_CURVE('',#6062,#6064,#69,.T.);
#7740=EDGE_CURVE('',#6066,#6067,#3512,.T.);
#7741=EDGE_CURVE('',#6065,#6067,#70,.T.);
#7742=EDGE_CURVE('',#6064,#6066,#71,.T.);
#7743=EDGE_CURVE('',#6068,#6069,#3513,.T.);
#7744=EDGE_CURVE('',#6067,#6069,#72,.T.);
#7745=EDGE_CURVE('',#6066,#6068,#73,.T.);
#7746=EDGE_CURVE('',#6070,#6071,#3514,.T.);
#7747=EDGE_CURVE('',#6069,#6071,#74,.T.);
#7748=EDGE_CURVE('',#6068,#6070,#75,.T.);
#7749=EDGE_CURVE('',#6072,#6073,#3515,.T.);
#7750=EDGE_CURVE('',#6071,#6073,#76,.T.);
#7751=EDGE_CURVE('',#6070,#6072,#77,.T.);
#7752=EDGE_CURVE('',#6074,#6075,#3516,.T.);
#7753=EDGE_CURVE('',#6074,#6076,#78,.T.);
#7754=EDGE_CURVE('',#6076,#6077,#3517,.T.);
#7755=EDGE_CURVE('',#6075,#6077,#79,.T.);
#7756=EDGE_CURVE('',#6078,#6079,#3518,.T.);
#7757=EDGE_CURVE('',#6079,#6080,#954,.T.);
#7758=EDGE_CURVE('',#6080,#6081,#3519,.T.);
#7759=EDGE_CURVE('',#6082,#6081,#955,.F.);
#7760=EDGE_CURVE('',#6082,#6083,#3520,.T.);
#7761=EDGE_CURVE('',#6083,#6083,#5019,.T.);
#7762=EDGE_CURVE('',#6078,#6082,#956,.F.);
#7763=EDGE_CURVE('',#6084,#6085,#3521,.T.);
#7764=EDGE_CURVE('',#6085,#6079,#957,.T.);
#7765=EDGE_CURVE('',#6084,#6078,#958,.F.);
#7766=EDGE_CURVE('',#6086,#6087,#3522,.T.);
#7767=EDGE_CURVE('',#6087,#6085,#959,.T.);
#7768=EDGE_CURVE('',#6086,#6084,#960,.F.);
#7769=EDGE_CURVE('',#6088,#6089,#3523,.T.);
#7770=EDGE_CURVE('',#6089,#6087,#961,.T.);
#7771=EDGE_CURVE('',#6088,#6086,#962,.F.);
#7772=EDGE_CURVE('',#6090,#6091,#3524,.T.);
#7773=EDGE_CURVE('',#6091,#6089,#963,.T.);
#7774=EDGE_CURVE('',#6090,#6088,#964,.F.);
#7775=EDGE_CURVE('',#6092,#6093,#3525,.T.);
#7776=EDGE_CURVE('',#6093,#6091,#965,.T.);
#7777=EDGE_CURVE('',#6092,#6090,#966,.F.);
#7778=EDGE_CURVE('',#6094,#6095,#3526,.T.);
#7779=EDGE_CURVE('',#6095,#6093,#967,.T.);
#7780=EDGE_CURVE('',#6094,#6092,#968,.F.);
#7781=EDGE_CURVE('',#6096,#6097,#3527,.T.);
#7782=EDGE_CURVE('',#6098,#6096,#969,.F.);
#7783=EDGE_CURVE('',#6098,#6099,#5020,.T.);
#7784=EDGE_CURVE('',#6099,#6097,#970,.T.);
#7785=EDGE_CURVE('',#6097,#6095,#971,.T.);
#7786=EDGE_CURVE('',#6096,#6094,#972,.F.);
#7787=EDGE_CURVE('',#6100,#6100,#5021,.T.);
#7788=EDGE_CURVE('',#6100,#6101,#3528,.T.);
#7789=EDGE_CURVE('',#6101,#6101,#5022,.T.);
#7790=EDGE_CURVE('',#6102,#6103,#3529,.T.);
#7791=EDGE_CURVE('',#6103,#6104,#3530,.T.);
#7792=EDGE_CURVE('',#6104,#6105,#3531,.T.);
#7793=EDGE_CURVE('',#6105,#6106,#3532,.T.);
#7794=EDGE_CURVE('',#6106,#6107,#3533,.T.);
#7795=EDGE_CURVE('',#6107,#6108,#3534,.T.);
#7796=EDGE_CURVE('',#6108,#6109,#3535,.T.);
#7797=EDGE_CURVE('',#6109,#6110,#3536,.T.);
#7798=EDGE_CURVE('',#6110,#6111,#3537,.T.);
#7799=EDGE_CURVE('',#6111,#6112,#3538,.T.);
#7800=EDGE_CURVE('',#6112,#6113,#3539,.T.);
#7801=EDGE_CURVE('',#6113,#6102,#3540,.T.);
#7802=EDGE_CURVE('',#6060,#6099,#973,.T.);
#7803=EDGE_CURVE('',#6098,#6061,#974,.T.);
#7804=EDGE_CURVE('',#6114,#6115,#3541,.T.);
#7805=EDGE_CURVE('',#6116,#6114,#3542,.T.);
#7806=EDGE_CURVE('',#6117,#6116,#3543,.T.);
#7807=EDGE_CURVE('',#6118,#6117,#3544,.T.);
#7808=EDGE_CURVE('',#6119,#6118,#3545,.T.);
#7809=EDGE_CURVE('',#6115,#6119,#3546,.T.);
#7810=EDGE_CURVE('',#6103,#6120,#3547,.T.);
#7811=EDGE_CURVE('',#6121,#6102,#3548,.T.);
#7812=EDGE_CURVE('',#6121,#6114,#3549,.T.);
#7813=EDGE_CURVE('',#6120,#6115,#3550,.T.);
#7814=EDGE_CURVE('',#6120,#6104,#3551,.T.);
#7815=EDGE_CURVE('',#6122,#6119,#3552,.T.);
#7816=EDGE_CURVE('',#6105,#6122,#3553,.T.);
#7817=EDGE_CURVE('',#6107,#6123,#3554,.T.);
#7818=EDGE_CURVE('',#6122,#6106,#3555,.T.);
#7819=EDGE_CURVE('',#6123,#6118,#3556,.T.);
#7820=EDGE_CURVE('',#6123,#6108,#3557,.T.);
#7821=EDGE_CURVE('',#6124,#6117,#3558,.T.);
#7822=EDGE_CURVE('',#6109,#6124,#3559,.T.);
#7823=EDGE_CURVE('',#6111,#6125,#3560,.T.);
#7824=EDGE_CURVE('',#6124,#6110,#3561,.T.);
#7825=EDGE_CURVE('',#6125,#6116,#3562,.T.);
#7826=EDGE_CURVE('',#6113,#6121,#3563,.T.);
#7827=EDGE_CURVE('',#6125,#6112,#3564,.T.);
#7828=EDGE_CURVE('',#6081,#6076,#3565,.T.);
#7829=EDGE_CURVE('',#6077,#6080,#3566,.T.);
#7830=EDGE_CURVE('',#6073,#6075,#80,.T.);
#7831=EDGE_CURVE('',#6072,#6074,#81,.T.);
#10647=ORIENTED_EDGE('',*,*,#7536,.F.);
#10648=ORIENTED_EDGE('',*,*,#7537,.F.);
#10649=ORIENTED_EDGE('',*,*,#7538,.T.);
#10650=ORIENTED_EDGE('',*,*,#7539,.F.);
#10651=ORIENTED_EDGE('',*,*,#7538,.F.);
#10652=ORIENTED_EDGE('',*,*,#7540,.F.);
#10653=ORIENTED_EDGE('',*,*,#7541,.T.);
#10654=ORIENTED_EDGE('',*,*,#7542,.F.);
#10655=ORIENTED_EDGE('',*,*,#7541,.F.);
#10656=ORIENTED_EDGE('',*,*,#7543,.F.);
#10657=ORIENTED_EDGE('',*,*,#7544,.T.);
#10658=ORIENTED_EDGE('',*,*,#7545,.F.);
#10659=ORIENTED_EDGE('',*,*,#7546,.F.);
#10660=ORIENTED_EDGE('',*,*,#7544,.F.);
#10661=ORIENTED_EDGE('',*,*,#7547,.F.);
#10662=ORIENTED_EDGE('',*,*,#7548,.T.);
#10663=ORIENTED_EDGE('',*,*,#7549,.F.);
#10664=ORIENTED_EDGE('',*,*,#7548,.F.);
#10665=ORIENTED_EDGE('',*,*,#7550,.F.);
#10666=ORIENTED_EDGE('',*,*,#7551,.F.);
#10667=ORIENTED_EDGE('',*,*,#7552,.T.);
#10668=ORIENTED_EDGE('',*,*,#7553,.F.);
#10669=ORIENTED_EDGE('',*,*,#7552,.F.);
#10670=ORIENTED_EDGE('',*,*,#7554,.F.);
#10671=ORIENTED_EDGE('',*,*,#7555,.T.);
#10672=ORIENTED_EDGE('',*,*,#7556,.F.);
#10673=ORIENTED_EDGE('',*,*,#7557,.F.);
#10674=ORIENTED_EDGE('',*,*,#7555,.F.);
#10675=ORIENTED_EDGE('',*,*,#7558,.T.);
#10676=ORIENTED_EDGE('',*,*,#7559,.T.);
#10677=ORIENTED_EDGE('',*,*,#7560,.T.);
#10678=ORIENTED_EDGE('',*,*,#7559,.F.);
#10679=ORIENTED_EDGE('',*,*,#7561,.T.);
#10680=ORIENTED_EDGE('',*,*,#7562,.T.);
#10681=ORIENTED_EDGE('',*,*,#7563,.F.);
#10682=ORIENTED_EDGE('',*,*,#7562,.F.);
#10683=ORIENTED_EDGE('',*,*,#7549,.T.);
#10684=ORIENTED_EDGE('',*,*,#7564,.T.);
#10685=ORIENTED_EDGE('',*,*,#7540,.T.);
#10686=ORIENTED_EDGE('',*,*,#7564,.F.);
#10687=ORIENTED_EDGE('',*,*,#7565,.F.);
#10688=ORIENTED_EDGE('',*,*,#7566,.T.);
#10689=ORIENTED_EDGE('',*,*,#7567,.T.);
#10690=ORIENTED_EDGE('',*,*,#7566,.F.);
#10691=ORIENTED_EDGE('',*,*,#7536,.T.);
#10692=ORIENTED_EDGE('',*,*,#7537,.T.);
#10693=ORIENTED_EDGE('',*,*,#7568,.T.);
#10694=ORIENTED_EDGE('',*,*,#7556,.T.);
#10695=ORIENTED_EDGE('',*,*,#7557,.T.);
#10696=ORIENTED_EDGE('',*,*,#7568,.F.);
#10697=ORIENTED_EDGE('',*,*,#7550,.T.);
#10698=ORIENTED_EDGE('',*,*,#7551,.T.);
#10699=ORIENTED_EDGE('',*,*,#7569,.T.);
#10700=ORIENTED_EDGE('',*,*,#7545,.T.);
#10701=ORIENTED_EDGE('',*,*,#7546,.T.);
#10702=ORIENTED_EDGE('',*,*,#7569,.F.);
#10703=ORIENTED_EDGE('',*,*,#7543,.T.);
#10704=ORIENTED_EDGE('',*,*,#7542,.T.);
#10705=ORIENTED_EDGE('',*,*,#7553,.T.);
#10706=ORIENTED_EDGE('',*,*,#7539,.T.);
#10707=ORIENTED_EDGE('',*,*,#7554,.T.);
#10708=ORIENTED_EDGE('',*,*,#7565,.T.);
#10709=ORIENTED_EDGE('',*,*,#7547,.T.);
#10710=ORIENTED_EDGE('',*,*,#7561,.F.);
#10711=ORIENTED_EDGE('',*,*,#7567,.F.);
#10712=ORIENTED_EDGE('',*,*,#7558,.F.);
#10713=ORIENTED_EDGE('',*,*,#7563,.T.);
#10714=ORIENTED_EDGE('',*,*,#7560,.F.);
#10715=ORIENTED_EDGE('',*,*,#7570,.F.);
#10716=ORIENTED_EDGE('',*,*,#7571,.T.);
#10717=ORIENTED_EDGE('',*,*,#7572,.F.);
#10718=ORIENTED_EDGE('',*,*,#7571,.F.);
#10719=ORIENTED_EDGE('',*,*,#7573,.F.);
#10720=ORIENTED_EDGE('',*,*,#7574,.F.);
#10721=ORIENTED_EDGE('',*,*,#7575,.T.);
#10722=ORIENTED_EDGE('',*,*,#7576,.F.);
#10723=ORIENTED_EDGE('',*,*,#7575,.F.);
#10724=ORIENTED_EDGE('',*,*,#7573,.T.);
#10725=ORIENTED_EDGE('',*,*,#7574,.T.);
#10726=ORIENTED_EDGE('',*,*,#7577,.T.);
#10727=ORIENTED_EDGE('',*,*,#7570,.T.);
#10728=ORIENTED_EDGE('',*,*,#7577,.F.);
#10729=ORIENTED_EDGE('',*,*,#7572,.T.);
#10730=ORIENTED_EDGE('',*,*,#7576,.T.);
#10731=ORIENTED_EDGE('',*,*,#7578,.F.);
#10732=ORIENTED_EDGE('',*,*,#7579,.T.);
#10733=ORIENTED_EDGE('',*,*,#7580,.T.);
#10734=ORIENTED_EDGE('',*,*,#7581,.F.);
#10735=ORIENTED_EDGE('',*,*,#7582,.F.);
#10736=ORIENTED_EDGE('',*,*,#7583,.T.);
#10737=ORIENTED_EDGE('',*,*,#7578,.T.);
#10738=ORIENTED_EDGE('',*,*,#7584,.F.);
#10739=ORIENTED_EDGE('',*,*,#7585,.F.);
#10740=ORIENTED_EDGE('',*,*,#7586,.T.);
#10741=ORIENTED_EDGE('',*,*,#7582,.T.);
#10742=ORIENTED_EDGE('',*,*,#7587,.F.);
#10743=ORIENTED_EDGE('',*,*,#7588,.F.);
#10744=ORIENTED_EDGE('',*,*,#7589,.T.);
#10745=ORIENTED_EDGE('',*,*,#7585,.T.);
#10746=ORIENTED_EDGE('',*,*,#7590,.F.);
#10747=ORIENTED_EDGE('',*,*,#7591,.F.);
#10748=ORIENTED_EDGE('',*,*,#7592,.T.);
#10749=ORIENTED_EDGE('',*,*,#7588,.T.);
#10750=ORIENTED_EDGE('',*,*,#7593,.F.);
#10751=ORIENTED_EDGE('',*,*,#7594,.F.);
#10752=ORIENTED_EDGE('',*,*,#7595,.T.);
#10753=ORIENTED_EDGE('',*,*,#7591,.T.);
#10754=ORIENTED_EDGE('',*,*,#7596,.F.);
#10755=ORIENTED_EDGE('',*,*,#7597,.F.);
#10756=ORIENTED_EDGE('',*,*,#7598,.T.);
#10757=ORIENTED_EDGE('',*,*,#7594,.T.);
#10758=ORIENTED_EDGE('',*,*,#7599,.F.);
#10759=ORIENTED_EDGE('',*,*,#7600,.F.);
#10760=ORIENTED_EDGE('',*,*,#7601,.T.);
#10761=ORIENTED_EDGE('',*,*,#7597,.T.);
#10762=ORIENTED_EDGE('',*,*,#7602,.F.);
#10763=ORIENTED_EDGE('',*,*,#7603,.F.);
#10764=ORIENTED_EDGE('',*,*,#7604,.T.);
#10765=ORIENTED_EDGE('',*,*,#7600,.T.);
#10766=ORIENTED_EDGE('',*,*,#7605,.F.);
#10767=ORIENTED_EDGE('',*,*,#7606,.F.);
#10768=ORIENTED_EDGE('',*,*,#7607,.T.);
#10769=ORIENTED_EDGE('',*,*,#7603,.T.);
#10770=ORIENTED_EDGE('',*,*,#7608,.F.);
#10771=ORIENTED_EDGE('',*,*,#7609,.F.);
#10772=ORIENTED_EDGE('',*,*,#7610,.T.);
#10773=ORIENTED_EDGE('',*,*,#7606,.T.);
#10774=ORIENTED_EDGE('',*,*,#7611,.F.);
#10775=ORIENTED_EDGE('',*,*,#7612,.F.);
#10776=ORIENTED_EDGE('',*,*,#7613,.T.);
#10777=ORIENTED_EDGE('',*,*,#7609,.T.);
#10778=ORIENTED_EDGE('',*,*,#7614,.F.);
#10779=ORIENTED_EDGE('',*,*,#7615,.F.);
#10780=ORIENTED_EDGE('',*,*,#7616,.T.);
#10781=ORIENTED_EDGE('',*,*,#7612,.T.);
#10782=ORIENTED_EDGE('',*,*,#7617,.F.);
#10783=ORIENTED_EDGE('',*,*,#7618,.F.);
#10784=ORIENTED_EDGE('',*,*,#7619,.T.);
#10785=ORIENTED_EDGE('',*,*,#7620,.T.);
#10786=ORIENTED_EDGE('',*,*,#7621,.T.);
#10787=ORIENTED_EDGE('',*,*,#7620,.F.);
#10788=ORIENTED_EDGE('',*,*,#7622,.T.);
#10789=ORIENTED_EDGE('',*,*,#7623,.T.);
#10790=ORIENTED_EDGE('',*,*,#7624,.F.);
#10791=ORIENTED_EDGE('',*,*,#7625,.F.);
#10792=ORIENTED_EDGE('',*,*,#7626,.T.);
#10793=ORIENTED_EDGE('',*,*,#7618,.T.);
#10794=ORIENTED_EDGE('',*,*,#7627,.F.);
#10795=ORIENTED_EDGE('',*,*,#7628,.F.);
#10796=ORIENTED_EDGE('',*,*,#7629,.T.);
#10797=ORIENTED_EDGE('',*,*,#7625,.T.);
#10798=ORIENTED_EDGE('',*,*,#7630,.F.);
#10799=ORIENTED_EDGE('',*,*,#7631,.F.);
#10800=ORIENTED_EDGE('',*,*,#7632,.T.);
#10801=ORIENTED_EDGE('',*,*,#7628,.T.);
#10802=ORIENTED_EDGE('',*,*,#7633,.F.);
#10803=ORIENTED_EDGE('',*,*,#7634,.F.);
#10804=ORIENTED_EDGE('',*,*,#7635,.T.);
#10805=ORIENTED_EDGE('',*,*,#7631,.T.);
#10806=ORIENTED_EDGE('',*,*,#7636,.F.);
#10807=ORIENTED_EDGE('',*,*,#7637,.F.);
#10808=ORIENTED_EDGE('',*,*,#7638,.T.);
#10809=ORIENTED_EDGE('',*,*,#7634,.T.);
#10810=ORIENTED_EDGE('',*,*,#7639,.F.);
#10811=ORIENTED_EDGE('',*,*,#7640,.F.);
#10812=ORIENTED_EDGE('',*,*,#7641,.T.);
#10813=ORIENTED_EDGE('',*,*,#7637,.T.);
#10814=ORIENTED_EDGE('',*,*,#7642,.F.);
#10815=ORIENTED_EDGE('',*,*,#7643,.F.);
#10816=ORIENTED_EDGE('',*,*,#7644,.T.);
#10817=ORIENTED_EDGE('',*,*,#7640,.T.);
#10818=ORIENTED_EDGE('',*,*,#7645,.F.);
#10819=ORIENTED_EDGE('',*,*,#7646,.F.);
#10820=ORIENTED_EDGE('',*,*,#7647,.T.);
#10821=ORIENTED_EDGE('',*,*,#7643,.T.);
#10822=ORIENTED_EDGE('',*,*,#7648,.F.);
#10823=ORIENTED_EDGE('',*,*,#7649,.F.);
#10824=ORIENTED_EDGE('',*,*,#7650,.T.);
#10825=ORIENTED_EDGE('',*,*,#7646,.T.);
#10826=ORIENTED_EDGE('',*,*,#7651,.F.);
#10827=ORIENTED_EDGE('',*,*,#7652,.F.);
#10828=ORIENTED_EDGE('',*,*,#7653,.T.);
#10829=ORIENTED_EDGE('',*,*,#7649,.T.);
#10830=ORIENTED_EDGE('',*,*,#7654,.F.);
#10831=ORIENTED_EDGE('',*,*,#7655,.F.);
#10832=ORIENTED_EDGE('',*,*,#7656,.T.);
#10833=ORIENTED_EDGE('',*,*,#7652,.T.);
#10834=ORIENTED_EDGE('',*,*,#7657,.F.);
#10835=ORIENTED_EDGE('',*,*,#7655,.T.);
#10836=ORIENTED_EDGE('',*,*,#7658,.F.);
#10837=ORIENTED_EDGE('',*,*,#7659,.T.);
#10838=ORIENTED_EDGE('',*,*,#7660,.T.);
#10839=ORIENTED_EDGE('',*,*,#7661,.F.);
#10840=ORIENTED_EDGE('',*,*,#7662,.T.);
#10841=ORIENTED_EDGE('',*,*,#7663,.T.);
#10842=ORIENTED_EDGE('',*,*,#7664,.T.);
#10843=ORIENTED_EDGE('',*,*,#7665,.T.);
#10844=ORIENTED_EDGE('',*,*,#7666,.T.);
#10845=ORIENTED_EDGE('',*,*,#7662,.F.);
#10846=ORIENTED_EDGE('',*,*,#7667,.T.);
#10847=ORIENTED_EDGE('',*,*,#7668,.T.);
#10848=ORIENTED_EDGE('',*,*,#7669,.T.);
#10849=ORIENTED_EDGE('',*,*,#7668,.F.);
#10850=ORIENTED_EDGE('',*,*,#7670,.F.);
#10851=ORIENTED_EDGE('',*,*,#7671,.T.);
#10852=ORIENTED_EDGE('',*,*,#7672,.T.);
#10853=ORIENTED_EDGE('',*,*,#7671,.F.);
#10854=ORIENTED_EDGE('',*,*,#7673,.T.);
#10855=ORIENTED_EDGE('',*,*,#7674,.T.);
#10856=ORIENTED_EDGE('',*,*,#7675,.F.);
#10857=ORIENTED_EDGE('',*,*,#7674,.F.);
#10858=ORIENTED_EDGE('',*,*,#7676,.T.);
#10859=ORIENTED_EDGE('',*,*,#7677,.T.);
#10860=ORIENTED_EDGE('',*,*,#7678,.T.);
#10861=ORIENTED_EDGE('',*,*,#7659,.F.);
#10862=ORIENTED_EDGE('',*,*,#7679,.T.);
#10863=ORIENTED_EDGE('',*,*,#7680,.T.);
#10864=ORIENTED_EDGE('',*,*,#7663,.F.);
#10865=ORIENTED_EDGE('',*,*,#7666,.F.);
#10866=ORIENTED_EDGE('',*,*,#7681,.T.);
#10867=ORIENTED_EDGE('',*,*,#7682,.F.);
#10868=ORIENTED_EDGE('',*,*,#7683,.T.);
#10869=ORIENTED_EDGE('',*,*,#7665,.F.);
#10870=ORIENTED_EDGE('',*,*,#7684,.F.);
#10871=ORIENTED_EDGE('',*,*,#7685,.T.);
#10872=ORIENTED_EDGE('',*,*,#7686,.F.);
#10873=ORIENTED_EDGE('',*,*,#7687,.F.);
#10874=ORIENTED_EDGE('',*,*,#7672,.F.);
#10875=ORIENTED_EDGE('',*,*,#7688,.T.);
#10876=ORIENTED_EDGE('',*,*,#7689,.T.);
#10877=ORIENTED_EDGE('',*,*,#7690,.T.);
#10878=ORIENTED_EDGE('',*,*,#7691,.T.);
#10879=ORIENTED_EDGE('',*,*,#7670,.T.);
#10880=ORIENTED_EDGE('',*,*,#7664,.F.);
#10881=ORIENTED_EDGE('',*,*,#7692,.T.);
#10882=ORIENTED_EDGE('',*,*,#7693,.F.);
#10883=ORIENTED_EDGE('',*,*,#7694,.F.);
#10884=ORIENTED_EDGE('',*,*,#7695,.T.);
#10885=ORIENTED_EDGE('',*,*,#7696,.F.);
#10886=ORIENTED_EDGE('',*,*,#7697,.F.);
#10887=ORIENTED_EDGE('',*,*,#7669,.F.);
#10888=ORIENTED_EDGE('',*,*,#7698,.F.);
#10889=ORIENTED_EDGE('',*,*,#7699,.T.);
#10890=ORIENTED_EDGE('',*,*,#7700,.F.);
#10891=ORIENTED_EDGE('',*,*,#7701,.F.);
#10892=ORIENTED_EDGE('',*,*,#7667,.F.);
#10893=ORIENTED_EDGE('',*,*,#7702,.T.);
#10894=ORIENTED_EDGE('',*,*,#7703,.T.);
#10895=ORIENTED_EDGE('',*,*,#7704,.F.);
#10896=ORIENTED_EDGE('',*,*,#7705,.T.);
#10897=ORIENTED_EDGE('',*,*,#7706,.F.);
#10898=ORIENTED_EDGE('',*,*,#7707,.T.);
#10899=ORIENTED_EDGE('',*,*,#7679,.F.);
#10900=ORIENTED_EDGE('',*,*,#7708,.T.);
#10901=ORIENTED_EDGE('',*,*,#7709,.F.);
#10902=ORIENTED_EDGE('',*,*,#7702,.F.);
#10903=ORIENTED_EDGE('',*,*,#7693,.T.);
#10904=ORIENTED_EDGE('',*,*,#7710,.T.);
#10905=ORIENTED_EDGE('',*,*,#7711,.T.);
#10906=ORIENTED_EDGE('',*,*,#7704,.T.);
#10907=ORIENTED_EDGE('',*,*,#7712,.T.);
#10908=ORIENTED_EDGE('',*,*,#7713,.T.);
#10909=ORIENTED_EDGE('',*,*,#7682,.T.);
#10910=ORIENTED_EDGE('',*,*,#7696,.T.);
#10911=ORIENTED_EDGE('',*,*,#7714,.T.);
#10912=ORIENTED_EDGE('',*,*,#7712,.F.);
#10913=ORIENTED_EDGE('',*,*,#7715,.T.);
#10914=ORIENTED_EDGE('',*,*,#7698,.T.);
#10915=ORIENTED_EDGE('',*,*,#7716,.T.);
#10916=ORIENTED_EDGE('',*,*,#7709,.T.);
#10917=ORIENTED_EDGE('',*,*,#7717,.T.);
#10918=ORIENTED_EDGE('',*,*,#7694,.T.);
#10919=ORIENTED_EDGE('',*,*,#7718,.F.);
#10920=ORIENTED_EDGE('',*,*,#7700,.T.);
#10921=ORIENTED_EDGE('',*,*,#7719,.T.);
#10922=ORIENTED_EDGE('',*,*,#7697,.T.);
#10923=ORIENTED_EDGE('',*,*,#7716,.F.);
#10924=ORIENTED_EDGE('',*,*,#7701,.T.);
#10925=ORIENTED_EDGE('',*,*,#7718,.T.);
#10926=ORIENTED_EDGE('',*,*,#7687,.T.);
#10927=ORIENTED_EDGE('',*,*,#7720,.F.);
#10928=ORIENTED_EDGE('',*,*,#7691,.F.);
#10929=ORIENTED_EDGE('',*,*,#7721,.T.);
#10930=ORIENTED_EDGE('',*,*,#7690,.F.);
#10931=ORIENTED_EDGE('',*,*,#7722,.T.);
#10932=ORIENTED_EDGE('',*,*,#7706,.T.);
#10933=ORIENTED_EDGE('',*,*,#7723,.T.);
#10934=ORIENTED_EDGE('',*,*,#7684,.T.);
#10935=ORIENTED_EDGE('',*,*,#7721,.F.);
#10936=ORIENTED_EDGE('',*,*,#7711,.F.);
#10937=ORIENTED_EDGE('',*,*,#7724,.T.);
#10938=ORIENTED_EDGE('',*,*,#7688,.F.);
#10939=ORIENTED_EDGE('',*,*,#7720,.T.);
#10940=ORIENTED_EDGE('',*,*,#7686,.T.);
#10941=ORIENTED_EDGE('',*,*,#7725,.T.);
#10942=ORIENTED_EDGE('',*,*,#7661,.T.);
#10943=ORIENTED_EDGE('',*,*,#7621,.F.);
#10944=ORIENTED_EDGE('',*,*,#7675,.T.);
#10945=ORIENTED_EDGE('',*,*,#7726,.F.);
#10946=ORIENTED_EDGE('',*,*,#7623,.F.);
#10947=ORIENTED_EDGE('',*,*,#7727,.F.);
#10948=ORIENTED_EDGE('',*,*,#7580,.F.);
#10949=ORIENTED_EDGE('',*,*,#7658,.T.);
#10950=ORIENTED_EDGE('',*,*,#7657,.T.);
#10951=ORIENTED_EDGE('',*,*,#7654,.T.);
#10952=ORIENTED_EDGE('',*,*,#7651,.T.);
#10953=ORIENTED_EDGE('',*,*,#7648,.T.);
#10954=ORIENTED_EDGE('',*,*,#7645,.T.);
#10955=ORIENTED_EDGE('',*,*,#7642,.T.);
#10956=ORIENTED_EDGE('',*,*,#7639,.T.);
#10957=ORIENTED_EDGE('',*,*,#7636,.T.);
#10958=ORIENTED_EDGE('',*,*,#7633,.T.);
#10959=ORIENTED_EDGE('',*,*,#7630,.T.);
#10960=ORIENTED_EDGE('',*,*,#7627,.T.);
#10961=ORIENTED_EDGE('',*,*,#7624,.T.);
#10962=ORIENTED_EDGE('',*,*,#7726,.T.);
#10963=ORIENTED_EDGE('',*,*,#7579,.F.);
#10964=ORIENTED_EDGE('',*,*,#7583,.F.);
#10965=ORIENTED_EDGE('',*,*,#7586,.F.);
#10966=ORIENTED_EDGE('',*,*,#7589,.F.);
#10967=ORIENTED_EDGE('',*,*,#7592,.F.);
#10968=ORIENTED_EDGE('',*,*,#7595,.F.);
#10969=ORIENTED_EDGE('',*,*,#7598,.F.);
#10970=ORIENTED_EDGE('',*,*,#7601,.F.);
#10971=ORIENTED_EDGE('',*,*,#7604,.F.);
#10972=ORIENTED_EDGE('',*,*,#7607,.F.);
#10973=ORIENTED_EDGE('',*,*,#7610,.F.);
#10974=ORIENTED_EDGE('',*,*,#7613,.F.);
#10975=ORIENTED_EDGE('',*,*,#7616,.F.);
#10976=ORIENTED_EDGE('',*,*,#7728,.F.);
#10977=ORIENTED_EDGE('',*,*,#7676,.F.);
#10978=ORIENTED_EDGE('',*,*,#7673,.F.);
#10979=ORIENTED_EDGE('',*,*,#7615,.T.);
#10980=ORIENTED_EDGE('',*,*,#7729,.F.);
#10981=ORIENTED_EDGE('',*,*,#7677,.F.);
#10982=ORIENTED_EDGE('',*,*,#7728,.T.);
#10983=ORIENTED_EDGE('',*,*,#7729,.T.);
#10984=ORIENTED_EDGE('',*,*,#7617,.T.);
#10985=ORIENTED_EDGE('',*,*,#7614,.T.);
#10986=ORIENTED_EDGE('',*,*,#7611,.T.);
#10987=ORIENTED_EDGE('',*,*,#7608,.T.);
#10988=ORIENTED_EDGE('',*,*,#7605,.T.);
#10989=ORIENTED_EDGE('',*,*,#7602,.T.);
#10990=ORIENTED_EDGE('',*,*,#7599,.T.);
#10991=ORIENTED_EDGE('',*,*,#7596,.T.);
#10992=ORIENTED_EDGE('',*,*,#7593,.T.);
#10993=ORIENTED_EDGE('',*,*,#7590,.T.);
#10994=ORIENTED_EDGE('',*,*,#7587,.T.);
#10995=ORIENTED_EDGE('',*,*,#7584,.T.);
#10996=ORIENTED_EDGE('',*,*,#7581,.T.);
#10997=ORIENTED_EDGE('',*,*,#7727,.T.);
#10998=ORIENTED_EDGE('',*,*,#7622,.F.);
#10999=ORIENTED_EDGE('',*,*,#7619,.F.);
#11000=ORIENTED_EDGE('',*,*,#7626,.F.);
#11001=ORIENTED_EDGE('',*,*,#7629,.F.);
#11002=ORIENTED_EDGE('',*,*,#7632,.F.);
#11003=ORIENTED_EDGE('',*,*,#7635,.F.);
#11004=ORIENTED_EDGE('',*,*,#7638,.F.);
#11005=ORIENTED_EDGE('',*,*,#7641,.F.);
#11006=ORIENTED_EDGE('',*,*,#7644,.F.);
#11007=ORIENTED_EDGE('',*,*,#7647,.F.);
#11008=ORIENTED_EDGE('',*,*,#7650,.F.);
#11009=ORIENTED_EDGE('',*,*,#7653,.F.);
#11010=ORIENTED_EDGE('',*,*,#7656,.F.);
#11011=ORIENTED_EDGE('',*,*,#7660,.F.);
#11012=ORIENTED_EDGE('',*,*,#7678,.F.);
#11013=ORIENTED_EDGE('',*,*,#7722,.F.);
#11014=ORIENTED_EDGE('',*,*,#7689,.F.);
#11015=ORIENTED_EDGE('',*,*,#7724,.F.);
#11016=ORIENTED_EDGE('',*,*,#7710,.F.);
#11017=ORIENTED_EDGE('',*,*,#7692,.F.);
#11018=ORIENTED_EDGE('',*,*,#7680,.F.);
#11019=ORIENTED_EDGE('',*,*,#7707,.F.);
#11020=ORIENTED_EDGE('',*,*,#7681,.F.);
#11021=ORIENTED_EDGE('',*,*,#7683,.F.);
#11022=ORIENTED_EDGE('',*,*,#7713,.F.);
#11023=ORIENTED_EDGE('',*,*,#7714,.F.);
#11024=ORIENTED_EDGE('',*,*,#7695,.F.);
#11025=ORIENTED_EDGE('',*,*,#7717,.F.);
#11026=ORIENTED_EDGE('',*,*,#7708,.F.);
#11027=ORIENTED_EDGE('',*,*,#7719,.F.);
#11028=ORIENTED_EDGE('',*,*,#7699,.F.);
#11029=ORIENTED_EDGE('',*,*,#7715,.F.);
#11030=ORIENTED_EDGE('',*,*,#7703,.F.);
#11031=ORIENTED_EDGE('',*,*,#7723,.F.);
#11032=ORIENTED_EDGE('',*,*,#7705,.F.);
#11033=ORIENTED_EDGE('',*,*,#7725,.F.);
#11034=ORIENTED_EDGE('',*,*,#7685,.F.);
#11035=ORIENTED_EDGE('',*,*,#7730,.T.);
#11036=ORIENTED_EDGE('',*,*,#7731,.F.);
#11037=ORIENTED_EDGE('',*,*,#7732,.F.);
#11038=ORIENTED_EDGE('',*,*,#7733,.T.);
#11039=ORIENTED_EDGE('',*,*,#7734,.T.);
#11040=ORIENTED_EDGE('',*,*,#7735,.F.);
#11041=ORIENTED_EDGE('',*,*,#7730,.F.);
#11042=ORIENTED_EDGE('',*,*,#7736,.T.);
#11043=ORIENTED_EDGE('',*,*,#7737,.T.);
#11044=ORIENTED_EDGE('',*,*,#7738,.F.);
#11045=ORIENTED_EDGE('',*,*,#7734,.F.);
#11046=ORIENTED_EDGE('',*,*,#7739,.T.);
#11047=ORIENTED_EDGE('',*,*,#7740,.T.);
#11048=ORIENTED_EDGE('',*,*,#7741,.F.);
#11049=ORIENTED_EDGE('',*,*,#7737,.F.);
#11050=ORIENTED_EDGE('',*,*,#7742,.T.);
#11051=ORIENTED_EDGE('',*,*,#7743,.T.);
#11052=ORIENTED_EDGE('',*,*,#7744,.F.);
#11053=ORIENTED_EDGE('',*,*,#7740,.F.);
#11054=ORIENTED_EDGE('',*,*,#7745,.T.);
#11055=ORIENTED_EDGE('',*,*,#7746,.T.);
#11056=ORIENTED_EDGE('',*,*,#7747,.F.);
#11057=ORIENTED_EDGE('',*,*,#7743,.F.);
#11058=ORIENTED_EDGE('',*,*,#7748,.T.);
#11059=ORIENTED_EDGE('',*,*,#7749,.T.);
#11060=ORIENTED_EDGE('',*,*,#7750,.F.);
#11061=ORIENTED_EDGE('',*,*,#7746,.F.);
#11062=ORIENTED_EDGE('',*,*,#7751,.T.);
#11063=ORIENTED_EDGE('',*,*,#7752,.F.);
#11064=ORIENTED_EDGE('',*,*,#7753,.T.);
#11065=ORIENTED_EDGE('',*,*,#7754,.T.);
#11066=ORIENTED_EDGE('',*,*,#7755,.F.);
#11067=ORIENTED_EDGE('',*,*,#7756,.T.);
#11068=ORIENTED_EDGE('',*,*,#7757,.T.);
#11069=ORIENTED_EDGE('',*,*,#7758,.T.);
#11070=ORIENTED_EDGE('',*,*,#7759,.F.);
#11071=ORIENTED_EDGE('',*,*,#7760,.T.);
#11072=ORIENTED_EDGE('',*,*,#7761,.F.);
#11073=ORIENTED_EDGE('',*,*,#7760,.F.);
#11074=ORIENTED_EDGE('',*,*,#7762,.F.);
#11075=ORIENTED_EDGE('',*,*,#7763,.T.);
#11076=ORIENTED_EDGE('',*,*,#7764,.T.);
#11077=ORIENTED_EDGE('',*,*,#7756,.F.);
#11078=ORIENTED_EDGE('',*,*,#7765,.F.);
#11079=ORIENTED_EDGE('',*,*,#7766,.T.);
#11080=ORIENTED_EDGE('',*,*,#7767,.T.);
#11081=ORIENTED_EDGE('',*,*,#7763,.F.);
#11082=ORIENTED_EDGE('',*,*,#7768,.F.);
#11083=ORIENTED_EDGE('',*,*,#7769,.T.);
#11084=ORIENTED_EDGE('',*,*,#7770,.T.);
#11085=ORIENTED_EDGE('',*,*,#7766,.F.);
#11086=ORIENTED_EDGE('',*,*,#7771,.F.);
#11087=ORIENTED_EDGE('',*,*,#7772,.T.);
#11088=ORIENTED_EDGE('',*,*,#7773,.T.);
#11089=ORIENTED_EDGE('',*,*,#7769,.F.);
#11090=ORIENTED_EDGE('',*,*,#7774,.F.);
#11091=ORIENTED_EDGE('',*,*,#7775,.T.);
#11092=ORIENTED_EDGE('',*,*,#7776,.T.);
#11093=ORIENTED_EDGE('',*,*,#7772,.F.);
#11094=ORIENTED_EDGE('',*,*,#7777,.F.);
#11095=ORIENTED_EDGE('',*,*,#7778,.T.);
#11096=ORIENTED_EDGE('',*,*,#7779,.T.);
#11097=ORIENTED_EDGE('',*,*,#7775,.F.);
#11098=ORIENTED_EDGE('',*,*,#7780,.F.);
#11099=ORIENTED_EDGE('',*,*,#7781,.F.);
#11100=ORIENTED_EDGE('',*,*,#7782,.F.);
#11101=ORIENTED_EDGE('',*,*,#7783,.T.);
#11102=ORIENTED_EDGE('',*,*,#7784,.T.);
#11103=ORIENTED_EDGE('',*,*,#7781,.T.);
#11104=ORIENTED_EDGE('',*,*,#7785,.T.);
#11105=ORIENTED_EDGE('',*,*,#7778,.F.);
#11106=ORIENTED_EDGE('',*,*,#7786,.F.);
#11107=ORIENTED_EDGE('',*,*,#7787,.T.);
#11108=ORIENTED_EDGE('',*,*,#7788,.T.);
#11109=ORIENTED_EDGE('',*,*,#7789,.F.);
#11110=ORIENTED_EDGE('',*,*,#7788,.F.);
#11111=ORIENTED_EDGE('',*,*,#7790,.T.);
#11112=ORIENTED_EDGE('',*,*,#7791,.T.);
#11113=ORIENTED_EDGE('',*,*,#7792,.T.);
#11114=ORIENTED_EDGE('',*,*,#7793,.T.);
#11115=ORIENTED_EDGE('',*,*,#7794,.T.);
#11116=ORIENTED_EDGE('',*,*,#7795,.T.);
#11117=ORIENTED_EDGE('',*,*,#7796,.T.);
#11118=ORIENTED_EDGE('',*,*,#7797,.T.);
#11119=ORIENTED_EDGE('',*,*,#7798,.T.);
#11120=ORIENTED_EDGE('',*,*,#7799,.T.);
#11121=ORIENTED_EDGE('',*,*,#7800,.T.);
#11122=ORIENTED_EDGE('',*,*,#7801,.T.);
#11123=ORIENTED_EDGE('',*,*,#7732,.T.);
#11124=ORIENTED_EDGE('',*,*,#7802,.T.);
#11125=ORIENTED_EDGE('',*,*,#7783,.F.);
#11126=ORIENTED_EDGE('',*,*,#7803,.T.);
#11127=ORIENTED_EDGE('',*,*,#7789,.T.);
#11128=ORIENTED_EDGE('',*,*,#7804,.F.);
#11129=ORIENTED_EDGE('',*,*,#7805,.F.);
#11130=ORIENTED_EDGE('',*,*,#7806,.F.);
#11131=ORIENTED_EDGE('',*,*,#7807,.F.);
#11132=ORIENTED_EDGE('',*,*,#7808,.F.);
#11133=ORIENTED_EDGE('',*,*,#7809,.F.);
#11134=ORIENTED_EDGE('',*,*,#7787,.F.);
#11135=ORIENTED_EDGE('',*,*,#7761,.T.);
#11136=ORIENTED_EDGE('',*,*,#7810,.F.);
#11137=ORIENTED_EDGE('',*,*,#7790,.F.);
#11138=ORIENTED_EDGE('',*,*,#7811,.F.);
#11139=ORIENTED_EDGE('',*,*,#7812,.T.);
#11140=ORIENTED_EDGE('',*,*,#7804,.T.);
#11141=ORIENTED_EDGE('',*,*,#7813,.F.);
#11142=ORIENTED_EDGE('',*,*,#7814,.F.);
#11143=ORIENTED_EDGE('',*,*,#7813,.T.);
#11144=ORIENTED_EDGE('',*,*,#7809,.T.);
#11145=ORIENTED_EDGE('',*,*,#7815,.F.);
#11146=ORIENTED_EDGE('',*,*,#7816,.F.);
#11147=ORIENTED_EDGE('',*,*,#7792,.F.);
#11148=ORIENTED_EDGE('',*,*,#7817,.F.);
#11149=ORIENTED_EDGE('',*,*,#7794,.F.);
#11150=ORIENTED_EDGE('',*,*,#7818,.F.);
#11151=ORIENTED_EDGE('',*,*,#7815,.T.);
#11152=ORIENTED_EDGE('',*,*,#7808,.T.);
#11153=ORIENTED_EDGE('',*,*,#7819,.F.);
#11154=ORIENTED_EDGE('',*,*,#7820,.F.);
#11155=ORIENTED_EDGE('',*,*,#7819,.T.);
#11156=ORIENTED_EDGE('',*,*,#7807,.T.);
#11157=ORIENTED_EDGE('',*,*,#7821,.F.);
#11158=ORIENTED_EDGE('',*,*,#7822,.F.);
#11159=ORIENTED_EDGE('',*,*,#7796,.F.);
#11160=ORIENTED_EDGE('',*,*,#7823,.F.);
#11161=ORIENTED_EDGE('',*,*,#7798,.F.);
#11162=ORIENTED_EDGE('',*,*,#7824,.F.);
#11163=ORIENTED_EDGE('',*,*,#7821,.T.);
#11164=ORIENTED_EDGE('',*,*,#7806,.T.);
#11165=ORIENTED_EDGE('',*,*,#7825,.F.);
#11166=ORIENTED_EDGE('',*,*,#7826,.F.);
#11167=ORIENTED_EDGE('',*,*,#7800,.F.);
#11168=ORIENTED_EDGE('',*,*,#7827,.F.);
#11169=ORIENTED_EDGE('',*,*,#7825,.T.);
#11170=ORIENTED_EDGE('',*,*,#7805,.T.);
#11171=ORIENTED_EDGE('',*,*,#7812,.F.);
#11172=ORIENTED_EDGE('',*,*,#7754,.F.);
#11173=ORIENTED_EDGE('',*,*,#7828,.F.);
#11174=ORIENTED_EDGE('',*,*,#7758,.F.);
#11175=ORIENTED_EDGE('',*,*,#7829,.F.);
#11176=ORIENTED_EDGE('',*,*,#7752,.T.);
#11177=ORIENTED_EDGE('',*,*,#7830,.F.);
#11178=ORIENTED_EDGE('',*,*,#7749,.F.);
#11179=ORIENTED_EDGE('',*,*,#7831,.T.);
#11180=ORIENTED_EDGE('',*,*,#7731,.T.);
#11181=ORIENTED_EDGE('',*,*,#7735,.T.);
#11182=ORIENTED_EDGE('',*,*,#7738,.T.);
#11183=ORIENTED_EDGE('',*,*,#7741,.T.);
#11184=ORIENTED_EDGE('',*,*,#7744,.T.);
#11185=ORIENTED_EDGE('',*,*,#7747,.T.);
#11186=ORIENTED_EDGE('',*,*,#7750,.T.);
#11187=ORIENTED_EDGE('',*,*,#7830,.T.);
#11188=ORIENTED_EDGE('',*,*,#7755,.T.);
#11189=ORIENTED_EDGE('',*,*,#7829,.T.);
#11190=ORIENTED_EDGE('',*,*,#7757,.F.);
#11191=ORIENTED_EDGE('',*,*,#7764,.F.);
#11192=ORIENTED_EDGE('',*,*,#7767,.F.);
#11193=ORIENTED_EDGE('',*,*,#7770,.F.);
#11194=ORIENTED_EDGE('',*,*,#7773,.F.);
#11195=ORIENTED_EDGE('',*,*,#7776,.F.);
#11196=ORIENTED_EDGE('',*,*,#7779,.F.);
#11197=ORIENTED_EDGE('',*,*,#7785,.F.);
#11198=ORIENTED_EDGE('',*,*,#7784,.F.);
#11199=ORIENTED_EDGE('',*,*,#7802,.F.);
#11200=ORIENTED_EDGE('',*,*,#7782,.T.);
#11201=ORIENTED_EDGE('',*,*,#7786,.T.);
#11202=ORIENTED_EDGE('',*,*,#7780,.T.);
#11203=ORIENTED_EDGE('',*,*,#7777,.T.);
#11204=ORIENTED_EDGE('',*,*,#7774,.T.);
#11205=ORIENTED_EDGE('',*,*,#7771,.T.);
#11206=ORIENTED_EDGE('',*,*,#7768,.T.);
#11207=ORIENTED_EDGE('',*,*,#7765,.T.);
#11208=ORIENTED_EDGE('',*,*,#7762,.T.);
#11209=ORIENTED_EDGE('',*,*,#7759,.T.);
#11210=ORIENTED_EDGE('',*,*,#7828,.T.);
#11211=ORIENTED_EDGE('',*,*,#7753,.F.);
#11212=ORIENTED_EDGE('',*,*,#7831,.F.);
#11213=ORIENTED_EDGE('',*,*,#7751,.F.);
#11214=ORIENTED_EDGE('',*,*,#7748,.F.);
#11215=ORIENTED_EDGE('',*,*,#7745,.F.);
#11216=ORIENTED_EDGE('',*,*,#7742,.F.);
#11217=ORIENTED_EDGE('',*,*,#7739,.F.);
#11218=ORIENTED_EDGE('',*,*,#7736,.F.);
#11219=ORIENTED_EDGE('',*,*,#7733,.F.);
#11220=ORIENTED_EDGE('',*,*,#7803,.F.);
#11221=ORIENTED_EDGE('',*,*,#7797,.F.);
#11222=ORIENTED_EDGE('',*,*,#7822,.T.);
#11223=ORIENTED_EDGE('',*,*,#7824,.T.);
#11224=ORIENTED_EDGE('',*,*,#7793,.F.);
#11225=ORIENTED_EDGE('',*,*,#7816,.T.);
#11226=ORIENTED_EDGE('',*,*,#7818,.T.);
#11227=ORIENTED_EDGE('',*,*,#7795,.F.);
#11228=ORIENTED_EDGE('',*,*,#7817,.T.);
#11229=ORIENTED_EDGE('',*,*,#7820,.T.);
#11230=ORIENTED_EDGE('',*,*,#7799,.F.);
#11231=ORIENTED_EDGE('',*,*,#7823,.T.);
#11232=ORIENTED_EDGE('',*,*,#7827,.T.);
#11233=ORIENTED_EDGE('',*,*,#7801,.F.);
#11234=ORIENTED_EDGE('',*,*,#7826,.T.);
#11235=ORIENTED_EDGE('',*,*,#7811,.T.);
#11236=ORIENTED_EDGE('',*,*,#7791,.F.);
#11237=ORIENTED_EDGE('',*,*,#7810,.T.);
#11238=ORIENTED_EDGE('',*,*,#7814,.T.);
#11318=CONICAL_SURFACE('',#13516,20.6,0.785398163397443);
#11319=CONICAL_SURFACE('',#13520,20.,0.785398163397457);
#11320=CONICAL_SURFACE('',#13545,7.,1.05840686648416);
#11321=CONICAL_SURFACE('',#13549,15.,1.05840686648416);
#11322=CONICAL_SURFACE('',#13560,4.90000000000001,0.785398163397295);
#11323=CONICAL_SURFACE('',#13563,4.7,0.785398163397478);
#11324=CONICAL_SURFACE('',#13610,4.35000000000001,0.785398163397442);
#11898=ADVANCED_FACE('',(#1816),#11318,.F.);
#11899=ADVANCED_FACE('',(#1817),#11319,.F.);
#11900=ADVANCED_FACE('',(#1818),#846,.T.);
#11901=ADVANCED_FACE('',(#1819),#847,.F.);
#11902=ADVANCED_FACE('',(#1820),#848,.T.);
#11903=ADVANCED_FACE('',(#1821),#849,.F.);
#11904=ADVANCED_FACE('',(#1822),#1184,.F.);
#11905=ADVANCED_FACE('',(#1823),#11320,.T.);
#11906=ADVANCED_FACE('',(#1824),#1185,.F.);
#11907=ADVANCED_FACE('',(#1825),#11321,.T.);
#11908=ADVANCED_FACE('',(#1826),#1186,.F.);
#11909=ADVANCED_FACE('',(#1827),#1187,.T.);
#11910=ADVANCED_FACE('',(#1828,#433),#701,.T.);
#11911=ADVANCED_FACE('',(#1829,#434),#702,.F.);
#11912=ADVANCED_FACE('',(#1830,#435),#703,.T.);
#11913=ADVANCED_FACE('',(#1831,#436),#704,.T.);
#11914=ADVANCED_FACE('',(#1832,#437),#705,.F.);
#11915=ADVANCED_FACE('',(#1833,#438),#706,.T.);
#11916=ADVANCED_FACE('',(#1834),#11322,.T.);
#11917=ADVANCED_FACE('',(#1835),#11323,.T.);
#11918=ADVANCED_FACE('',(#1836),#1188,.T.);
#11919=ADVANCED_FACE('',(#1837),#707,.T.);
#11920=ADVANCED_FACE('',(#1838),#708,.T.);
#11921=ADVANCED_FACE('',(#1839),#1189,.T.);
#11922=ADVANCED_FACE('',(#1840),#1190,.T.);
#11923=ADVANCED_FACE('',(#1841),#1191,.T.);
#11924=ADVANCED_FACE('',(#1842),#1192,.T.);
#11925=ADVANCED_FACE('',(#1843),#1193,.T.);
#11926=ADVANCED_FACE('',(#1844),#1194,.T.);
#11927=ADVANCED_FACE('',(#1845),#1195,.T.);
#11928=ADVANCED_FACE('',(#1846),#1196,.T.);
#11929=ADVANCED_FACE('',(#1847),#1197,.T.);
#11930=ADVANCED_FACE('',(#1848),#1198,.T.);
#11931=ADVANCED_FACE('',(#1849),#1199,.T.);
#11932=ADVANCED_FACE('',(#1850),#1200,.T.);
#11933=ADVANCED_FACE('',(#1851),#1201,.T.);
#11934=ADVANCED_FACE('',(#1852),#1202,.T.);
#11935=ADVANCED_FACE('',(#1853),#1203,.T.);
#11936=ADVANCED_FACE('',(#1854),#1204,.T.);
#11937=ADVANCED_FACE('',(#1855),#1205,.T.);
#11938=ADVANCED_FACE('',(#1856),#1206,.T.);
#11939=ADVANCED_FACE('',(#1857),#1207,.T.);
#11940=ADVANCED_FACE('',(#1858),#1208,.T.);
#11941=ADVANCED_FACE('',(#1859),#1209,.T.);
#11942=ADVANCED_FACE('',(#1860),#1210,.T.);
#11943=ADVANCED_FACE('',(#1861),#1211,.T.);
#11944=ADVANCED_FACE('',(#1862),#1212,.T.);
#11945=ADVANCED_FACE('',(#1863),#1213,.T.);
#11946=ADVANCED_FACE('',(#1864),#1214,.T.);
#11947=ADVANCED_FACE('',(#1865),#1215,.T.);
#11948=ADVANCED_FACE('',(#1866),#1216,.F.);
#11949=ADVANCED_FACE('',(#1867),#1217,.F.);
#11950=ADVANCED_FACE('',(#1868),#11324,.T.);
#11951=ADVANCED_FACE('',(#1869),#709,.T.);
#11952=ADVANCED_FACE('',(#1870),#710,.T.);
#11953=ADVANCED_FACE('',(#1871,#439),#711,.T.);
#11954=ADVANCED_FACE('',(#1872,#440),#712,.T.);
#11955=ADVANCED_FACE('',(#1873),#713,.T.);
#11956=ADVANCED_FACE('',(#1874,#441),#714,.T.);
#11957=ADVANCED_FACE('',(#1875,#442),#715,.T.);
#11958=ADVANCED_FACE('',(#1876),#716,.T.);
#11959=ADVANCED_FACE('',(#1877),#717,.T.);
#11960=ADVANCED_FACE('',(#1878),#718,.F.);
#11961=ADVANCED_FACE('',(#1879),#719,.F.);
#11962=ADVANCED_FACE('',(#1880),#720,.F.);
#11963=ADVANCED_FACE('',(#1881),#1218,.T.);
#11964=ADVANCED_FACE('',(#1882),#1219,.T.);
#11965=ADVANCED_FACE('',(#1883),#721,.F.);
#11966=ADVANCED_FACE('',(#1884),#722,.F.);
#11967=ADVANCED_FACE('',(#1885,#443),#723,.T.);
#11968=ADVANCED_FACE('',(#1886),#724,.T.);
#11969=ADVANCED_FACE('',(#1887),#725,.F.);
#11970=ADVANCED_FACE('',(#1888),#323,.T.);
#11971=ADVANCED_FACE('',(#1889),#1220,.T.);
#11972=ADVANCED_FACE('',(#1890),#324,.T.);
#11973=ADVANCED_FACE('',(#1891),#1221,.T.);
#11974=ADVANCED_FACE('',(#1892),#1222,.T.);
#11975=ADVANCED_FACE('',(#1893),#1223,.F.);
#11976=ADVANCED_FACE('',(#1894),#1224,.F.);
#11977=ADVANCED_FACE('',(#1895),#1225,.F.);
#11978=ADVANCED_FACE('',(#1896),#1226,.F.);
#11979=ADVANCED_FACE('',(#1897),#1227,.F.);
#11980=ADVANCED_FACE('',(#1898),#1228,.F.);
#11981=ADVANCED_FACE('',(#1899),#1229,.F.);
#11982=ADVANCED_FACE('',(#1900),#1230,.F.);
#11983=ADVANCED_FACE('',(#1901),#1231,.F.);
#11984=ADVANCED_FACE('',(#1902),#1232,.F.);
#11985=ADVANCED_FACE('',(#1903),#1233,.F.);
#11986=ADVANCED_FACE('',(#1904),#1234,.F.);
#11987=ADVANCED_FACE('',(#1905),#1235,.F.);
#11988=ADVANCED_FACE('',(#1906),#1236,.F.);
#11989=ADVANCED_FACE('',(#1907),#1237,.F.);
#11990=ADVANCED_FACE('',(#1908),#1238,.F.);
#11991=ADVANCED_FACE('',(#1909),#1239,.F.);
#11992=ADVANCED_FACE('',(#1910),#1240,.F.);
#11993=ADVANCED_FACE('',(#1911),#1241,.F.);
#11994=ADVANCED_FACE('',(#1912),#1242,.T.);
#11995=ADVANCED_FACE('',(#1913,#444),#726,.T.);
#11996=ADVANCED_FACE('',(#1914,#445),#727,.T.);
#11997=ADVANCED_FACE('',(#1915,#446),#728,.F.);
#11998=ADVANCED_FACE('',(#1916),#729,.F.);
#11999=ADVANCED_FACE('',(#1917),#730,.F.);
#12000=ADVANCED_FACE('',(#1918),#731,.F.);
#12001=ADVANCED_FACE('',(#1919),#732,.F.);
#12002=ADVANCED_FACE('',(#1920),#733,.F.);
#12003=ADVANCED_FACE('',(#1921),#734,.F.);
#12004=ADVANCED_FACE('',(#1922),#735,.F.);
#12005=ADVANCED_FACE('',(#1923),#1243,.F.);
#12006=ADVANCED_FACE('',(#1924),#325,.T.);
#12007=ADVANCED_FACE('',(#1925),#326,.T.);
#12008=ADVANCED_FACE('',(#1926),#736,.T.);
#12009=ADVANCED_FACE('',(#1927),#737,.T.);
#12010=ADVANCED_FACE('',(#1928),#738,.T.);
#12011=ADVANCED_FACE('',(#1929),#739,.T.);
#12012=ADVANCED_FACE('',(#1930),#740,.T.);
#12013=ADVANCED_FACE('',(#1931),#741,.T.);
#12049=CLOSED_SHELL('',(#11898,#11899,#11900,#11901,#11902,#11903,#11904,
#11905,#11906,#11907,#11908,#11909,#11910,#11911,#11912,#11913,#11914,#11915));
#12050=CLOSED_SHELL('',(#11916,#11917,#11918,#11919,#11920));
#12051=CLOSED_SHELL('',(#11921,#11922,#11923,#11924,#11925,#11926,#11927,
#11928,#11929,#11930,#11931,#11932,#11933,#11934,#11935,#11936,#11937,#11938,
#11939,#11940,#11941,#11942,#11943,#11944,#11945,#11946,#11947,#11948,#11949,
#11950,#11951,#11952,#11953,#11954,#11955,#11956,#11957,#11958,#11959,#11960,
#11961,#11962,#11963,#11964,#11965,#11966,#11967,#11968,#11969,#11970,#11971,
#11972,#11973,#11974,#11975,#11976));
#12052=CLOSED_SHELL('',(#11977,#11978,#11979,#11980,#11981,#11982,#11983,
#11984,#11985,#11986,#11987,#11988,#11989,#11990,#11991,#11992,#11993,#11994,
#11995,#11996,#11997,#11998,#11999,#12000,#12001,#12002,#12003,#12004,#12005,
#12006,#12007,#12008,#12009,#12010,#12011,#12012,#12013));
#13515=AXIS2_PLACEMENT_3D('',#23312,#16845,#16846);
#13516=AXIS2_PLACEMENT_3D('',#23313,#16847,#16848);
#13517=AXIS2_PLACEMENT_3D('',#23316,#16849,#16850);
#13518=AXIS2_PLACEMENT_3D('',#23317,#16851,#16852);
#13519=AXIS2_PLACEMENT_3D('',#23320,#16854,#16855);
#13520=AXIS2_PLACEMENT_3D('',#23321,#16856,#16857);
#13521=AXIS2_PLACEMENT_3D('',#23323,#16858,#16859);
#13522=AXIS2_PLACEMENT_3D('',#23326,#16861,#16862);
#13523=AXIS2_PLACEMENT_3D('',#23327,#16863,#16864);
#13524=AXIS2_PLACEMENT_3D('',#23329,#16865,#16866);
#13525=AXIS2_PLACEMENT_3D('',#23331,#16867,#16868);
#13526=AXIS2_PLACEMENT_3D('',#23333,#16869,#16870);
#13527=AXIS2_PLACEMENT_3D('',#23334,#16871,#16872);
#13528=AXIS2_PLACEMENT_3D('',#23335,#16873,#16874);
#13529=AXIS2_PLACEMENT_3D('',#23337,#16875,#16876);
#13530=AXIS2_PLACEMENT_3D('',#23339,#16877,#16878);
#13531=AXIS2_PLACEMENT_3D('',#23340,#16879,#16880);
#13532=AXIS2_PLACEMENT_3D('',#23341,#16881,#16882);
#13533=AXIS2_PLACEMENT_3D('',#23344,#16883,#16884);
#13534=AXIS2_PLACEMENT_3D('',#23345,#16885,#16886);
#13535=AXIS2_PLACEMENT_3D('',#23347,#16887,#16888);
#13536=AXIS2_PLACEMENT_3D('',#23348,#16889,#16890);
#13537=AXIS2_PLACEMENT_3D('',#23349,#16891,#16892);
#13538=AXIS2_PLACEMENT_3D('',#23351,#16893,#16894);
#13539=AXIS2_PLACEMENT_3D('',#23353,#16895,#16896);
#13540=AXIS2_PLACEMENT_3D('',#23355,#16897,#16898);
#13541=AXIS2_PLACEMENT_3D('',#23356,#16899,#16900);
#13542=AXIS2_PLACEMENT_3D('',#23357,#16901,#16902);
#13543=AXIS2_PLACEMENT_3D('',#23359,#16903,#16904);
#13544=AXIS2_PLACEMENT_3D('',#23362,#16906,#16907);
#13545=AXIS2_PLACEMENT_3D('',#23363,#16908,#16909);
#13546=AXIS2_PLACEMENT_3D('',#23365,#16910,#16911);
#13547=AXIS2_PLACEMENT_3D('',#23368,#16913,#16914);
#13548=AXIS2_PLACEMENT_3D('',#23369,#16915,#16916);
#13549=AXIS2_PLACEMENT_3D('',#23371,#16918,#16919);
#13550=AXIS2_PLACEMENT_3D('',#23373,#16920,#16921);
#13551=AXIS2_PLACEMENT_3D('',#23376,#16923,#16924);
#13552=AXIS2_PLACEMENT_3D('',#23377,#16925,#16926);
#13553=AXIS2_PLACEMENT_3D('',#23379,#16928,#16929);
#13554=AXIS2_PLACEMENT_3D('',#23381,#16931,#16932);
#13555=AXIS2_PLACEMENT_3D('',#23382,#16933,#16934);
#13556=AXIS2_PLACEMENT_3D('',#23383,#16935,#16936);
#13557=AXIS2_PLACEMENT_3D('',#23384,#16937,#16938);
#13558=AXIS2_PLACEMENT_3D('',#23385,#16939,#16940);
#13559=AXIS2_PLACEMENT_3D('',#23386,#16941,#16942);
#13560=AXIS2_PLACEMENT_3D('',#23387,#16943,#16944);
#13561=AXIS2_PLACEMENT_3D('',#23389,#16945,#16946);
#13562=AXIS2_PLACEMENT_3D('',#23392,#16948,#16949);
#13563=AXIS2_PLACEMENT_3D('',#23393,#16950,#16951);
#13564=AXIS2_PLACEMENT_3D('',#23396,#16952,#16953);
#13565=AXIS2_PLACEMENT_3D('',#23397,#16954,#16955);
#13566=AXIS2_PLACEMENT_3D('',#23400,#16957,#16958);
#13567=AXIS2_PLACEMENT_3D('',#23401,#16959,#16960);
#13568=AXIS2_PLACEMENT_3D('',#23403,#16962,#16963);
#13569=AXIS2_PLACEMENT_3D('',#23404,#16964,#16965);
#13570=AXIS2_PLACEMENT_3D('',#23405,#16966,#16967);
#13571=AXIS2_PLACEMENT_3D('',#23430,#16970,#16971);
#13572=AXIS2_PLACEMENT_3D('',#23468,#16973,#16974);
#13573=AXIS2_PLACEMENT_3D('',#23506,#16976,#16977);
#13574=AXIS2_PLACEMENT_3D('',#23544,#16979,#16980);
#13575=AXIS2_PLACEMENT_3D('',#23582,#16982,#16983);
#13576=AXIS2_PLACEMENT_3D('',#23620,#16985,#16986);
#13577=AXIS2_PLACEMENT_3D('',#23658,#16988,#16989);
#13578=AXIS2_PLACEMENT_3D('',#23696,#16991,#16992);
#13579=AXIS2_PLACEMENT_3D('',#23734,#16994,#16995);
#13580=AXIS2_PLACEMENT_3D('',#23772,#16997,#16998);
#13581=AXIS2_PLACEMENT_3D('',#23810,#17000,#17001);
#13582=AXIS2_PLACEMENT_3D('',#23848,#17003,#17004);
#13583=AXIS2_PLACEMENT_3D('',#23886,#17006,#17007);
#13584=AXIS2_PLACEMENT_3D('',#23929,#17010,#17011);
#13585=AXIS2_PLACEMENT_3D('',#23989,#17013,#17014);
#13586=AXIS2_PLACEMENT_3D('',#24065,#17016,#17017);
#13587=AXIS2_PLACEMENT_3D('',#24143,#17019,#17020);
#13588=AXIS2_PLACEMENT_3D('',#24219,#17022,#17023);
#13589=AXIS2_PLACEMENT_3D('',#24295,#17025,#17026);
#13590=AXIS2_PLACEMENT_3D('',#24371,#17028,#17029);
#13591=AXIS2_PLACEMENT_3D('',#24447,#17031,#17032);
#13592=AXIS2_PLACEMENT_3D('',#24523,#17034,#17035);
#13593=AXIS2_PLACEMENT_3D('',#24601,#17037,#17038);
#13594=AXIS2_PLACEMENT_3D('',#24677,#17040,#17041);
#13595=AXIS2_PLACEMENT_3D('',#24753,#17043,#17044);
#13596=AXIS2_PLACEMENT_3D('',#24829,#17046,#17047);
#13597=AXIS2_PLACEMENT_3D('',#24844,#17048,#17049);
#13598=AXIS2_PLACEMENT_3D('',#24853,#17050,#17051);
#13599=AXIS2_PLACEMENT_3D('',#24855,#17052,#17053);
#13600=AXIS2_PLACEMENT_3D('',#24859,#17055,#17056);
#13601=AXIS2_PLACEMENT_3D('',#24861,#17057,#17058);
#13602=AXIS2_PLACEMENT_3D('',#24863,#17059,#17060);
#13603=AXIS2_PLACEMENT_3D('',#24864,#17061,#17062);
#13604=AXIS2_PLACEMENT_3D('',#24865,#17063,#17064);
#13605=AXIS2_PLACEMENT_3D('',#24867,#17065,#17066);
#13606=AXIS2_PLACEMENT_3D('',#24870,#17068,#17069);
#13607=AXIS2_PLACEMENT_3D('',#24871,#17070,#17071);
#13608=AXIS2_PLACEMENT_3D('',#24873,#17072,#17073);
#13609=AXIS2_PLACEMENT_3D('',#24876,#17075,#17076);
#13610=AXIS2_PLACEMENT_3D('',#24877,#17077,#17078);
#13611=AXIS2_PLACEMENT_3D('',#24893,#17080,#17081);
#13612=AXIS2_PLACEMENT_3D('',#24922,#17082,#17083);
#13613=AXIS2_PLACEMENT_3D('',#24935,#17084,#17085);
#13614=AXIS2_PLACEMENT_3D('',#24941,#17089,#17090);
#13615=AXIS2_PLACEMENT_3D('',#24945,#17093,#17094);
#13616=AXIS2_PLACEMENT_3D('',#24953,#17098,#17099);
#13617=AXIS2_PLACEMENT_3D('',#24954,#17100,#17101);
#13618=AXIS2_PLACEMENT_3D('',#24962,#17105,#17106);
#13619=AXIS2_PLACEMENT_3D('',#24963,#17107,#17108);
#13620=AXIS2_PLACEMENT_3D('',#24967,#17111,#17112);
#13621=AXIS2_PLACEMENT_3D('',#24975,#17116,#17117);
#13622=AXIS2_PLACEMENT_3D('',#24976,#17118,#17119);
#13623=AXIS2_PLACEMENT_3D('',#24984,#17123,#17124);
#13624=AXIS2_PLACEMENT_3D('',#24985,#17125,#17126);
#13625=AXIS2_PLACEMENT_3D('',#24994,#17131,#17132);
#13626=AXIS2_PLACEMENT_3D('',#24997,#17134,#17135);
#13627=AXIS2_PLACEMENT_3D('',#24999,#17136,#17137);
#13628=AXIS2_PLACEMENT_3D('',#25001,#17139,#17140);
#13629=AXIS2_PLACEMENT_3D('',#25003,#17141,#17142);
#13630=AXIS2_PLACEMENT_3D('',#25007,#17145,#17146);
#13631=AXIS2_PLACEMENT_3D('',#25008,#17147,#17148);
#13632=AXIS2_PLACEMENT_3D('',#25009,#17149,#17150);
#13633=AXIS2_PLACEMENT_3D('',#25010,#17151,#17152);
#13634=AXIS2_PLACEMENT_3D('',#25012,#17154,#17155);
#13635=AXIS2_PLACEMENT_3D('',#25013,#17156,#17157);
#13636=AXIS2_PLACEMENT_3D('',#25015,#17159,#17160);
#13637=AXIS2_PLACEMENT_3D('',#25016,#17161,#17162);
#13638=AXIS2_PLACEMENT_3D('',#25017,#17163,#17164);
#13639=AXIS2_PLACEMENT_3D('',#25020,#17167,#17168);
#13640=AXIS2_PLACEMENT_3D('',#25021,#17169,#17170);
#13641=AXIS2_PLACEMENT_3D('',#25022,#17171,#17172);
#13642=AXIS2_PLACEMENT_3D('',#25023,#17173,#17174);
#13643=AXIS2_PLACEMENT_3D('',#25024,#17175,#17176);
#13644=AXIS2_PLACEMENT_3D('',#25025,#17177,#17178);
#13645=AXIS2_PLACEMENT_3D('',#25026,#17179,#17180);
#13646=AXIS2_PLACEMENT_3D('',#25027,#17181,#17182);
#13647=AXIS2_PLACEMENT_3D('',#25028,#17183,#17184);
#13648=AXIS2_PLACEMENT_3D('',#25488,#17187,#17188);
#13649=AXIS2_PLACEMENT_3D('',#25950,#17189,#17190);
#13650=AXIS2_PLACEMENT_3D('',#25951,#17191,#17192);
#13651=AXIS2_PLACEMENT_3D('',#25952,#17193,#17194);
#13652=AXIS2_PLACEMENT_3D('',#25953,#17195,#17196);
#13653=AXIS2_PLACEMENT_3D('',#25954,#17197,#17198);
#13654=AXIS2_PLACEMENT_3D('',#25975,#17200,#17201);
#13655=AXIS2_PLACEMENT_3D('',#25993,#17202,#17203);
#13656=AXIS2_PLACEMENT_3D('',#26031,#17205,#17206);
#13657=AXIS2_PLACEMENT_3D('',#26069,#17208,#17209);
#13658=AXIS2_PLACEMENT_3D('',#26107,#17211,#17212);
#13659=AXIS2_PLACEMENT_3D('',#26145,#17214,#17215);
#13660=AXIS2_PLACEMENT_3D('',#26183,#17217,#17218);
#13661=AXIS2_PLACEMENT_3D('',#26221,#17220,#17221);
#13662=AXIS2_PLACEMENT_3D('',#26246,#17224,#17225);
#13663=AXIS2_PLACEMENT_3D('',#26294,#17229,#17230);
#13664=AXIS2_PLACEMENT_3D('',#26331,#17231,#17232);
#13665=AXIS2_PLACEMENT_3D('',#26409,#17234,#17235);
#13666=AXIS2_PLACEMENT_3D('',#26485,#17237,#17238);
#13667=AXIS2_PLACEMENT_3D('',#26561,#17240,#17241);
#13668=AXIS2_PLACEMENT_3D('',#26637,#17243,#17244);
#13669=AXIS2_PLACEMENT_3D('',#26713,#17246,#17247);
#13670=AXIS2_PLACEMENT_3D('',#26789,#17249,#17250);
#13671=AXIS2_PLACEMENT_3D('',#26807,#17252,#17253);
#13672=AXIS2_PLACEMENT_3D('',#26828,#17254,#17255);
#13673=AXIS2_PLACEMENT_3D('',#26901,#17256,#17257);
#13674=AXIS2_PLACEMENT_3D('',#26903,#17258,#17259);
#13675=AXIS2_PLACEMENT_3D('',#26906,#17261,#17262);
#13676=AXIS2_PLACEMENT_3D('',#26907,#17263,#17264);
#13677=AXIS2_PLACEMENT_3D('',#26960,#17277,#17278);
#13678=AXIS2_PLACEMENT_3D('',#26973,#17285,#17286);
#13679=AXIS2_PLACEMENT_3D('',#26974,#17287,#17288);
#13680=AXIS2_PLACEMENT_3D('',#26981,#17293,#17294);
#13681=AXIS2_PLACEMENT_3D('',#26986,#17298,#17299);
#13682=AXIS2_PLACEMENT_3D('',#26991,#17303,#17304);
#13683=AXIS2_PLACEMENT_3D('',#26996,#17308,#17309);
#13684=AXIS2_PLACEMENT_3D('',#27001,#17313,#17314);
#13685=AXIS2_PLACEMENT_3D('',#27004,#17317,#17318);
#13686=AXIS2_PLACEMENT_3D('',#27007,#17321,#17322);
#13687=AXIS2_PLACEMENT_3D('',#27686,#17323,#17324);
#13688=AXIS2_PLACEMENT_3D('',#27687,#17325,#17326);
#13689=AXIS2_PLACEMENT_3D('',#27688,#17327,#17328);
#13690=AXIS2_PLACEMENT_3D('',#27689,#17329,#17330);
#13691=AXIS2_PLACEMENT_3D('',#27690,#17331,#17332);
#13692=AXIS2_PLACEMENT_3D('',#27691,#17333,#17334);
#16845=DIRECTION('axis',(0.,0.,1.));
#16846=DIRECTION('refdir',(1.,0.,0.));
#16847=DIRECTION('center_axis',(-0.223538897454057,-2.77555756156289E-16,
0.974695009387565));
#16848=DIRECTION('ref_axis',(0.945835712345015,-0.241537608024065,0.216920236867866));
#16849=DIRECTION('center_axis',(-0.223538897454057,-2.77555756156289E-16,
0.974695009387565));
#16850=DIRECTION('ref_axis',(-0.945835712345015,0.241537608024065,-0.216920236867866));
#16851=DIRECTION('center_axis',(-0.223538897454057,-2.77555756156289E-16,
0.974695009387565));
#16852=DIRECTION('ref_axis',(-0.945835712345015,0.241537608024065,-0.216920236867866));
#16853=DIRECTION('',(-0.826872716336294,0.170792880545394,0.535827680260777));
#16854=DIRECTION('center_axis',(0.223538897454057,2.77555756156289E-16,
-0.974695009387565));
#16855=DIRECTION('ref_axis',(-0.945835712345015,0.241537608024065,-0.216920236867866));
#16856=DIRECTION('center_axis',(0.223538897454057,2.77555756156289E-16,
-0.974695009387565));
#16857=DIRECTION('ref_axis',(-0.945835712345015,0.241537608024065,-0.216920236867866));
#16858=DIRECTION('center_axis',(0.223538897454057,2.77555756156289E-16,
-0.974695009387565));
#16859=DIRECTION('ref_axis',(-0.945835712345015,0.241537608024065,-0.216920236867866));
#16860=DIRECTION('',(0.826872716336301,-0.170792880545396,-0.535827680260765));
#16861=DIRECTION('center_axis',(-0.223538897454057,-2.77555756156289E-16,
0.974695009387565));
#16862=DIRECTION('ref_axis',(-0.945835712345015,0.241537608024065,-0.216920236867866));
#16863=DIRECTION('center_axis',(0.223538897454057,2.77555756156289E-16,
-0.974695009387565));
#16864=DIRECTION('ref_axis',(-0.945835712345015,0.241537608024065,-0.216920236867868));
#16865=DIRECTION('center_axis',(0.223538897454057,2.77555756156289E-16,
-0.974695009387565));
#16866=DIRECTION('ref_axis',(-0.945835712345015,0.241537608024065,-0.216920236867866));
#16867=DIRECTION('center_axis',(-0.235425501120466,-0.970391459108134,-0.0539930505913901));
#16868=DIRECTION('ref_axis',(0.945835712345015,-0.241537608024065,0.216920236867867));
#16869=DIRECTION('center_axis',(-0.223538897454057,-2.77555756156289E-16,
0.974695009387565));
#16870=DIRECTION('ref_axis',(-0.945835712345015,0.241537608024065,-0.216920236867866));
#16871=DIRECTION('center_axis',(-0.223538897454057,-2.77555756156289E-16,
0.974695009387565));
#16872=DIRECTION('ref_axis',(-0.945835712345015,0.241537608024065,-0.216920236867866));
#16873=DIRECTION('center_axis',(0.223538897454057,2.77555756156289E-16,
-0.974695009387565));
#16874=DIRECTION('ref_axis',(-0.945835712345015,0.241537608024065,-0.216920236867867));
#16875=DIRECTION('center_axis',(0.223538897454057,2.77555756156289E-16,
-0.974695009387565));
#16876=DIRECTION('ref_axis',(-0.945835712345015,0.241537608024065,-0.216920236867866));
#16877=DIRECTION('center_axis',(0.235425501120466,0.970391459108134,0.05399305059139));
#16878=DIRECTION('ref_axis',(0.945835712345015,-0.241537608024065,0.216920236867867));
#16879=DIRECTION('center_axis',(-0.223538897454057,-2.77555756156289E-16,
0.974695009387565));
#16880=DIRECTION('ref_axis',(-0.945835712345015,0.241537608024065,-0.216920236867866));
#16881=DIRECTION('center_axis',(0.223538897454057,2.77555756156289E-16,
-0.974695009387565));
#16882=DIRECTION('ref_axis',(-0.945835712345015,0.241537608024065,-0.216920236867868));
#16883=DIRECTION('center_axis',(0.223538897454057,2.77555756156289E-16,
-0.974695009387565));
#16884=DIRECTION('ref_axis',(-0.945835712345015,0.241537608024065,-0.216920236867866));
#16885=DIRECTION('center_axis',(0.223538897454057,2.77555756156289E-16,
-0.974695009387565));
#16886=DIRECTION('ref_axis',(-0.945835712345015,0.241537608024065,-0.216920236867866));
#16887=DIRECTION('center_axis',(-0.235425501120466,-0.970391459108134,-0.0539930505913901));
#16888=DIRECTION('ref_axis',(0.945835712345015,-0.241537608024065,0.216920236867867));
#16889=DIRECTION('center_axis',(-0.223538897454057,-2.77555756156289E-16,
0.974695009387565));
#16890=DIRECTION('ref_axis',(-0.945835712345015,0.241537608024065,-0.216920236867866));
#16891=DIRECTION('center_axis',(-0.223538897454057,-2.77555756156289E-16,
0.974695009387565));
#16892=DIRECTION('ref_axis',(0.945835712345015,-0.241537608024065,0.216920236867867));
#16893=DIRECTION('center_axis',(-0.223538897454057,-2.77555756156289E-16,
0.974695009387565));
#16894=DIRECTION('ref_axis',(0.945835712345015,-0.241537608024065,0.216920236867866));
#16895=DIRECTION('center_axis',(0.235425501120466,0.970391459108134,0.0539930505913899));
#16896=DIRECTION('ref_axis',(-0.945835712345015,0.241537608024065,-0.216920236867867));
#16897=DIRECTION('center_axis',(0.223538897454057,2.77555756156289E-16,
-0.974695009387565));
#16898=DIRECTION('ref_axis',(0.945835712345015,-0.241537608024065,0.216920236867866));
#16899=DIRECTION('center_axis',(0.223538897454057,2.77555756156289E-16,
-0.974695009387565));
#16900=DIRECTION('ref_axis',(0.945835712345015,-0.241537608024065,0.216920236867866));
#16901=DIRECTION('center_axis',(0.223538897454057,2.77555756156289E-16,
-0.974695009387565));
#16902=DIRECTION('ref_axis',(-0.945835712345015,0.241537608024065,-0.216920236867866));
#16903=DIRECTION('center_axis',(-0.223538897454057,-2.77555756156289E-16,
0.974695009387565));
#16904=DIRECTION('ref_axis',(-0.945835712345015,0.241537608024064,-0.216920236867866));
#16905=DIRECTION('',(0.223538897454057,2.77555756156289E-16,-0.974695009387565));
#16906=DIRECTION('center_axis',(0.223538897454057,2.77555756156289E-16,
-0.974695009387565));
#16907=DIRECTION('ref_axis',(-0.945835712345015,0.241537608024065,-0.216920236867866));
#16908=DIRECTION('center_axis',(-0.223538897454057,-2.77555756156289E-16,
0.974695009387565));
#16909=DIRECTION('ref_axis',(0.945835712345015,-0.241537608024066,0.216920236867866));
#16910=DIRECTION('center_axis',(0.223538897454057,2.77555756156289E-16,
-0.974695009387565));
#16911=DIRECTION('ref_axis',(-0.945835712345015,0.241537608024065,-0.216920236867866));
#16912=DIRECTION('',(0.933959725990609,-0.210518270449354,-0.288792811604722));
#16913=DIRECTION('center_axis',(0.223538897454057,2.77555756156289E-16,
-0.974695009387565));
#16914=DIRECTION('ref_axis',(-0.945835712345015,0.241537608024066,-0.216920236867866));
#16915=DIRECTION('center_axis',(0.223538897454057,2.77555756156289E-16,
-0.974695009387565));
#16916=DIRECTION('ref_axis',(-0.945835712345015,0.241537608024065,-0.216920236867866));
#16917=DIRECTION('',(0.223538897454057,2.77555756156289E-16,-0.974695009387564));
#16918=DIRECTION('center_axis',(0.223538897454057,2.77555756156289E-16,
-0.974695009387565));
#16919=DIRECTION('ref_axis',(-0.945835712345015,0.241537608024065,-0.216920236867866));
#16920=DIRECTION('center_axis',(0.223538897454057,2.77555756156289E-16,
-0.974695009387565));
#16921=DIRECTION('ref_axis',(-0.945835712345015,0.241537608024065,-0.216920236867866));
#16922=DIRECTION('',(-0.933959725990608,0.210518270449354,0.288792811604722));
#16923=DIRECTION('center_axis',(0.223538897454057,2.77555756156289E-16,
-0.974695009387565));
#16924=DIRECTION('ref_axis',(-0.945835712345015,0.241537608024066,-0.216920236867866));
#16925=DIRECTION('center_axis',(0.223538897454057,2.77555756156289E-16,
-0.974695009387565));
#16926=DIRECTION('ref_axis',(-0.945835712345015,0.241537608024065,-0.216920236867866));
#16927=DIRECTION('',(0.223538897454057,2.77555756156289E-16,-0.974695009387564));
#16928=DIRECTION('center_axis',(-0.223538897454057,-2.77555756156289E-16,
0.974695009387565));
#16929=DIRECTION('ref_axis',(0.945835712345015,-0.241537608024065,0.216920236867866));
#16930=DIRECTION('',(0.223538897454057,2.77555756156289E-16,-0.974695009387564));
#16931=DIRECTION('center_axis',(0.223538897454057,2.63677968348475E-16,
-0.974695009387565));
#16932=DIRECTION('ref_axis',(-0.945835712345015,0.241537608024065,-0.216920236867866));
#16933=DIRECTION('center_axis',(0.223538897454057,2.63677968348475E-16,
-0.974695009387565));
#16934=DIRECTION('ref_axis',(-0.945835712345015,0.241537608024065,-0.216920236867866));
#16935=DIRECTION('center_axis',(-0.223538897454057,-2.63677968348475E-16,
0.974695009387565));
#16936=DIRECTION('ref_axis',(0.945835712345015,-0.241537608024065,0.216920236867866));
#16937=DIRECTION('center_axis',(0.223538897454057,2.63677968348475E-16,
-0.974695009387565));
#16938=DIRECTION('ref_axis',(-0.945835712345015,0.241537608024065,-0.216920236867866));
#16939=DIRECTION('center_axis',(0.223538897454057,2.63677968348475E-16,
-0.974695009387565));
#16940=DIRECTION('ref_axis',(-0.945835712345015,0.241537608024065,-0.216920236867866));
#16941=DIRECTION('center_axis',(0.223538897454057,2.63677968348475E-16,
-0.974695009387565));
#16942=DIRECTION('ref_axis',(-0.945835712345015,0.241537608024065,-0.216920236867866));
#16943=DIRECTION('center_axis',(-0.223538897454133,0.,0.974695009387547));
#16944=DIRECTION('ref_axis',(0.974695009387547,0.,0.223538897454133));
#16945=DIRECTION('center_axis',(-0.223538897454133,0.,0.974695009387547));
#16946=DIRECTION('ref_axis',(-0.974695009387547,0.,-0.223538897454133));
#16947=DIRECTION('',(0.84727932097532,8.65956056235361E-17,-0.531147580477968));
#16948=DIRECTION('center_axis',(0.223538897454057,1.10873856701773E-16,
-0.974695009387565));
#16949=DIRECTION('ref_axis',(-0.974695009387564,4.77630626208034E-31,-0.223538897454057));
#16950=DIRECTION('center_axis',(0.223538897454062,0.,-0.974695009387563));
#16951=DIRECTION('ref_axis',(-0.974695009387563,0.,-0.223538897454062));
#16952=DIRECTION('center_axis',(0.223538897454062,0.,-0.974695009387563));
#16953=DIRECTION('ref_axis',(0.974695009387563,0.,0.223538897454062));
#16954=DIRECTION('center_axis',(0.223538897454062,0.,-0.974695009387563));
#16955=DIRECTION('ref_axis',(0.974695009387563,0.,0.223538897454062));
#16956=DIRECTION('',(-0.847279320975379,8.65956056235519E-17,0.531147580477875));
#16957=DIRECTION('center_axis',(-0.223538897454057,1.56006678063889E-16,
0.974695009387565));
#16958=DIRECTION('ref_axis',(0.974695009387565,-2.09541177949331E-31,0.223538897454057));
#16959=DIRECTION('center_axis',(-0.223538897454057,1.56006678063889E-16,
0.974695009387565));
#16960=DIRECTION('ref_axis',(0.974695009387564,6.34786509670033E-31,0.223538897454057));
#16961=DIRECTION('',(0.223538897454057,-1.56006678063889E-16,-0.974695009387564));
#16962=DIRECTION('center_axis',(0.223538897454057,1.10873856701773E-16,
-0.974695009387565));
#16963=DIRECTION('ref_axis',(-0.974695009387565,1.39180436012088E-16,-0.223538897454057));
#16964=DIRECTION('center_axis',(-0.223538897454057,1.56006678063889E-16,
0.974695009387565));
#16965=DIRECTION('ref_axis',(0.974695009387565,0.,0.223538897454057));
#16966=DIRECTION('center_axis',(0.,1.,0.));
#16967=DIRECTION('ref_axis',(0.223538897454053,0.,-0.974695009387565));
#16968=DIRECTION('',(0.,-1.,0.));
#16969=DIRECTION('',(-1.10873856701774E-16,-1.,-1.39180436012088E-16));
#16970=DIRECTION('center_axis',(0.,1.,0.));
#16971=DIRECTION('ref_axis',(0.223538897454053,0.,-0.974695009387565));
#16972=DIRECTION('',(0.,-1.,0.));
#16973=DIRECTION('center_axis',(0.,1.,0.));
#16974=DIRECTION('ref_axis',(0.223538897454053,0.,-0.974695009387565));
#16975=DIRECTION('',(0.,-1.,0.));
#16976=DIRECTION('center_axis',(0.,1.,0.));
#16977=DIRECTION('ref_axis',(0.223538897454053,0.,-0.974695009387565));
#16978=DIRECTION('',(0.,-1.,0.));
#16979=DIRECTION('center_axis',(0.,1.,0.));
#16980=DIRECTION('ref_axis',(0.223538897454053,0.,-0.974695009387565));
#16981=DIRECTION('',(0.,-1.,0.));
#16982=DIRECTION('center_axis',(0.,1.,0.));
#16983=DIRECTION('ref_axis',(0.223538897454053,0.,-0.974695009387565));
#16984=DIRECTION('',(0.,-1.,0.));
#16985=DIRECTION('center_axis',(0.,1.,0.));
#16986=DIRECTION('ref_axis',(0.223538897454053,0.,-0.974695009387565));
#16987=DIRECTION('',(0.,-1.,0.));
#16988=DIRECTION('center_axis',(0.,1.,0.));
#16989=DIRECTION('ref_axis',(0.223538897454053,0.,-0.974695009387565));
#16990=DIRECTION('',(0.,-1.,0.));
#16991=DIRECTION('center_axis',(0.,1.,0.));
#16992=DIRECTION('ref_axis',(0.223538897454053,0.,-0.974695009387565));
#16993=DIRECTION('',(0.,-1.,0.));
#16994=DIRECTION('center_axis',(0.,1.,0.));
#16995=DIRECTION('ref_axis',(0.223538897454053,0.,-0.974695009387565));
#16996=DIRECTION('',(0.,-1.,0.));
#16997=DIRECTION('center_axis',(0.,1.,0.));
#16998=DIRECTION('ref_axis',(0.223538897454053,0.,-0.974695009387565));
#16999=DIRECTION('',(0.,-1.,0.));
#17000=DIRECTION('center_axis',(0.,1.,0.));
#17001=DIRECTION('ref_axis',(0.223538897454053,0.,-0.974695009387565));
#17002=DIRECTION('',(0.,-1.,0.));
#17003=DIRECTION('center_axis',(0.,1.,0.));
#17004=DIRECTION('ref_axis',(0.223538897454053,0.,-0.974695009387565));
#17005=DIRECTION('',(0.,-1.,0.));
#17006=DIRECTION('center_axis',(4.06756404254584E-31,1.,1.13752359080447E-16));
#17007=DIRECTION('ref_axis',(-0.974695009387565,2.54280769316413E-17,-0.223538897454056));
#17008=DIRECTION('',(-4.06756404254584E-31,-1.,-1.13752359080446E-16));
#17009=DIRECTION('',(-4.06756404254584E-31,-1.,-1.13752359080446E-16));
#17010=DIRECTION('center_axis',(4.06756404254584E-31,1.,1.13752359080447E-16));
#17011=DIRECTION('ref_axis',(-0.974695009387565,2.54280769316413E-17,-0.223538897454056));
#17012=DIRECTION('',(1.10873856701774E-16,1.,1.39180436012088E-16));
#17013=DIRECTION('center_axis',(4.06756404254584E-31,1.,1.13752359080447E-16));
#17014=DIRECTION('ref_axis',(-0.974695009387565,2.54280769316413E-17,-0.223538897454056));
#17015=DIRECTION('',(-4.06756404254584E-31,-1.,-1.13752359080446E-16));
#17016=DIRECTION('center_axis',(4.06756404254584E-31,1.,1.13752359080447E-16));
#17017=DIRECTION('ref_axis',(-0.974695009387565,2.54280769316413E-17,-0.223538897454056));
#17018=DIRECTION('',(-4.06756404254584E-31,-1.,-1.13752359080446E-16));
#17019=DIRECTION('center_axis',(4.06756404254584E-31,1.,1.13752359080447E-16));
#17020=DIRECTION('ref_axis',(-0.974695009387565,2.54280769316413E-17,-0.223538897454056));
#17021=DIRECTION('',(-4.06756404254584E-31,-1.,-1.13752359080446E-16));
#17022=DIRECTION('center_axis',(4.06756404254584E-31,1.,1.13752359080447E-16));
#17023=DIRECTION('ref_axis',(-0.974695009387565,2.54280769316413E-17,-0.223538897454056));
#17024=DIRECTION('',(-4.06756404254584E-31,-1.,-1.13752359080446E-16));
#17025=DIRECTION('center_axis',(4.06756404254584E-31,1.,1.13752359080447E-16));
#17026=DIRECTION('ref_axis',(-0.974695009387565,2.54280769316413E-17,-0.223538897454056));
#17027=DIRECTION('',(-4.06756404254584E-31,-1.,-1.13752359080446E-16));
#17028=DIRECTION('center_axis',(4.06756404254584E-31,1.,1.13752359080447E-16));
#17029=DIRECTION('ref_axis',(-0.974695009387565,2.54280769316413E-17,-0.223538897454056));
#17030=DIRECTION('',(-4.06756404254584E-31,-1.,-1.13752359080446E-16));
#17031=DIRECTION('center_axis',(4.06756404254584E-31,1.,1.13752359080447E-16));
#17032=DIRECTION('ref_axis',(-0.974695009387565,2.54280769316413E-17,-0.223538897454056));
#17033=DIRECTION('',(-4.06756404254584E-31,-1.,-1.13752359080446E-16));
#17034=DIRECTION('center_axis',(4.06756404254584E-31,1.,1.13752359080447E-16));
#17035=DIRECTION('ref_axis',(-0.974695009387565,2.54280769316413E-17,-0.223538897454056));
#17036=DIRECTION('',(-4.06756404254584E-31,-1.,-1.13752359080446E-16));
#17037=DIRECTION('center_axis',(4.06756404254584E-31,1.,1.13752359080447E-16));
#17038=DIRECTION('ref_axis',(-0.974695009387565,2.54280769316413E-17,-0.223538897454056));
#17039=DIRECTION('',(-4.06756404254584E-31,-1.,-1.13752359080446E-16));
#17040=DIRECTION('center_axis',(4.06756404254584E-31,1.,1.13752359080447E-16));
#17041=DIRECTION('ref_axis',(-0.974695009387565,2.54280769316413E-17,-0.223538897454056));
#17042=DIRECTION('',(-4.06756404254584E-31,-1.,-1.13752359080446E-16));
#17043=DIRECTION('center_axis',(4.06756404254584E-31,1.,1.13752359080447E-16));
#17044=DIRECTION('ref_axis',(-0.974695009387565,2.54280769316413E-17,-0.223538897454056));
#17045=DIRECTION('',(-4.06756404254584E-31,-1.,-1.13752359080446E-16));
#17046=DIRECTION('center_axis',(4.06756404254584E-31,1.,1.13752359080447E-16));
#17047=DIRECTION('ref_axis',(-0.974695009387565,2.54280769316413E-17,-0.223538897454056));
#17048=DIRECTION('center_axis',(-1.10873856701774E-16,-1.,-1.39180436012088E-16));
#17049=DIRECTION('ref_axis',(-0.974695009387565,1.39180436012088E-16,-0.223538897454056));
#17050=DIRECTION('center_axis',(4.06756404254584E-31,1.,1.13752359080447E-16));
#17051=DIRECTION('ref_axis',(-0.974695009387565,2.54280769316414E-17,-0.223538897454057));
#17052=DIRECTION('center_axis',(4.06756404254584E-31,1.,1.13752359080447E-16));
#17053=DIRECTION('ref_axis',(-0.974695009387565,2.54280769316414E-17,-0.223538897454057));
#17054=DIRECTION('',(-4.06756404254584E-31,-1.,-1.13752359080447E-16));
#17055=DIRECTION('center_axis',(4.06756404254584E-31,1.,1.13752359080447E-16));
#17056=DIRECTION('ref_axis',(-0.974695009387565,2.54280769316413E-17,-0.223538897454056));
#17057=DIRECTION('center_axis',(4.06756404254584E-31,1.,1.13752359080447E-16));
#17058=DIRECTION('ref_axis',(-0.974695009387565,2.54280769316413E-17,-0.223538897454056));
#17059=DIRECTION('center_axis',(4.06756404254584E-31,1.,1.13752359080447E-16));
#17060=DIRECTION('ref_axis',(-0.974695009387565,2.54280769316413E-17,-0.223538897454056));
#17061=DIRECTION('center_axis',(4.06756404254584E-31,1.,1.13752359080447E-16));
#17062=DIRECTION('ref_axis',(-0.974695009387565,2.54280769316413E-17,-0.223538897454056));
#17063=DIRECTION('center_axis',(-0.223538897454057,1.56006678063889E-16,
0.974695009387565));
#17064=DIRECTION('ref_axis',(3.48735608098719E-17,1.,-1.52058930540005E-16));
#17065=DIRECTION('center_axis',(0.223538897454057,-8.18731961845386E-17,
-0.974695009387565));
#17066=DIRECTION('ref_axis',(-1.83018440061315E-17,-1.,7.98013957236788E-17));
#17067=DIRECTION('',(-0.223538897454057,1.56006678063889E-16,0.974695009387564));
#17068=DIRECTION('center_axis',(-0.223538897454057,1.56006678063889E-16,
0.974695009387565));
#17069=DIRECTION('ref_axis',(3.48735608098719E-17,1.,-1.52058930540005E-16));
#17070=DIRECTION('center_axis',(-0.223538897454057,1.56006678063889E-16,
0.974695009387565));
#17071=DIRECTION('ref_axis',(3.48735608098719E-17,1.,-1.52058930540005E-16));
#17072=DIRECTION('center_axis',(-0.223538897454057,1.56006678063889E-16,
0.974695009387565));
#17073=DIRECTION('ref_axis',(3.48735608098719E-17,1.,-1.52058930540005E-16));
#17074=DIRECTION('',(-0.223538897454057,1.56006678063889E-16,0.974695009387564));
#17075=DIRECTION('center_axis',(-0.223538897454057,-1.45003302586173E-17,
0.974695009387565));
#17076=DIRECTION('ref_axis',(-3.24138783873102E-18,1.,1.41333995375458E-17));
#17077=DIRECTION('center_axis',(-1.10873856701774E-16,-1.,-1.39180436012088E-16));
#17078=DIRECTION('ref_axis',(0.974695009387565,-1.39180436012088E-16,0.223538897454055));
#17079=DIRECTION('',(0.689213450726628,0.707106781186552,0.158065870248726));
#17080=DIRECTION('center_axis',(4.06756404254584E-31,1.,1.13752359080447E-16));
#17081=DIRECTION('ref_axis',(-0.974695009387565,2.54280769316412E-17,-0.223538897454055));
#17082=DIRECTION('center_axis',(9.65226914079907E-15,1.,-2.54344969793374E-14));
#17083=DIRECTION('ref_axis',(-0.41021732252356,-1.99199681972541E-14,-0.911987800522354));
#17084=DIRECTION('center_axis',(1.62577613129444E-16,1.,-8.62630726148516E-17));
#17085=DIRECTION('ref_axis',(0.223538897454057,-1.20422606761801E-16,-0.974695009387565));
#17086=DIRECTION('',(0.223538897454057,-1.20422606761801E-16,-0.974695009387564));
#17087=DIRECTION('',(-0.974695009387564,1.39180436012088E-16,-0.223538897454057));
#17088=DIRECTION('',(0.974695009387564,-1.39180436012088E-16,0.223538897454057));
#17089=DIRECTION('center_axis',(1.62577613129444E-16,1.,-8.62630726148516E-17));
#17090=DIRECTION('ref_axis',(0.223538897454057,-1.20422606761801E-16,-0.974695009387565));
#17091=DIRECTION('',(0.223538897454057,-1.20422606761801E-16,-0.974695009387564));
#17092=DIRECTION('',(0.974695009387564,-1.39180436012088E-16,0.223538897454057));
#17093=DIRECTION('center_axis',(-0.223538897454057,-1.45003302586173E-17,
0.974695009387565));
#17094=DIRECTION('ref_axis',(1.32417088546636E-16,1.,4.52456407508629E-17));
#17095=DIRECTION('',(-0.0358554746668518,-0.999323153056184,-0.00822318078734816));
#17096=DIRECTION('',(-0.974695009387564,1.39180436012088E-16,-0.223538897454057));
#17097=DIRECTION('',(-0.34917785007855,0.933628307384311,-0.0800812878594524));
#17098=DIRECTION('center_axis',(0.223538897454057,1.45003302586173E-17,
-0.974695009387565));
#17099=DIRECTION('ref_axis',(-3.24138783873102E-18,1.,1.41333995375458E-17));
#17100=DIRECTION('center_axis',(0.223538897454057,1.10873856701773E-16,
-0.974695009387565));
#17101=DIRECTION('ref_axis',(-0.974695009387565,1.39180436012088E-16,-0.223538897454057));
#17102=DIRECTION('',(-0.34917785007855,0.933628307384311,-0.0800812878594525));
#17103=DIRECTION('',(0.974695009387564,-1.39180436012088E-16,0.223538897454057));
#17104=DIRECTION('',(-0.0358554746668519,-0.999323153056184,-0.00822318078734794));
#17105=DIRECTION('center_axis',(0.223538897454057,-1.56006678063889E-16,
-0.974695009387565));
#17106=DIRECTION('ref_axis',(-3.48735608098719E-17,-1.,1.52058930540005E-16));
#17107=DIRECTION('center_axis',(1.62577613129444E-16,1.,-8.62630726148516E-17));
#17108=DIRECTION('ref_axis',(0.223538897454057,-1.20422606761801E-16,-0.974695009387565));
#17109=DIRECTION('',(-0.974695009387565,1.39180436012088E-16,-0.223538897454057));
#17110=DIRECTION('',(0.223538897454057,-1.20422606761801E-16,-0.974695009387564));
#17111=DIRECTION('center_axis',(-0.223538897454057,1.56006678063889E-16,
0.974695009387565));
#17112=DIRECTION('ref_axis',(1.70532037195239E-16,1.,-1.20946689326688E-16));
#17113=DIRECTION('',(-0.0358554746668519,-0.999323153056184,-0.00822318078734794));
#17114=DIRECTION('',(-0.974695009387564,1.39180436012088E-16,-0.223538897454057));
#17115=DIRECTION('',(-0.34917785007855,0.933628307384311,-0.0800812878594525));
#17116=DIRECTION('center_axis',(0.223538897454057,-1.56006678063889E-16,
-0.974695009387565));
#17117=DIRECTION('ref_axis',(-3.48735608098719E-17,-1.,1.52058930540005E-16));
#17118=DIRECTION('center_axis',(0.223538897454057,-8.18731961845386E-17,
-0.974695009387565));
#17119=DIRECTION('ref_axis',(-1.53960320391499E-16,-1.,4.86891545103617E-17));
#17120=DIRECTION('',(0.34917785007855,-0.933628307384311,0.0800812878594524));
#17121=DIRECTION('',(0.974695009387564,-1.39180436012088E-16,0.223538897454057));
#17122=DIRECTION('',(0.0358554746668518,0.999323153056184,0.00822318078734806));
#17123=DIRECTION('center_axis',(-0.223538897454057,8.18731961845386E-17,
0.974695009387565));
#17124=DIRECTION('ref_axis',(-1.83018440061315E-17,-1.,7.98013957236788E-17));
#17125=DIRECTION('center_axis',(-1.10873856701774E-16,-1.,-1.39180436012088E-16));
#17126=DIRECTION('ref_axis',(0.974695009387565,-1.39180436012088E-16,0.223538897454057));
#17127=DIRECTION('',(-0.223538897454057,-1.10873856701773E-16,0.974695009387564));
#17128=DIRECTION('',(-0.974695009387564,1.39180436012088E-16,-0.223538897454057));
#17129=DIRECTION('',(-0.223538897454057,-1.10873856701773E-16,0.974695009387564));
#17130=DIRECTION('',(0.974695009387564,-1.39180436012088E-16,0.223538897454057));
#17131=DIRECTION('center_axis',(0.974695009387565,-1.39180436012088E-16,
0.223538897454057));
#17132=DIRECTION('ref_axis',(0.223538897454057,1.10873856701773E-16,-0.974695009387565));
#17133=DIRECTION('',(-0.223538897454057,1.56006678063889E-16,0.974695009387564));
#17134=DIRECTION('center_axis',(0.974695009387565,-1.39180436012088E-16,
0.223538897454057));
#17135=DIRECTION('ref_axis',(0.223538897454057,6.16297582203915E-33,-0.974695009387565));
#17136=DIRECTION('center_axis',(0.974695009387565,-1.39180436012088E-16,
0.223538897454057));
#17137=DIRECTION('ref_axis',(0.223538897454057,6.16297582203915E-33,-0.974695009387565));
#17138=DIRECTION('',(-0.223538897454057,1.56006678063889E-16,0.974695009387564));
#17139=DIRECTION('center_axis',(0.974695009387565,-1.39180436012088E-16,
0.223538897454057));
#17140=DIRECTION('ref_axis',(0.223538897454057,1.10873856701773E-16,-0.974695009387565));
#17141=DIRECTION('center_axis',(-0.974695009387565,1.39180436012088E-16,
-0.223538897454057));
#17142=DIRECTION('ref_axis',(0.223538897454057,5.55111512312581E-15,-0.974695009387565));
#17143=DIRECTION('',(-0.223538897454057,1.56006678063889E-16,0.974695009387564));
#17144=DIRECTION('',(-0.223538897454057,1.56006678063889E-16,0.974695009387564));
#17145=DIRECTION('center_axis',(-0.974695009387565,1.39180436012088E-16,
-0.223538897454057));
#17146=DIRECTION('ref_axis',(0.223538897454057,6.16297582203915E-33,-0.974695009387565));
#17147=DIRECTION('center_axis',(0.910002851830447,0.358243190655045,0.208702242464586));
#17148=DIRECTION('ref_axis',(-0.34917785007855,0.933628307384311,-0.0800812878594523));
#17149=DIRECTION('center_axis',(-0.910002851830524,-0.358243190654995,-0.208702242464336));
#17150=DIRECTION('ref_axis',(0.349177850069457,-0.93362830738433,0.0800812878988744));
#17151=DIRECTION('center_axis',(0.910002851830446,0.358243190655048,0.208702242464584));
#17152=DIRECTION('ref_axis',(0.349177850078086,-0.93362830738431,0.0800812878614929));
#17153=DIRECTION('',(-0.223538897454057,1.56006678063889E-16,0.974695009387564));
#17154=DIRECTION('center_axis',(-0.974035290049308,0.0367863529837719,-0.223387595834492));
#17155=DIRECTION('ref_axis',(-0.0358554746668518,-0.999323153056184,-0.00822318078734825));
#17156=DIRECTION('center_axis',(0.974035290049308,-0.0367863529837719,0.223387595834492));
#17157=DIRECTION('ref_axis',(0.0358554746668518,0.999323153056184,0.00822318078734814));
#17158=DIRECTION('',(-0.223538897454057,1.56006678063889E-16,0.974695009387564));
#17159=DIRECTION('center_axis',(-0.974035290049323,0.0367863529838382,-0.223387595834417));
#17160=DIRECTION('ref_axis',(0.0358554746968573,0.999323153056181,0.00822318065681202));
#17161=DIRECTION('center_axis',(-0.223538897454057,1.56006678063889E-16,
0.974695009387565));
#17162=DIRECTION('ref_axis',(0.159899237082201,-0.986451936077797,0.0366716755670673));
#17163=DIRECTION('center_axis',(-0.223538897454057,1.56006678063889E-16,
0.974695009387565));
#17164=DIRECTION('ref_axis',(0.159899237082201,-0.986451936077797,0.0366716755670673));
#17165=DIRECTION('',(-0.223538897454057,1.56006678063889E-16,0.974695009387565));
#17166=DIRECTION('',(-0.223538897454057,1.56006678063889E-16,0.974695009387564));
#17167=DIRECTION('center_axis',(-0.974035290049308,0.0367863529837719,-0.223387595834492));
#17168=DIRECTION('ref_axis',(-0.0358554746668518,-0.999323153056184,-0.00822318078734825));
#17169=DIRECTION('center_axis',(0.974035290049308,-0.0367863529837719,0.223387595834492));
#17170=DIRECTION('ref_axis',(0.0358554746668518,0.999323153056184,0.00822318078734814));
#17171=DIRECTION('center_axis',(-0.974035290049297,0.0367863529838035,-0.223387595834534));
#17172=DIRECTION('ref_axis',(0.0358554743858934,0.999323153056183,0.00822318201255029));
#17173=DIRECTION('center_axis',(0.910002851830447,0.358243190655045,0.208702242464586));
#17174=DIRECTION('ref_axis',(-0.34917785007855,0.933628307384311,-0.0800812878594523));
#17175=DIRECTION('center_axis',(-0.910002851830389,-0.358243190654987,-0.208702242464939));
#17176=DIRECTION('ref_axis',(0.349177850195129,-0.933628307384333,0.080081287350873));
#17177=DIRECTION('center_axis',(0.910002851830444,0.358243190655049,0.20870224246459));
#17178=DIRECTION('ref_axis',(0.349177850076088,-0.933628307384309,0.0800812878702079));
#17179=DIRECTION('center_axis',(4.19082355898663E-31,1.,1.13752359080447E-16));
#17180=DIRECTION('ref_axis',(-0.974695009387565,2.54280769316415E-17,-0.223538897454057));
#17181=DIRECTION('center_axis',(4.19082355898663E-31,1.,1.13752359080447E-16));
#17182=DIRECTION('ref_axis',(-0.974695009387565,2.54280769316415E-17,-0.223538897454057));
#17183=DIRECTION('center_axis',(0.974695009387565,-1.39180436012088E-16,
0.223538897454057));
#17184=DIRECTION('ref_axis',(0.223538897454057,1.10873856701773E-16,-0.974695009387565));
#17185=DIRECTION('',(-0.193590363929179,-0.499999999999996,0.844110639071545));
#17186=DIRECTION('',(0.193590363929179,-0.499999999999996,-0.844110639071545));
#17187=DIRECTION('center_axis',(0.,1.,0.));
#17188=DIRECTION('ref_axis',(0.223538897454053,0.,-0.974695009387565));
#17189=DIRECTION('center_axis',(-0.974695009387565,1.39180436012088E-16,
-0.223538897454057));
#17190=DIRECTION('ref_axis',(-0.223538897454057,-6.16297582203915E-33,0.974695009387565));
#17191=DIRECTION('center_axis',(-0.974695009387565,1.39180436012088E-16,
-0.223538897454057));
#17192=DIRECTION('ref_axis',(-0.223538897454057,-6.16297582203915E-33,0.974695009387565));
#17193=DIRECTION('center_axis',(0.974695009387565,-1.39180436012088E-16,
0.223538897454057));
#17194=DIRECTION('ref_axis',(0.223538897454057,-1.10317267214501E-30,-0.974695009387565));
#17195=DIRECTION('center_axis',(0.974695009387565,-1.39180436012088E-16,
0.223538897454057));
#17196=DIRECTION('ref_axis',(0.223538897454057,-1.10317267214501E-30,-0.974695009387565));
#17197=DIRECTION('center_axis',(0.,-1.,0.));
#17198=DIRECTION('ref_axis',(-0.99646141012762,0.,-0.0840515206672309));
#17199=DIRECTION('',(0.,1.,0.));
#17200=DIRECTION('center_axis',(-4.15314294130208E-14,-1.,-7.5151094970912E-14));
#17201=DIRECTION('ref_axis',(0.303675785059601,-8.33478827153308E-14,0.952775428717825));
#17202=DIRECTION('center_axis',(0.,-1.,0.));
#17203=DIRECTION('ref_axis',(-0.99646141012762,0.,-0.0840515206672309));
#17204=DIRECTION('',(0.,1.,0.));
#17205=DIRECTION('center_axis',(0.,-1.,0.));
#17206=DIRECTION('ref_axis',(-0.99646141012762,0.,-0.0840515206672309));
#17207=DIRECTION('',(0.,1.,0.));
#17208=DIRECTION('center_axis',(0.,-1.,0.));
#17209=DIRECTION('ref_axis',(-0.99646141012762,0.,-0.0840515206672309));
#17210=DIRECTION('',(0.,1.,0.));
#17211=DIRECTION('center_axis',(0.,-1.,0.));
#17212=DIRECTION('ref_axis',(-0.99646141012762,0.,-0.0840515206672309));
#17213=DIRECTION('',(0.,1.,0.));
#17214=DIRECTION('center_axis',(0.,-1.,0.));
#17215=DIRECTION('ref_axis',(-0.99646141012762,0.,-0.0840515206672309));
#17216=DIRECTION('',(0.,1.,0.));
#17217=DIRECTION('center_axis',(0.,-1.,0.));
#17218=DIRECTION('ref_axis',(-0.99646141012762,0.,-0.0840515206672309));
#17219=DIRECTION('',(0.,1.,0.));
#17220=DIRECTION('center_axis',(0.,-1.,0.));
#17221=DIRECTION('ref_axis',(-0.99646141012762,0.,-0.0840515206672309));
#17222=DIRECTION('',(0.,1.,0.));
#17223=DIRECTION('',(4.52978722919878E-31,1.,1.13752359080446E-16));
#17224=DIRECTION('center_axis',(-4.52978722919878E-31,-1.,-1.13752359080446E-16));
#17225=DIRECTION('ref_axis',(-0.99646141012762,9.56105876019769E-18,-0.0840515206672388));
#17226=DIRECTION('',(-4.52978722919878E-31,-1.,-1.13752359080446E-16));
#17227=DIRECTION('',(-4.52978722919878E-31,-1.,-1.13752359080446E-16));
#17228=DIRECTION('',(-4.52978722919878E-31,-1.,-1.13752359080446E-16));
#17229=DIRECTION('center_axis',(4.52978722919878E-31,1.,1.13752359080446E-16));
#17230=DIRECTION('ref_axis',(0.99646141012762,-9.56105876019769E-18,0.0840515206672388));
#17231=DIRECTION('center_axis',(-4.52978722919878E-31,-1.,-1.13752359080446E-16));
#17232=DIRECTION('ref_axis',(-0.99646141012762,9.56105876019769E-18,-0.0840515206672388));
#17233=DIRECTION('',(-4.52978722919878E-31,-1.,-1.13752359080446E-16));
#17234=DIRECTION('center_axis',(-4.52978722919878E-31,-1.,-1.13752359080446E-16));
#17235=DIRECTION('ref_axis',(-0.99646141012762,9.56105876019769E-18,-0.0840515206672388));
#17236=DIRECTION('',(-4.52978722919878E-31,-1.,-1.13752359080446E-16));
#17237=DIRECTION('center_axis',(-4.52978722919878E-31,-1.,-1.13752359080446E-16));
#17238=DIRECTION('ref_axis',(-0.99646141012762,9.56105876019769E-18,-0.0840515206672388));
#17239=DIRECTION('',(-4.52978722919878E-31,-1.,-1.13752359080446E-16));
#17240=DIRECTION('center_axis',(-4.52978722919878E-31,-1.,-1.13752359080446E-16));
#17241=DIRECTION('ref_axis',(-0.99646141012762,9.56105876019769E-18,-0.0840515206672388));
#17242=DIRECTION('',(-4.52978722919878E-31,-1.,-1.13752359080446E-16));
#17243=DIRECTION('center_axis',(-4.52978722919878E-31,-1.,-1.13752359080446E-16));
#17244=DIRECTION('ref_axis',(-0.99646141012762,9.56105876019769E-18,-0.0840515206672388));
#17245=DIRECTION('',(-4.52978722919878E-31,-1.,-1.13752359080446E-16));
#17246=DIRECTION('center_axis',(-4.52978722919878E-31,-1.,-1.13752359080446E-16));
#17247=DIRECTION('ref_axis',(-0.99646141012762,9.56105876019769E-18,-0.0840515206672388));
#17248=DIRECTION('',(-4.52978722919878E-31,-1.,-1.13752359080446E-16));
#17249=DIRECTION('center_axis',(-4.52978722919878E-31,-1.,-1.13752359080446E-16));
#17250=DIRECTION('ref_axis',(-0.99646141012762,9.56105876019769E-18,-0.0840515206672388));
#17251=DIRECTION('',(-4.52978722919878E-31,-1.,-1.13752359080446E-16));
#17252=DIRECTION('center_axis',(4.52978722919878E-31,1.,1.13752359080446E-16));
#17253=DIRECTION('ref_axis',(0.99646141012762,-9.56105876019769E-18,0.0840515206672388));
#17254=DIRECTION('center_axis',(-4.52978722919878E-31,-1.,-1.13752359080446E-16));
#17255=DIRECTION('ref_axis',(-0.99646141012762,9.56105876019769E-18,-0.0840515206672388));
#17256=DIRECTION('center_axis',(-4.52978722919878E-31,-1.,-1.13752359080446E-16));
#17257=DIRECTION('ref_axis',(-0.99646141012762,9.56105876019769E-18,-0.0840515206672388));
#17258=DIRECTION('center_axis',(4.52978722919878E-31,1.,1.13752359080446E-16));
#17259=DIRECTION('ref_axis',(0.99646141012762,-9.56105876019769E-18,0.0840515206672388));
#17260=DIRECTION('',(4.52978722919878E-31,1.,1.13752359080446E-16));
#17261=DIRECTION('center_axis',(4.52978722919878E-31,1.,1.13752359080446E-16));
#17262=DIRECTION('ref_axis',(0.99646141012762,-9.56105876019769E-18,0.0840515206672388));
#17263=DIRECTION('center_axis',(4.51437978964368E-31,1.,1.13752359080446E-16));
#17264=DIRECTION('ref_axis',(0.99646141012762,-9.56105876019768E-18,0.0840515206672388));
#17265=DIRECTION('',(0.99646141012762,-9.56105876019769E-18,0.0840515206672387));
#17266=DIRECTION('',(0.904986655395003,4.83947982939151E-17,-0.425439952939268));
#17267=DIRECTION('',(0.571021457188351,9.33833082273063E-17,-0.820935134727764));
#17268=DIRECTION('',(0.0840515206672388,1.13349836134644E-16,-0.99646141012762));
#17269=DIRECTION('',(-0.425439952939269,1.02944366987504E-16,-0.904986655395002));
#17270=DIRECTION('',(-0.820935134727764,6.4955037840729E-17,-0.571021457188351));
#17271=DIRECTION('',(-0.99646141012762,9.56105876019769E-18,-0.0840515206672387));
#17272=DIRECTION('',(-0.904986655395003,-4.83947982939151E-17,0.425439952939268));
#17273=DIRECTION('',(-0.571021457188351,-9.33833082273063E-17,0.820935134727764));
#17274=DIRECTION('',(-0.0840515206672388,-1.13349836134644E-16,0.99646141012762));
#17275=DIRECTION('',(0.425439952939269,-1.02944366987504E-16,0.904986655395002));
#17276=DIRECTION('',(0.820935134727764,-6.4955037840729E-17,0.571021457188351));
#17277=DIRECTION('center_axis',(4.51437978964368E-31,1.,1.13752359080446E-16));
#17278=DIRECTION('ref_axis',(0.99646141012762,-9.56105876019768E-18,0.0840515206672388));
#17279=DIRECTION('',(0.99646141012762,-9.56105876019769E-18,0.0840515206672387));
#17280=DIRECTION('',(0.425439952939269,-1.02944366987504E-16,0.904986655395002));
#17281=DIRECTION('',(-0.571021457188351,-9.33833082273063E-17,0.820935134727764));
#17282=DIRECTION('',(-0.99646141012762,9.56105876019769E-18,-0.0840515206672387));
#17283=DIRECTION('',(-0.425439952939269,1.02944366987504E-16,-0.904986655395002));
#17284=DIRECTION('',(0.571021457188351,9.33833082273063E-17,-0.820935134727764));
#17285=DIRECTION('center_axis',(4.51437978964368E-31,1.,1.13752359080446E-16));
#17286=DIRECTION('ref_axis',(0.99646141012762,-9.56105876019768E-18,0.0840515206672388));
#17287=DIRECTION('center_axis',(0.0840515206672388,1.13349836134644E-16,
-0.99646141012762));
#17288=DIRECTION('ref_axis',(4.54519466875388E-31,1.,1.13752359080446E-16));
#17289=DIRECTION('',(0.70460462029195,-0.707106781186548,0.0594334002328457));
#17290=DIRECTION('',(0.704604620291949,0.707106781186547,0.0594334002328458));
#17291=DIRECTION('',(-4.52978722919878E-31,-1.,-1.13752359080446E-16));
#17292=DIRECTION('',(-4.52978722919878E-31,-1.,-1.13752359080446E-16));
#17293=DIRECTION('center_axis',(-0.820935134727764,6.4955037840729E-17,
-0.571021457188352));
#17294=DIRECTION('ref_axis',(-0.571021457188352,-9.33833082273063E-17,0.820935134727764));
#17295=DIRECTION('',(0.403773144580907,0.707106781186548,-0.580488800680294));
#17296=DIRECTION('',(-4.52978722919878E-31,-1.,-1.13752359080446E-16));
#17297=DIRECTION('',(0.403773144580907,-0.707106781186547,-0.580488800680294));
#17298=DIRECTION('center_axis',(-0.904986655395002,-4.83947982939152E-17,
0.425439952939269));
#17299=DIRECTION('ref_axis',(0.425439952939269,-1.02944366987504E-16,0.904986655395002));
#17300=DIRECTION('',(-0.300831475711043,-0.707106781186547,-0.63992220091314));
#17301=DIRECTION('',(-0.300831475711043,0.707106781186548,-0.639922200913139));
#17302=DIRECTION('',(-4.52978722919878E-31,-1.,-1.13752359080446E-16));
#17303=DIRECTION('center_axis',(-0.0840515206672388,-1.13349836134644E-16,
0.99646141012762));
#17304=DIRECTION('ref_axis',(-4.54519466875388E-31,-1.,-1.13752359080446E-16));
#17305=DIRECTION('',(-0.70460462029195,0.707106781186548,-0.0594334002328457));
#17306=DIRECTION('',(-4.52978722919878E-31,-1.,-1.13752359080446E-16));
#17307=DIRECTION('',(-0.704604620291949,-0.707106781186547,-0.0594334002328458));
#17308=DIRECTION('center_axis',(0.820935134727764,-6.4955037840729E-17,
0.571021457188352));
#17309=DIRECTION('ref_axis',(0.571021457188352,9.33833082273063E-17,-0.820935134727764));
#17310=DIRECTION('',(-0.403773144580907,-0.707106781186548,0.580488800680294));
#17311=DIRECTION('',(-0.403773144580907,0.707106781186547,0.580488800680294));
#17312=DIRECTION('',(-4.52978722919878E-31,-1.,-1.13752359080446E-16));
#17313=DIRECTION('center_axis',(0.904986655395002,4.83947982939152E-17,
-0.425439952939269));
#17314=DIRECTION('ref_axis',(-0.425439952939269,1.02944366987504E-16,-0.904986655395002));
#17315=DIRECTION('',(0.300831475711043,-0.707106781186548,0.639922200913139));
#17316=DIRECTION('',(0.300831475711043,0.707106781186548,0.639922200913139));
#17317=DIRECTION('center_axis',(0.0840515206672388,1.13349836134644E-16,
-0.99646141012762));
#17318=DIRECTION('ref_axis',(4.54519466875388E-31,1.,1.13752359080446E-16));
#17319=DIRECTION('',(-0.862960895061384,0.499999999999998,-0.0727907521245416));
#17320=DIRECTION('',(0.862960895061384,0.499999999999998,0.0727907521245417));
#17321=DIRECTION('center_axis',(0.,-1.,0.));
#17322=DIRECTION('ref_axis',(-0.99646141012762,0.,-0.0840515206672309));
#17323=DIRECTION('center_axis',(-0.380525062046606,0.447213595499958,-0.809444672077361));
#17324=DIRECTION('ref_axis',(-0.0420257603336194,0.866025403784439,0.49823070506381));
#17325=DIRECTION('center_axis',(0.891262180000262,0.447213595499958,0.0751779655296698));
#17326=DIRECTION('ref_axis',(0.445631090000131,-0.894427190999916,0.0375889827648348));
#17327=DIRECTION('center_axis',(0.510737117953656,0.447213595499958,-0.734266706547691));
#17328=DIRECTION('ref_axis',(-0.0420257603336193,0.866025403784439,0.49823070506381));
#17329=DIRECTION('center_axis',(-0.891262180000262,0.447213595499958,-0.0751779655296697));
#17330=DIRECTION('ref_axis',(0.445631090000131,0.894427190999916,0.037588982764835));
#17331=DIRECTION('center_axis',(-0.510737117953656,0.447213595499958,0.734266706547692));
#17332=DIRECTION('ref_axis',(-0.0420257603336193,-0.866025403784439,0.49823070506381));
#17333=DIRECTION('center_axis',(0.380525062046606,0.447213595499958,0.809444672077361));
#17334=DIRECTION('ref_axis',(-0.0420257603336194,-0.866025403784439,0.49823070506381));
#23312=CARTESIAN_POINT('',(0.,0.,0.));
#23313=CARTESIAN_POINT('Origin',(210.55281376718,40.2397376070394,351.055932202117));
#23314=CARTESIAN_POINT('',(229.603651352553,35.4089854465581,354.809519933842));
#23315=CARTESIAN_POINT('',(191.770222858752,45.0704897675207,346.132710459127));
#23316=CARTESIAN_POINT('Origin',(210.686937105653,40.2397376070394,350.471115196485));
#23317=CARTESIAN_POINT('Origin',(210.686937105653,40.2397376070394,350.471115196485));
#23318=CARTESIAN_POINT('',(191.068598092873,45.2154123323351,346.587375322639));
#23319=CARTESIAN_POINT('',(191.068598092873,45.2154123323351,346.587375322639));
#23320=CARTESIAN_POINT('Origin',(210.55281376718,40.2397376070394,351.055932202117));
#23321=CARTESIAN_POINT('Origin',(214.889468377789,40.2397376070394,332.146849019998));
#23322=CARTESIAN_POINT('',(233.806182624689,35.4089854465581,336.485253757356));
#23323=CARTESIAN_POINT('Origin',(214.889468377789,40.2397376070394,332.146849019998));
#23324=CARTESIAN_POINT('',(234.507807390569,35.2640628817436,336.030588893844));
#23325=CARTESIAN_POINT('',(233.806182624689,35.4089854465581,336.485253757356));
#23326=CARTESIAN_POINT('Origin',(215.023591716261,40.2397376070394,331.562032014366));
#23327=CARTESIAN_POINT('Origin',(214.576513921353,40.2397376070394,333.511422033141));
#23328=CARTESIAN_POINT('',(236.777813100197,34.6843726224859,336.551197462327));
#23329=CARTESIAN_POINT('Origin',(215.023591716261,40.2397376070394,331.562032014366));
#23330=CARTESIAN_POINT('',(238.222406729979,34.2012974064378,338.934427954838));
#23331=CARTESIAN_POINT('Origin',(236.330735305289,34.6843726224859,338.500587481102));
#23332=CARTESIAN_POINT('',(190.930621112728,46.278177807641,328.088416111445));
#23333=CARTESIAN_POINT('Origin',(214.576513921353,40.2397376070394,333.511422033141));
#23334=CARTESIAN_POINT('Origin',(214.576513921353,40.2397376070394,333.511422033141));
#23335=CARTESIAN_POINT('Origin',(214.464744472626,40.2397376070394,333.998769537835));
#23336=CARTESIAN_POINT('',(231.042709499928,35.8920606626062,339.852723820232));
#23337=CARTESIAN_POINT('Origin',(214.017666677718,40.2397376070394,335.94815955661));
#23338=CARTESIAN_POINT('',(233.381458719527,35.4089854465581,338.337174275192));
#23339=CARTESIAN_POINT('Origin',(231.489787294837,35.8920606626062,337.903333801457));
#23340=CARTESIAN_POINT('Origin',(214.464744472626,40.2397376070394,333.998769537835));
#23341=CARTESIAN_POINT('Origin',(210.999891562088,40.2397376070394,349.106542183342));
#23342=CARTESIAN_POINT('',(187.353998753463,46.278177807641,343.683536261645));
#23343=CARTESIAN_POINT('',(234.645784370714,34.2012974064378,354.529548105039));
#23344=CARTESIAN_POINT('Origin',(210.999891562088,40.2397376070394,349.106542183342));
#23345=CARTESIAN_POINT('Origin',(210.999891562088,40.2397376070394,349.106542183342));
#23346=CARTESIAN_POINT('',(232.307035151116,34.6843726224859,356.045097650078));
#23347=CARTESIAN_POINT('Origin',(232.754112946024,34.6843726224859,354.095707631303));
#23348=CARTESIAN_POINT('Origin',(210.55281376718,40.2397376070394,351.055932202117));
#23349=CARTESIAN_POINT('Origin',(211.111661010815,40.2397376070394,348.619194678648));
#23350=CARTESIAN_POINT('',(194.533695983513,44.5874145514725,342.765240396252));
#23351=CARTESIAN_POINT('Origin',(211.558738805724,40.2397376070394,346.669804659873));
#23352=CARTESIAN_POINT('',(192.194946763915,45.0704897675207,344.280789941291));
#23353=CARTESIAN_POINT('Origin',(194.086618188605,44.5874145514726,344.714630415027));
#23354=CARTESIAN_POINT('',(230.028375257716,35.4089854465581,352.957599416006));
#23355=CARTESIAN_POINT('Origin',(211.111661010815,40.2397376070394,348.619194678648));
#23356=CARTESIAN_POINT('Origin',(211.111661010815,40.2397376070394,348.619194678648));
#23357=CARTESIAN_POINT('Origin',(210.552590228283,40.2397376070394,351.056906897127));
#23358=CARTESIAN_POINT('',(215.281992328905,39.0320495669191,352.140533386457));
#23359=CARTESIAN_POINT('Origin',(210.55281376718,40.2397376070394,351.055932202117));
#23360=CARTESIAN_POINT('',(219.752770277987,39.0320495669191,332.646633198705));
#23361=CARTESIAN_POINT('',(215.281768790008,39.0320495669191,352.141508081466));
#23362=CARTESIAN_POINT('Origin',(215.023591716261,40.2397376070394,331.562032014366));
#23363=CARTESIAN_POINT('Origin',(215.023591716261,40.2397376070394,331.562032014366));
#23364=CARTESIAN_POINT('',(199.830130992543,43.8628017274004,332.694356003592));
#23365=CARTESIAN_POINT('Origin',(214.017666677718,40.2397376070394,335.94815955661));
#23366=CARTESIAN_POINT('',(208.402741729846,41.9305008632078,330.043590356291));
#23367=CARTESIAN_POINT('',(208.402741729846,41.9305008632078,330.043590356291));
#23368=CARTESIAN_POINT('Origin',(215.023591716261,40.2397376070394,331.562032014366));
#23369=CARTESIAN_POINT('Origin',(212.788202741721,40.2397376070394,341.308982108242));
#23370=CARTESIAN_POINT('',(231.704916988621,35.4089854465581,345.647386845599));
#23371=CARTESIAN_POINT('Origin',(211.558738805724,40.2397376070394,346.669804659873));
#23372=CARTESIAN_POINT('',(225.746274490899,36.6166734866784,349.923608212891));
#23373=CARTESIAN_POINT('Origin',(211.558738805724,40.2397376070394,346.669804659873));
#23374=CARTESIAN_POINT('',(217.173663753595,38.5489743508709,352.574373860192));
#23375=CARTESIAN_POINT('',(225.746274490899,36.6166734866784,349.923608212891));
#23376=CARTESIAN_POINT('Origin',(210.55281376718,40.2397376070394,351.055932202117));
#23377=CARTESIAN_POINT('Origin',(212.788202741721,40.2397376070394,341.308982108242));
#23378=CARTESIAN_POINT('',(231.704916988621,35.4089854465581,345.647386845599));
#23379=CARTESIAN_POINT('Origin',(215.023591716261,40.2397376070394,331.562032014366));
#23380=CARTESIAN_POINT('',(191.377698907636,46.278177807641,326.139026092669));
#23381=CARTESIAN_POINT('Origin',(215.023591716261,40.2397376070394,331.562032014366));
#23382=CARTESIAN_POINT('Origin',(210.55281376718,40.2397376070394,351.055932202117));
#23383=CARTESIAN_POINT('Origin',(216.267248828133,59.6475667892021,347.749665671701));
#23384=CARTESIAN_POINT('Origin',(218.726176700127,59.6475667892021,337.028020568438));
#23385=CARTESIAN_POINT('Origin',(210.55281376718,40.2397376070394,351.055932202117));
#23386=CARTESIAN_POINT('Origin',(215.023591716261,40.2397376070394,331.562032014366));
#23387=CARTESIAN_POINT('Origin',(216.096578424042,40.2397376070391,326.883495969306));
#23388=CARTESIAN_POINT('',(211.320572878043,40.2397376070391,325.78815537178));
#23389=CARTESIAN_POINT('Origin',(216.096578424042,40.2397376070391,326.883495969306));
#23390=CARTESIAN_POINT('',(211.560219659412,40.2397376070391,325.637924149394));
#23391=CARTESIAN_POINT('',(211.320572878043,40.2397376070391,325.78815537178));
#23392=CARTESIAN_POINT('Origin',(216.141286203533,40.2397376070391,326.688556967428));
#23393=CARTESIAN_POINT('Origin',(209.435119279911,40.2397376070391,355.929407249055));
#23394=CARTESIAN_POINT('',(204.703821513403,40.2397376070391,354.639127649653));
#23395=CARTESIAN_POINT('',(214.255832605401,40.2397376070391,356.829808844702));
#23396=CARTESIAN_POINT('Origin',(209.479827059402,40.2397376070391,355.734468247177));
#23397=CARTESIAN_POINT('Origin',(209.479827059402,40.2397376070391,355.734468247177));
#23398=CARTESIAN_POINT('',(214.016185824033,40.2397376070391,356.980040067089));
#23399=CARTESIAN_POINT('',(214.016185824033,40.2397376070391,356.980040067089));
#23400=CARTESIAN_POINT('Origin',(209.435119279911,40.2397376070391,355.929407249055));
#23401=CARTESIAN_POINT('Origin',(219.239377260408,40.2397376070391,313.179973333186));
#23402=CARTESIAN_POINT('',(214.463371714409,40.2397376070391,312.084632735661));
#23403=CARTESIAN_POINT('Origin',(225.888236297409,31.2397376070391,328.923945941969));
#23404=CARTESIAN_POINT('Origin',(209.435119279911,40.2397376070391,355.929407249055));
#23405=CARTESIAN_POINT('Origin',(203.041252647847,101.652237608405,339.0735931337));
#23406=CARTESIAN_POINT('',(202.044552137503,88.2772376084047,343.419499033524));
#23407=CARTESIAN_POINT('',(202.044552137503,88.0272376084047,343.419499033524));
#23408=CARTESIAN_POINT('',(202.044552137504,101.652237608405,343.419499033523));
#23409=CARTESIAN_POINT('',(204.03795315819,87.7772376084047,334.727687233877));
#23410=CARTESIAN_POINT('Ctrl Pts',(202.044552137503,88.2772376084047,343.419499033524));
#23411=CARTESIAN_POINT('Ctrl Pts',(200.244418972999,88.2147376084047,343.006652164516));
#23412=CARTESIAN_POINT('Ctrl Pts',(199.263459426007,88.1522376084047,341.441838976189));
#23413=CARTESIAN_POINT('Ctrl Pts',(198.282499879015,88.0897376084047,339.877025787862));
#23414=CARTESIAN_POINT('Ctrl Pts',(198.695346748023,88.0272376084047,338.076892623358));
#23415=CARTESIAN_POINT('Ctrl Pts',(199.108193617031,87.9647376084047,336.276759458854));
#23416=CARTESIAN_POINT('Ctrl Pts',(200.673006805358,87.9022376084047,335.295799911861));
#23417=CARTESIAN_POINT('Ctrl Pts',(202.237819993686,87.8397376084047,334.314840364869));
#23418=CARTESIAN_POINT('Ctrl Pts',(204.03795315819,87.7772376084047,334.727687233877));
#23419=CARTESIAN_POINT('',(204.03795315819,87.5272376084047,334.727687233877));
#23420=CARTESIAN_POINT('',(204.03795315819,87.6522376084047,334.727687233877));
#23421=CARTESIAN_POINT('Ctrl Pts',(202.044552137503,88.0272376084047,343.419499033524));
#23422=CARTESIAN_POINT('Ctrl Pts',(200.244418972999,87.9647376084047,343.006652164516));
#23423=CARTESIAN_POINT('Ctrl Pts',(199.263459426007,87.9022376084047,341.441838976189));
#23424=CARTESIAN_POINT('Ctrl Pts',(198.282499879015,87.8397376084047,339.877025787862));
#23425=CARTESIAN_POINT('Ctrl Pts',(198.695346748023,87.7772376084047,338.076892623358));
#23426=CARTESIAN_POINT('Ctrl Pts',(199.108193617031,87.7147376084047,336.276759458854));
#23427=CARTESIAN_POINT('Ctrl Pts',(200.673006805358,87.6522376084047,335.295799911861));
#23428=CARTESIAN_POINT('Ctrl Pts',(202.237819993686,87.5897376084047,334.314840364869));
#23429=CARTESIAN_POINT('Ctrl Pts',(204.03795315819,87.5272376084047,334.727687233877));
#23430=CARTESIAN_POINT('Origin',(203.041252647847,101.652237608405,339.0735931337));
#23431=CARTESIAN_POINT('',(202.044552137503,89.2772376084047,343.419499033524));
#23432=CARTESIAN_POINT('',(202.044552137503,89.0272376084047,343.419499033524));
#23433=CARTESIAN_POINT('',(202.044552137504,101.652237608405,343.419499033523));
#23434=CARTESIAN_POINT('Ctrl Pts',(202.044552137503,89.2772376084047,343.419499033524));
#23435=CARTESIAN_POINT('Ctrl Pts',(200.244418972999,89.2147376084047,343.006652164516));
#23436=CARTESIAN_POINT('Ctrl Pts',(199.263459426007,89.1522376084047,341.441838976189));
#23437=CARTESIAN_POINT('Ctrl Pts',(198.282499879015,89.0897376084047,339.877025787862));
#23438=CARTESIAN_POINT('Ctrl Pts',(198.695346748023,89.0272376084047,338.076892623358));
#23439=CARTESIAN_POINT('Ctrl Pts',(199.108193617031,88.9647376084047,336.276759458854));
#23440=CARTESIAN_POINT('Ctrl Pts',(200.673006805358,88.9022376084047,335.295799911861));
#23441=CARTESIAN_POINT('Ctrl Pts',(202.237819993686,88.8397376084047,334.314840364869));
#23442=CARTESIAN_POINT('Ctrl Pts',(204.03795315819,88.7772376084047,334.727687233877));
#23443=CARTESIAN_POINT('Ctrl Pts',(205.838086322694,88.7147376084047,335.140534102886));
#23444=CARTESIAN_POINT('Ctrl Pts',(206.819045869686,88.6522376084047,336.705347291213));
#23445=CARTESIAN_POINT('Ctrl Pts',(207.800005416678,88.5897376084047,338.27016047954));
#23446=CARTESIAN_POINT('Ctrl Pts',(207.38715854767,88.5272376084047,340.070293644044));
#23447=CARTESIAN_POINT('Ctrl Pts',(206.974311678662,88.4647376084047,341.870426808548));
#23448=CARTESIAN_POINT('Ctrl Pts',(205.409498490334,88.4022376084047,342.851386355541));
#23449=CARTESIAN_POINT('Ctrl Pts',(203.844685302007,88.3397376084047,343.832345902533));
#23450=CARTESIAN_POINT('Ctrl Pts',(202.044552137503,88.2772376084047,343.419499033524));
#23451=CARTESIAN_POINT('Ctrl Pts',(202.044552137503,89.0272376084047,343.419499033524));
#23452=CARTESIAN_POINT('Ctrl Pts',(200.244418972999,88.9647376084047,343.006652164516));
#23453=CARTESIAN_POINT('Ctrl Pts',(199.263459426007,88.9022376084047,341.441838976189));
#23454=CARTESIAN_POINT('Ctrl Pts',(198.282499879015,88.8397376084047,339.877025787862));
#23455=CARTESIAN_POINT('Ctrl Pts',(198.695346748023,88.7772376084047,338.076892623358));
#23456=CARTESIAN_POINT('Ctrl Pts',(199.108193617031,88.7147376084047,336.276759458854));
#23457=CARTESIAN_POINT('Ctrl Pts',(200.673006805358,88.6522376084047,335.295799911861));
#23458=CARTESIAN_POINT('Ctrl Pts',(202.237819993686,88.5897376084047,334.314840364869));
#23459=CARTESIAN_POINT('Ctrl Pts',(204.03795315819,88.5272376084047,334.727687233877));
#23460=CARTESIAN_POINT('Ctrl Pts',(205.838086322694,88.4647376084047,335.140534102886));
#23461=CARTESIAN_POINT('Ctrl Pts',(206.819045869686,88.4022376084047,336.705347291213));
#23462=CARTESIAN_POINT('Ctrl Pts',(207.800005416678,88.3397376084047,338.27016047954));
#23463=CARTESIAN_POINT('Ctrl Pts',(207.38715854767,88.2772376084047,340.070293644044));
#23464=CARTESIAN_POINT('Ctrl Pts',(206.974311678662,88.2147376084047,341.870426808548));
#23465=CARTESIAN_POINT('Ctrl Pts',(205.409498490334,88.1522376084047,342.851386355541));
#23466=CARTESIAN_POINT('Ctrl Pts',(203.844685302007,88.0897376084047,343.832345902533));
#23467=CARTESIAN_POINT('Ctrl Pts',(202.044552137503,88.0272376084047,343.419499033524));
#23468=CARTESIAN_POINT('Origin',(203.041252647847,101.652237608405,339.0735931337));
#23469=CARTESIAN_POINT('',(202.044552137503,90.2772376084047,343.419499033524));
#23470=CARTESIAN_POINT('',(202.044552137503,90.0272376084047,343.419499033524));
#23471=CARTESIAN_POINT('',(202.044552137504,101.652237608405,343.419499033523));
#23472=CARTESIAN_POINT('Ctrl Pts',(202.044552137503,90.2772376084047,343.419499033524));
#23473=CARTESIAN_POINT('Ctrl Pts',(200.244418972999,90.2147376084047,343.006652164516));
#23474=CARTESIAN_POINT('Ctrl Pts',(199.263459426007,90.1522376084047,341.441838976189));
#23475=CARTESIAN_POINT('Ctrl Pts',(198.282499879015,90.0897376084047,339.877025787862));
#23476=CARTESIAN_POINT('Ctrl Pts',(198.695346748023,90.0272376084047,338.076892623358));
#23477=CARTESIAN_POINT('Ctrl Pts',(199.108193617031,89.9647376084047,336.276759458854));
#23478=CARTESIAN_POINT('Ctrl Pts',(200.673006805358,89.9022376084047,335.295799911861));
#23479=CARTESIAN_POINT('Ctrl Pts',(202.237819993686,89.8397376084047,334.314840364869));
#23480=CARTESIAN_POINT('Ctrl Pts',(204.03795315819,89.7772376084047,334.727687233877));
#23481=CARTESIAN_POINT('Ctrl Pts',(205.838086322694,89.7147376084047,335.140534102886));
#23482=CARTESIAN_POINT('Ctrl Pts',(206.819045869686,89.6522376084047,336.705347291213));
#23483=CARTESIAN_POINT('Ctrl Pts',(207.800005416678,89.5897376084047,338.27016047954));
#23484=CARTESIAN_POINT('Ctrl Pts',(207.38715854767,89.5272376084047,340.070293644044));
#23485=CARTESIAN_POINT('Ctrl Pts',(206.974311678662,89.4647376084047,341.870426808548));
#23486=CARTESIAN_POINT('Ctrl Pts',(205.409498490334,89.4022376084047,342.851386355541));
#23487=CARTESIAN_POINT('Ctrl Pts',(203.844685302007,89.3397376084047,343.832345902533));
#23488=CARTESIAN_POINT('Ctrl Pts',(202.044552137503,89.2772376084047,343.419499033524));
#23489=CARTESIAN_POINT('Ctrl Pts',(202.044552137503,90.0272376084047,343.419499033524));
#23490=CARTESIAN_POINT('Ctrl Pts',(200.244418972999,89.9647376084047,343.006652164516));
#23491=CARTESIAN_POINT('Ctrl Pts',(199.263459426007,89.9022376084047,341.441838976189));
#23492=CARTESIAN_POINT('Ctrl Pts',(198.282499879015,89.8397376084047,339.877025787862));
#23493=CARTESIAN_POINT('Ctrl Pts',(198.695346748023,89.7772376084047,338.076892623358));
#23494=CARTESIAN_POINT('Ctrl Pts',(199.108193617031,89.7147376084047,336.276759458854));
#23495=CARTESIAN_POINT('Ctrl Pts',(200.673006805358,89.6522376084047,335.295799911861));
#23496=CARTESIAN_POINT('Ctrl Pts',(202.237819993686,89.5897376084047,334.314840364869));
#23497=CARTESIAN_POINT('Ctrl Pts',(204.03795315819,89.5272376084047,334.727687233877));
#23498=CARTESIAN_POINT('Ctrl Pts',(205.838086322694,89.4647376084047,335.140534102886));
#23499=CARTESIAN_POINT('Ctrl Pts',(206.819045869686,89.4022376084047,336.705347291213));
#23500=CARTESIAN_POINT('Ctrl Pts',(207.800005416678,89.3397376084047,338.27016047954));
#23501=CARTESIAN_POINT('Ctrl Pts',(207.38715854767,89.2772376084047,340.070293644044));
#23502=CARTESIAN_POINT('Ctrl Pts',(206.974311678662,89.2147376084047,341.870426808548));
#23503=CARTESIAN_POINT('Ctrl Pts',(205.409498490334,89.1522376084047,342.851386355541));
#23504=CARTESIAN_POINT('Ctrl Pts',(203.844685302007,89.0897376084047,343.832345902533));
#23505=CARTESIAN_POINT('Ctrl Pts',(202.044552137503,89.0272376084047,343.419499033524));
#23506=CARTESIAN_POINT('Origin',(203.041252647847,101.652237608405,339.0735931337));
#23507=CARTESIAN_POINT('',(202.044552137503,91.2772376084047,343.419499033524));
#23508=CARTESIAN_POINT('',(202.044552137503,91.0272376084047,343.419499033524));
#23509=CARTESIAN_POINT('',(202.044552137504,101.652237608405,343.419499033523));
#23510=CARTESIAN_POINT('Ctrl Pts',(202.044552137503,91.2772376084047,343.419499033524));
#23511=CARTESIAN_POINT('Ctrl Pts',(200.244418972999,91.2147376084047,343.006652164516));
#23512=CARTESIAN_POINT('Ctrl Pts',(199.263459426007,91.1522376084047,341.441838976189));
#23513=CARTESIAN_POINT('Ctrl Pts',(198.282499879015,91.0897376084047,339.877025787862));
#23514=CARTESIAN_POINT('Ctrl Pts',(198.695346748023,91.0272376084047,338.076892623358));
#23515=CARTESIAN_POINT('Ctrl Pts',(199.108193617031,90.9647376084047,336.276759458854));
#23516=CARTESIAN_POINT('Ctrl Pts',(200.673006805358,90.9022376084047,335.295799911861));
#23517=CARTESIAN_POINT('Ctrl Pts',(202.237819993686,90.8397376084047,334.314840364869));
#23518=CARTESIAN_POINT('Ctrl Pts',(204.03795315819,90.7772376084047,334.727687233877));
#23519=CARTESIAN_POINT('Ctrl Pts',(205.838086322694,90.7147376084047,335.140534102886));
#23520=CARTESIAN_POINT('Ctrl Pts',(206.819045869686,90.6522376084047,336.705347291213));
#23521=CARTESIAN_POINT('Ctrl Pts',(207.800005416678,90.5897376084047,338.27016047954));
#23522=CARTESIAN_POINT('Ctrl Pts',(207.38715854767,90.5272376084047,340.070293644044));
#23523=CARTESIAN_POINT('Ctrl Pts',(206.974311678662,90.4647376084047,341.870426808548));
#23524=CARTESIAN_POINT('Ctrl Pts',(205.409498490334,90.4022376084047,342.851386355541));
#23525=CARTESIAN_POINT('Ctrl Pts',(203.844685302007,90.3397376084047,343.832345902533));
#23526=CARTESIAN_POINT('Ctrl Pts',(202.044552137503,90.2772376084047,343.419499033524));
#23527=CARTESIAN_POINT('Ctrl Pts',(202.044552137503,91.0272376084047,343.419499033524));
#23528=CARTESIAN_POINT('Ctrl Pts',(200.244418972999,90.9647376084047,343.006652164516));
#23529=CARTESIAN_POINT('Ctrl Pts',(199.263459426007,90.9022376084047,341.441838976189));
#23530=CARTESIAN_POINT('Ctrl Pts',(198.282499879015,90.8397376084047,339.877025787862));
#23531=CARTESIAN_POINT('Ctrl Pts',(198.695346748023,90.7772376084047,338.076892623358));
#23532=CARTESIAN_POINT('Ctrl Pts',(199.108193617031,90.7147376084047,336.276759458854));
#23533=CARTESIAN_POINT('Ctrl Pts',(200.673006805358,90.6522376084047,335.295799911861));
#23534=CARTESIAN_POINT('Ctrl Pts',(202.237819993686,90.5897376084047,334.314840364869));
#23535=CARTESIAN_POINT('Ctrl Pts',(204.03795315819,90.5272376084047,334.727687233877));
#23536=CARTESIAN_POINT('Ctrl Pts',(205.838086322694,90.4647376084047,335.140534102886));
#23537=CARTESIAN_POINT('Ctrl Pts',(206.819045869686,90.4022376084047,336.705347291213));
#23538=CARTESIAN_POINT('Ctrl Pts',(207.800005416678,90.3397376084047,338.27016047954));
#23539=CARTESIAN_POINT('Ctrl Pts',(207.38715854767,90.2772376084047,340.070293644044));
#23540=CARTESIAN_POINT('Ctrl Pts',(206.974311678662,90.2147376084047,341.870426808548));
#23541=CARTESIAN_POINT('Ctrl Pts',(205.409498490334,90.1522376084047,342.851386355541));
#23542=CARTESIAN_POINT('Ctrl Pts',(203.844685302007,90.0897376084047,343.832345902533));
#23543=CARTESIAN_POINT('Ctrl Pts',(202.044552137503,90.0272376084047,343.419499033524));
#23544=CARTESIAN_POINT('Origin',(203.041252647847,101.652237608405,339.0735931337));
#23545=CARTESIAN_POINT('',(202.044552137503,92.2772376084047,343.419499033524));
#23546=CARTESIAN_POINT('',(202.044552137503,92.0272376084047,343.419499033524));
#23547=CARTESIAN_POINT('',(202.044552137504,101.652237608405,343.419499033523));
#23548=CARTESIAN_POINT('Ctrl Pts',(202.044552137503,92.2772376084047,343.419499033524));
#23549=CARTESIAN_POINT('Ctrl Pts',(200.244418972999,92.2147376084047,343.006652164516));
#23550=CARTESIAN_POINT('Ctrl Pts',(199.263459426007,92.1522376084047,341.441838976189));
#23551=CARTESIAN_POINT('Ctrl Pts',(198.282499879015,92.0897376084047,339.877025787862));
#23552=CARTESIAN_POINT('Ctrl Pts',(198.695346748023,92.0272376084047,338.076892623358));
#23553=CARTESIAN_POINT('Ctrl Pts',(199.108193617031,91.9647376084047,336.276759458854));
#23554=CARTESIAN_POINT('Ctrl Pts',(200.673006805358,91.9022376084047,335.295799911861));
#23555=CARTESIAN_POINT('Ctrl Pts',(202.237819993686,91.8397376084047,334.314840364869));
#23556=CARTESIAN_POINT('Ctrl Pts',(204.03795315819,91.7772376084047,334.727687233877));
#23557=CARTESIAN_POINT('Ctrl Pts',(205.838086322694,91.7147376084047,335.140534102886));
#23558=CARTESIAN_POINT('Ctrl Pts',(206.819045869686,91.6522376084047,336.705347291213));
#23559=CARTESIAN_POINT('Ctrl Pts',(207.800005416678,91.5897376084047,338.27016047954));
#23560=CARTESIAN_POINT('Ctrl Pts',(207.38715854767,91.5272376084047,340.070293644044));
#23561=CARTESIAN_POINT('Ctrl Pts',(206.974311678662,91.4647376084047,341.870426808548));
#23562=CARTESIAN_POINT('Ctrl Pts',(205.409498490334,91.4022376084047,342.851386355541));
#23563=CARTESIAN_POINT('Ctrl Pts',(203.844685302007,91.3397376084047,343.832345902533));
#23564=CARTESIAN_POINT('Ctrl Pts',(202.044552137503,91.2772376084047,343.419499033524));
#23565=CARTESIAN_POINT('Ctrl Pts',(202.044552137503,92.0272376084047,343.419499033524));
#23566=CARTESIAN_POINT('Ctrl Pts',(200.244418972999,91.9647376084047,343.006652164516));
#23567=CARTESIAN_POINT('Ctrl Pts',(199.263459426007,91.9022376084047,341.441838976189));
#23568=CARTESIAN_POINT('Ctrl Pts',(198.282499879015,91.8397376084047,339.877025787862));
#23569=CARTESIAN_POINT('Ctrl Pts',(198.695346748023,91.7772376084047,338.076892623358));
#23570=CARTESIAN_POINT('Ctrl Pts',(199.108193617031,91.7147376084047,336.276759458854));
#23571=CARTESIAN_POINT('Ctrl Pts',(200.673006805358,91.6522376084047,335.295799911861));
#23572=CARTESIAN_POINT('Ctrl Pts',(202.237819993686,91.5897376084047,334.314840364869));
#23573=CARTESIAN_POINT('Ctrl Pts',(204.03795315819,91.5272376084047,334.727687233877));
#23574=CARTESIAN_POINT('Ctrl Pts',(205.838086322694,91.4647376084047,335.140534102886));
#23575=CARTESIAN_POINT('Ctrl Pts',(206.819045869686,91.4022376084047,336.705347291213));
#23576=CARTESIAN_POINT('Ctrl Pts',(207.800005416678,91.3397376084047,338.27016047954));
#23577=CARTESIAN_POINT('Ctrl Pts',(207.38715854767,91.2772376084047,340.070293644044));
#23578=CARTESIAN_POINT('Ctrl Pts',(206.974311678662,91.2147376084047,341.870426808548));
#23579=CARTESIAN_POINT('Ctrl Pts',(205.409498490334,91.1522376084047,342.851386355541));
#23580=CARTESIAN_POINT('Ctrl Pts',(203.844685302007,91.0897376084047,343.832345902533));
#23581=CARTESIAN_POINT('Ctrl Pts',(202.044552137503,91.0272376084047,343.419499033524));
#23582=CARTESIAN_POINT('Origin',(203.041252647847,101.652237608405,339.0735931337));
#23583=CARTESIAN_POINT('',(202.044552137503,93.2772376084047,343.419499033524));
#23584=CARTESIAN_POINT('',(202.044552137503,93.0272376084047,343.419499033524));
#23585=CARTESIAN_POINT('',(202.044552137504,101.652237608405,343.419499033523));
#23586=CARTESIAN_POINT('Ctrl Pts',(202.044552137503,93.2772376084047,343.419499033524));
#23587=CARTESIAN_POINT('Ctrl Pts',(200.244418972999,93.2147376084047,343.006652164516));
#23588=CARTESIAN_POINT('Ctrl Pts',(199.263459426007,93.1522376084047,341.441838976189));
#23589=CARTESIAN_POINT('Ctrl Pts',(198.282499879015,93.0897376084047,339.877025787862));
#23590=CARTESIAN_POINT('Ctrl Pts',(198.695346748023,93.0272376084047,338.076892623358));
#23591=CARTESIAN_POINT('Ctrl Pts',(199.108193617031,92.9647376084047,336.276759458854));
#23592=CARTESIAN_POINT('Ctrl Pts',(200.673006805358,92.9022376084047,335.295799911861));
#23593=CARTESIAN_POINT('Ctrl Pts',(202.237819993686,92.8397376084047,334.314840364869));
#23594=CARTESIAN_POINT('Ctrl Pts',(204.03795315819,92.7772376084047,334.727687233877));
#23595=CARTESIAN_POINT('Ctrl Pts',(205.838086322694,92.7147376084047,335.140534102886));
#23596=CARTESIAN_POINT('Ctrl Pts',(206.819045869686,92.6522376084047,336.705347291213));
#23597=CARTESIAN_POINT('Ctrl Pts',(207.800005416678,92.5897376084047,338.27016047954));
#23598=CARTESIAN_POINT('Ctrl Pts',(207.38715854767,92.5272376084047,340.070293644044));
#23599=CARTESIAN_POINT('Ctrl Pts',(206.974311678662,92.4647376084047,341.870426808548));
#23600=CARTESIAN_POINT('Ctrl Pts',(205.409498490334,92.4022376084047,342.851386355541));
#23601=CARTESIAN_POINT('Ctrl Pts',(203.844685302007,92.3397376084047,343.832345902533));
#23602=CARTESIAN_POINT('Ctrl Pts',(202.044552137503,92.2772376084047,343.419499033524));
#23603=CARTESIAN_POINT('Ctrl Pts',(202.044552137503,93.0272376084047,343.419499033524));
#23604=CARTESIAN_POINT('Ctrl Pts',(200.244418972999,92.9647376084047,343.006652164516));
#23605=CARTESIAN_POINT('Ctrl Pts',(199.263459426007,92.9022376084047,341.441838976189));
#23606=CARTESIAN_POINT('Ctrl Pts',(198.282499879015,92.8397376084047,339.877025787862));
#23607=CARTESIAN_POINT('Ctrl Pts',(198.695346748023,92.7772376084047,338.076892623358));
#23608=CARTESIAN_POINT('Ctrl Pts',(199.108193617031,92.7147376084047,336.276759458854));
#23609=CARTESIAN_POINT('Ctrl Pts',(200.673006805358,92.6522376084047,335.295799911861));
#23610=CARTESIAN_POINT('Ctrl Pts',(202.237819993686,92.5897376084047,334.314840364869));
#23611=CARTESIAN_POINT('Ctrl Pts',(204.03795315819,92.5272376084047,334.727687233877));
#23612=CARTESIAN_POINT('Ctrl Pts',(205.838086322694,92.4647376084047,335.140534102886));
#23613=CARTESIAN_POINT('Ctrl Pts',(206.819045869686,92.4022376084047,336.705347291213));
#23614=CARTESIAN_POINT('Ctrl Pts',(207.800005416678,92.3397376084047,338.27016047954));
#23615=CARTESIAN_POINT('Ctrl Pts',(207.38715854767,92.2772376084047,340.070293644044));
#23616=CARTESIAN_POINT('Ctrl Pts',(206.974311678662,92.2147376084047,341.870426808548));
#23617=CARTESIAN_POINT('Ctrl Pts',(205.409498490334,92.1522376084047,342.851386355541));
#23618=CARTESIAN_POINT('Ctrl Pts',(203.844685302007,92.0897376084047,343.832345902533));
#23619=CARTESIAN_POINT('Ctrl Pts',(202.044552137503,92.0272376084047,343.419499033524));
#23620=CARTESIAN_POINT('Origin',(203.041252647847,101.652237608405,339.0735931337));
#23621=CARTESIAN_POINT('',(202.044552137503,94.2772376084047,343.419499033524));
#23622=CARTESIAN_POINT('',(202.044552137503,94.0272376084047,343.419499033524));
#23623=CARTESIAN_POINT('',(202.044552137504,101.652237608405,343.419499033523));
#23624=CARTESIAN_POINT('Ctrl Pts',(202.044552137503,94.2772376084047,343.419499033524));
#23625=CARTESIAN_POINT('Ctrl Pts',(200.244418972999,94.2147376084047,343.006652164516));
#23626=CARTESIAN_POINT('Ctrl Pts',(199.263459426007,94.1522376084047,341.441838976189));
#23627=CARTESIAN_POINT('Ctrl Pts',(198.282499879015,94.0897376084047,339.877025787862));
#23628=CARTESIAN_POINT('Ctrl Pts',(198.695346748023,94.0272376084047,338.076892623358));
#23629=CARTESIAN_POINT('Ctrl Pts',(199.108193617031,93.9647376084047,336.276759458854));
#23630=CARTESIAN_POINT('Ctrl Pts',(200.673006805358,93.9022376084047,335.295799911861));
#23631=CARTESIAN_POINT('Ctrl Pts',(202.237819993686,93.8397376084047,334.314840364869));
#23632=CARTESIAN_POINT('Ctrl Pts',(204.03795315819,93.7772376084047,334.727687233877));
#23633=CARTESIAN_POINT('Ctrl Pts',(205.838086322694,93.7147376084047,335.140534102886));
#23634=CARTESIAN_POINT('Ctrl Pts',(206.819045869686,93.6522376084047,336.705347291213));
#23635=CARTESIAN_POINT('Ctrl Pts',(207.800005416678,93.5897376084047,338.27016047954));
#23636=CARTESIAN_POINT('Ctrl Pts',(207.38715854767,93.5272376084047,340.070293644044));
#23637=CARTESIAN_POINT('Ctrl Pts',(206.974311678662,93.4647376084047,341.870426808548));
#23638=CARTESIAN_POINT('Ctrl Pts',(205.409498490334,93.4022376084047,342.851386355541));
#23639=CARTESIAN_POINT('Ctrl Pts',(203.844685302007,93.3397376084047,343.832345902533));
#23640=CARTESIAN_POINT('Ctrl Pts',(202.044552137503,93.2772376084047,343.419499033524));
#23641=CARTESIAN_POINT('Ctrl Pts',(202.044552137503,94.0272376084047,343.419499033524));
#23642=CARTESIAN_POINT('Ctrl Pts',(200.244418972999,93.9647376084047,343.006652164516));
#23643=CARTESIAN_POINT('Ctrl Pts',(199.263459426007,93.9022376084047,341.441838976189));
#23644=CARTESIAN_POINT('Ctrl Pts',(198.282499879015,93.8397376084047,339.877025787862));
#23645=CARTESIAN_POINT('Ctrl Pts',(198.695346748023,93.7772376084047,338.076892623358));
#23646=CARTESIAN_POINT('Ctrl Pts',(199.108193617031,93.7147376084047,336.276759458854));
#23647=CARTESIAN_POINT('Ctrl Pts',(200.673006805358,93.6522376084047,335.295799911861));
#23648=CARTESIAN_POINT('Ctrl Pts',(202.237819993686,93.5897376084047,334.314840364869));
#23649=CARTESIAN_POINT('Ctrl Pts',(204.03795315819,93.5272376084047,334.727687233877));
#23650=CARTESIAN_POINT('Ctrl Pts',(205.838086322694,93.4647376084047,335.140534102886));
#23651=CARTESIAN_POINT('Ctrl Pts',(206.819045869686,93.4022376084047,336.705347291213));
#23652=CARTESIAN_POINT('Ctrl Pts',(207.800005416678,93.3397376084047,338.27016047954));
#23653=CARTESIAN_POINT('Ctrl Pts',(207.38715854767,93.2772376084047,340.070293644044));
#23654=CARTESIAN_POINT('Ctrl Pts',(206.974311678662,93.2147376084047,341.870426808548));
#23655=CARTESIAN_POINT('Ctrl Pts',(205.409498490334,93.1522376084047,342.851386355541));
#23656=CARTESIAN_POINT('Ctrl Pts',(203.844685302007,93.0897376084047,343.832345902533));
#23657=CARTESIAN_POINT('Ctrl Pts',(202.044552137503,93.0272376084047,343.419499033524));
#23658=CARTESIAN_POINT('Origin',(203.041252647847,101.652237608405,339.0735931337));
#23659=CARTESIAN_POINT('',(202.044552137503,95.2772376084047,343.419499033524));
#23660=CARTESIAN_POINT('',(202.044552137503,95.0272376084047,343.419499033524));
#23661=CARTESIAN_POINT('',(202.044552137504,101.652237608405,343.419499033523));
#23662=CARTESIAN_POINT('Ctrl Pts',(202.044552137503,95.2772376084047,343.419499033524));
#23663=CARTESIAN_POINT('Ctrl Pts',(200.244418972999,95.2147376084047,343.006652164516));
#23664=CARTESIAN_POINT('Ctrl Pts',(199.263459426007,95.1522376084047,341.441838976189));
#23665=CARTESIAN_POINT('Ctrl Pts',(198.282499879015,95.0897376084047,339.877025787862));
#23666=CARTESIAN_POINT('Ctrl Pts',(198.695346748023,95.0272376084047,338.076892623358));
#23667=CARTESIAN_POINT('Ctrl Pts',(199.108193617031,94.9647376084047,336.276759458854));
#23668=CARTESIAN_POINT('Ctrl Pts',(200.673006805358,94.9022376084047,335.295799911861));
#23669=CARTESIAN_POINT('Ctrl Pts',(202.237819993686,94.8397376084047,334.314840364869));
#23670=CARTESIAN_POINT('Ctrl Pts',(204.03795315819,94.7772376084047,334.727687233877));
#23671=CARTESIAN_POINT('Ctrl Pts',(205.838086322694,94.7147376084047,335.140534102886));
#23672=CARTESIAN_POINT('Ctrl Pts',(206.819045869686,94.6522376084047,336.705347291213));
#23673=CARTESIAN_POINT('Ctrl Pts',(207.800005416678,94.5897376084047,338.27016047954));
#23674=CARTESIAN_POINT('Ctrl Pts',(207.38715854767,94.5272376084047,340.070293644044));
#23675=CARTESIAN_POINT('Ctrl Pts',(206.974311678662,94.4647376084047,341.870426808548));
#23676=CARTESIAN_POINT('Ctrl Pts',(205.409498490334,94.4022376084047,342.851386355541));
#23677=CARTESIAN_POINT('Ctrl Pts',(203.844685302007,94.3397376084047,343.832345902533));
#23678=CARTESIAN_POINT('Ctrl Pts',(202.044552137503,94.2772376084047,343.419499033524));
#23679=CARTESIAN_POINT('Ctrl Pts',(202.044552137503,95.0272376084047,343.419499033524));
#23680=CARTESIAN_POINT('Ctrl Pts',(200.244418972999,94.9647376084047,343.006652164516));
#23681=CARTESIAN_POINT('Ctrl Pts',(199.263459426007,94.9022376084047,341.441838976189));
#23682=CARTESIAN_POINT('Ctrl Pts',(198.282499879015,94.8397376084047,339.877025787862));
#23683=CARTESIAN_POINT('Ctrl Pts',(198.695346748023,94.7772376084047,338.076892623358));
#23684=CARTESIAN_POINT('Ctrl Pts',(199.108193617031,94.7147376084047,336.276759458854));
#23685=CARTESIAN_POINT('Ctrl Pts',(200.673006805358,94.6522376084047,335.295799911861));
#23686=CARTESIAN_POINT('Ctrl Pts',(202.237819993686,94.5897376084047,334.314840364869));
#23687=CARTESIAN_POINT('Ctrl Pts',(204.03795315819,94.5272376084047,334.727687233877));
#23688=CARTESIAN_POINT('Ctrl Pts',(205.838086322694,94.4647376084047,335.140534102886));
#23689=CARTESIAN_POINT('Ctrl Pts',(206.819045869686,94.4022376084047,336.705347291213));
#23690=CARTESIAN_POINT('Ctrl Pts',(207.800005416678,94.3397376084047,338.27016047954));
#23691=CARTESIAN_POINT('Ctrl Pts',(207.38715854767,94.2772376084047,340.070293644044));
#23692=CARTESIAN_POINT('Ctrl Pts',(206.974311678662,94.2147376084047,341.870426808548));
#23693=CARTESIAN_POINT('Ctrl Pts',(205.409498490334,94.1522376084047,342.851386355541));
#23694=CARTESIAN_POINT('Ctrl Pts',(203.844685302007,94.0897376084047,343.832345902533));
#23695=CARTESIAN_POINT('Ctrl Pts',(202.044552137503,94.0272376084047,343.419499033524));
#23696=CARTESIAN_POINT('Origin',(203.041252647847,101.652237608405,339.0735931337));
#23697=CARTESIAN_POINT('',(202.044552137503,96.2772376084047,343.419499033524));
#23698=CARTESIAN_POINT('',(202.044552137503,96.0272376084047,343.419499033524));
#23699=CARTESIAN_POINT('',(202.044552137504,101.652237608405,343.419499033523));
#23700=CARTESIAN_POINT('Ctrl Pts',(202.044552137503,96.2772376084047,343.419499033524));
#23701=CARTESIAN_POINT('Ctrl Pts',(200.244418972999,96.2147376084047,343.006652164516));
#23702=CARTESIAN_POINT('Ctrl Pts',(199.263459426007,96.1522376084047,341.441838976189));
#23703=CARTESIAN_POINT('Ctrl Pts',(198.282499879015,96.0897376084047,339.877025787862));
#23704=CARTESIAN_POINT('Ctrl Pts',(198.695346748023,96.0272376084047,338.076892623358));
#23705=CARTESIAN_POINT('Ctrl Pts',(199.108193617031,95.9647376084047,336.276759458854));
#23706=CARTESIAN_POINT('Ctrl Pts',(200.673006805358,95.9022376084047,335.295799911861));
#23707=CARTESIAN_POINT('Ctrl Pts',(202.237819993686,95.8397376084047,334.314840364869));
#23708=CARTESIAN_POINT('Ctrl Pts',(204.03795315819,95.7772376084047,334.727687233877));
#23709=CARTESIAN_POINT('Ctrl Pts',(205.838086322694,95.7147376084047,335.140534102886));
#23710=CARTESIAN_POINT('Ctrl Pts',(206.819045869686,95.6522376084047,336.705347291213));
#23711=CARTESIAN_POINT('Ctrl Pts',(207.800005416678,95.5897376084047,338.27016047954));
#23712=CARTESIAN_POINT('Ctrl Pts',(207.38715854767,95.5272376084047,340.070293644044));
#23713=CARTESIAN_POINT('Ctrl Pts',(206.974311678662,95.4647376084047,341.870426808548));
#23714=CARTESIAN_POINT('Ctrl Pts',(205.409498490334,95.4022376084047,342.851386355541));
#23715=CARTESIAN_POINT('Ctrl Pts',(203.844685302007,95.3397376084047,343.832345902533));
#23716=CARTESIAN_POINT('Ctrl Pts',(202.044552137503,95.2772376084047,343.419499033524));
#23717=CARTESIAN_POINT('Ctrl Pts',(202.044552137503,96.0272376084047,343.419499033524));
#23718=CARTESIAN_POINT('Ctrl Pts',(200.244418972999,95.9647376084047,343.006652164516));
#23719=CARTESIAN_POINT('Ctrl Pts',(199.263459426007,95.9022376084047,341.441838976189));
#23720=CARTESIAN_POINT('Ctrl Pts',(198.282499879015,95.8397376084047,339.877025787862));
#23721=CARTESIAN_POINT('Ctrl Pts',(198.695346748023,95.7772376084047,338.076892623358));
#23722=CARTESIAN_POINT('Ctrl Pts',(199.108193617031,95.7147376084047,336.276759458854));
#23723=CARTESIAN_POINT('Ctrl Pts',(200.673006805358,95.6522376084047,335.295799911861));
#23724=CARTESIAN_POINT('Ctrl Pts',(202.237819993686,95.5897376084047,334.314840364869));
#23725=CARTESIAN_POINT('Ctrl Pts',(204.03795315819,95.5272376084047,334.727687233877));
#23726=CARTESIAN_POINT('Ctrl Pts',(205.838086322694,95.4647376084047,335.140534102886));
#23727=CARTESIAN_POINT('Ctrl Pts',(206.819045869686,95.4022376084047,336.705347291213));
#23728=CARTESIAN_POINT('Ctrl Pts',(207.800005416678,95.3397376084047,338.27016047954));
#23729=CARTESIAN_POINT('Ctrl Pts',(207.38715854767,95.2772376084047,340.070293644044));
#23730=CARTESIAN_POINT('Ctrl Pts',(206.974311678662,95.2147376084047,341.870426808548));
#23731=CARTESIAN_POINT('Ctrl Pts',(205.409498490334,95.1522376084047,342.851386355541));
#23732=CARTESIAN_POINT('Ctrl Pts',(203.844685302007,95.0897376084047,343.832345902533));
#23733=CARTESIAN_POINT('Ctrl Pts',(202.044552137503,95.0272376084047,343.419499033524));
#23734=CARTESIAN_POINT('Origin',(203.041252647847,101.652237608405,339.0735931337));
#23735=CARTESIAN_POINT('',(202.044552137503,97.2772376084047,343.419499033524));
#23736=CARTESIAN_POINT('',(202.044552137503,97.0272376084047,343.419499033524));
#23737=CARTESIAN_POINT('',(202.044552137504,101.652237608405,343.419499033523));
#23738=CARTESIAN_POINT('Ctrl Pts',(202.044552137503,97.2772376084047,343.419499033524));
#23739=CARTESIAN_POINT('Ctrl Pts',(200.244418972999,97.2147376084047,343.006652164516));
#23740=CARTESIAN_POINT('Ctrl Pts',(199.263459426007,97.1522376084047,341.441838976189));
#23741=CARTESIAN_POINT('Ctrl Pts',(198.282499879015,97.0897376084047,339.877025787862));
#23742=CARTESIAN_POINT('Ctrl Pts',(198.695346748023,97.0272376084047,338.076892623358));
#23743=CARTESIAN_POINT('Ctrl Pts',(199.108193617031,96.9647376084047,336.276759458854));
#23744=CARTESIAN_POINT('Ctrl Pts',(200.673006805358,96.9022376084047,335.295799911861));
#23745=CARTESIAN_POINT('Ctrl Pts',(202.237819993686,96.8397376084047,334.314840364869));
#23746=CARTESIAN_POINT('Ctrl Pts',(204.03795315819,96.7772376084047,334.727687233877));
#23747=CARTESIAN_POINT('Ctrl Pts',(205.838086322694,96.7147376084047,335.140534102886));
#23748=CARTESIAN_POINT('Ctrl Pts',(206.819045869686,96.6522376084047,336.705347291213));
#23749=CARTESIAN_POINT('Ctrl Pts',(207.800005416678,96.5897376084047,338.27016047954));
#23750=CARTESIAN_POINT('Ctrl Pts',(207.38715854767,96.5272376084047,340.070293644044));
#23751=CARTESIAN_POINT('Ctrl Pts',(206.974311678662,96.4647376084047,341.870426808548));
#23752=CARTESIAN_POINT('Ctrl Pts',(205.409498490334,96.4022376084047,342.851386355541));
#23753=CARTESIAN_POINT('Ctrl Pts',(203.844685302007,96.3397376084047,343.832345902533));
#23754=CARTESIAN_POINT('Ctrl Pts',(202.044552137503,96.2772376084047,343.419499033524));
#23755=CARTESIAN_POINT('Ctrl Pts',(202.044552137503,97.0272376084047,343.419499033524));
#23756=CARTESIAN_POINT('Ctrl Pts',(200.244418972999,96.9647376084047,343.006652164516));
#23757=CARTESIAN_POINT('Ctrl Pts',(199.263459426007,96.9022376084047,341.441838976189));
#23758=CARTESIAN_POINT('Ctrl Pts',(198.282499879015,96.8397376084047,339.877025787862));
#23759=CARTESIAN_POINT('Ctrl Pts',(198.695346748023,96.7772376084047,338.076892623358));
#23760=CARTESIAN_POINT('Ctrl Pts',(199.108193617031,96.7147376084047,336.276759458854));
#23761=CARTESIAN_POINT('Ctrl Pts',(200.673006805358,96.6522376084047,335.295799911861));
#23762=CARTESIAN_POINT('Ctrl Pts',(202.237819993686,96.5897376084047,334.314840364869));
#23763=CARTESIAN_POINT('Ctrl Pts',(204.03795315819,96.5272376084047,334.727687233877));
#23764=CARTESIAN_POINT('Ctrl Pts',(205.838086322694,96.4647376084047,335.140534102886));
#23765=CARTESIAN_POINT('Ctrl Pts',(206.819045869686,96.4022376084047,336.705347291213));
#23766=CARTESIAN_POINT('Ctrl Pts',(207.800005416678,96.3397376084047,338.27016047954));
#23767=CARTESIAN_POINT('Ctrl Pts',(207.38715854767,96.2772376084047,340.070293644044));
#23768=CARTESIAN_POINT('Ctrl Pts',(206.974311678662,96.2147376084047,341.870426808548));
#23769=CARTESIAN_POINT('Ctrl Pts',(205.409498490334,96.1522376084047,342.851386355541));
#23770=CARTESIAN_POINT('Ctrl Pts',(203.844685302007,96.0897376084047,343.832345902533));
#23771=CARTESIAN_POINT('Ctrl Pts',(202.044552137503,96.0272376084047,343.419499033524));
#23772=CARTESIAN_POINT('Origin',(203.041252647847,101.652237608405,339.0735931337));
#23773=CARTESIAN_POINT('',(202.044552137503,98.2772376084047,343.419499033524));
#23774=CARTESIAN_POINT('',(202.044552137503,98.0272376084047,343.419499033524));
#23775=CARTESIAN_POINT('',(202.044552137504,101.652237608405,343.419499033523));
#23776=CARTESIAN_POINT('Ctrl Pts',(202.044552137503,98.2772376084047,343.419499033524));
#23777=CARTESIAN_POINT('Ctrl Pts',(200.244418972999,98.2147376084047,343.006652164516));
#23778=CARTESIAN_POINT('Ctrl Pts',(199.263459426007,98.1522376084047,341.441838976189));
#23779=CARTESIAN_POINT('Ctrl Pts',(198.282499879015,98.0897376084047,339.877025787862));
#23780=CARTESIAN_POINT('Ctrl Pts',(198.695346748023,98.0272376084047,338.076892623358));
#23781=CARTESIAN_POINT('Ctrl Pts',(199.108193617031,97.9647376084047,336.276759458854));
#23782=CARTESIAN_POINT('Ctrl Pts',(200.673006805358,97.9022376084047,335.295799911861));
#23783=CARTESIAN_POINT('Ctrl Pts',(202.237819993686,97.8397376084047,334.314840364869));
#23784=CARTESIAN_POINT('Ctrl Pts',(204.03795315819,97.7772376084047,334.727687233877));
#23785=CARTESIAN_POINT('Ctrl Pts',(205.838086322694,97.7147376084047,335.140534102886));
#23786=CARTESIAN_POINT('Ctrl Pts',(206.819045869686,97.6522376084047,336.705347291213));
#23787=CARTESIAN_POINT('Ctrl Pts',(207.800005416678,97.5897376084047,338.27016047954));
#23788=CARTESIAN_POINT('Ctrl Pts',(207.38715854767,97.5272376084047,340.070293644044));
#23789=CARTESIAN_POINT('Ctrl Pts',(206.974311678662,97.4647376084047,341.870426808548));
#23790=CARTESIAN_POINT('Ctrl Pts',(205.409498490334,97.4022376084047,342.851386355541));
#23791=CARTESIAN_POINT('Ctrl Pts',(203.844685302007,97.3397376084047,343.832345902533));
#23792=CARTESIAN_POINT('Ctrl Pts',(202.044552137503,97.2772376084047,343.419499033524));
#23793=CARTESIAN_POINT('Ctrl Pts',(202.044552137503,98.0272376084047,343.419499033524));
#23794=CARTESIAN_POINT('Ctrl Pts',(200.244418972999,97.9647376084047,343.006652164516));
#23795=CARTESIAN_POINT('Ctrl Pts',(199.263459426007,97.9022376084047,341.441838976189));
#23796=CARTESIAN_POINT('Ctrl Pts',(198.282499879015,97.8397376084047,339.877025787862));
#23797=CARTESIAN_POINT('Ctrl Pts',(198.695346748023,97.7772376084047,338.076892623358));
#23798=CARTESIAN_POINT('Ctrl Pts',(199.108193617031,97.7147376084047,336.276759458854));
#23799=CARTESIAN_POINT('Ctrl Pts',(200.673006805358,97.6522376084047,335.295799911861));
#23800=CARTESIAN_POINT('Ctrl Pts',(202.237819993686,97.5897376084047,334.314840364869));
#23801=CARTESIAN_POINT('Ctrl Pts',(204.03795315819,97.5272376084047,334.727687233877));
#23802=CARTESIAN_POINT('Ctrl Pts',(205.838086322694,97.4647376084047,335.140534102886));
#23803=CARTESIAN_POINT('Ctrl Pts',(206.819045869686,97.4022376084047,336.705347291213));
#23804=CARTESIAN_POINT('Ctrl Pts',(207.800005416678,97.3397376084047,338.27016047954));
#23805=CARTESIAN_POINT('Ctrl Pts',(207.38715854767,97.2772376084047,340.070293644044));
#23806=CARTESIAN_POINT('Ctrl Pts',(206.974311678662,97.2147376084047,341.870426808548));
#23807=CARTESIAN_POINT('Ctrl Pts',(205.409498490334,97.1522376084047,342.851386355541));
#23808=CARTESIAN_POINT('Ctrl Pts',(203.844685302007,97.0897376084047,343.832345902533));
#23809=CARTESIAN_POINT('Ctrl Pts',(202.044552137503,97.0272376084047,343.419499033524));
#23810=CARTESIAN_POINT('Origin',(203.041252647847,101.652237608405,339.0735931337));
#23811=CARTESIAN_POINT('',(202.044552137503,99.2772376084047,343.419499033524));
#23812=CARTESIAN_POINT('',(202.044552137503,99.0272376084047,343.419499033524));
#23813=CARTESIAN_POINT('',(202.044552137504,101.652237608405,343.419499033523));
#23814=CARTESIAN_POINT('Ctrl Pts',(202.044552137503,99.2772376084047,343.419499033524));
#23815=CARTESIAN_POINT('Ctrl Pts',(200.244418972999,99.2147376084047,343.006652164516));
#23816=CARTESIAN_POINT('Ctrl Pts',(199.263459426007,99.1522376084047,341.441838976189));
#23817=CARTESIAN_POINT('Ctrl Pts',(198.282499879015,99.0897376084047,339.877025787862));
#23818=CARTESIAN_POINT('Ctrl Pts',(198.695346748023,99.0272376084047,338.076892623358));
#23819=CARTESIAN_POINT('Ctrl Pts',(199.108193617031,98.9647376084047,336.276759458854));
#23820=CARTESIAN_POINT('Ctrl Pts',(200.673006805358,98.9022376084047,335.295799911861));
#23821=CARTESIAN_POINT('Ctrl Pts',(202.237819993686,98.8397376084047,334.314840364869));
#23822=CARTESIAN_POINT('Ctrl Pts',(204.03795315819,98.7772376084047,334.727687233877));
#23823=CARTESIAN_POINT('Ctrl Pts',(205.838086322694,98.7147376084047,335.140534102886));
#23824=CARTESIAN_POINT('Ctrl Pts',(206.819045869686,98.6522376084047,336.705347291213));
#23825=CARTESIAN_POINT('Ctrl Pts',(207.800005416678,98.5897376084047,338.27016047954));
#23826=CARTESIAN_POINT('Ctrl Pts',(207.38715854767,98.5272376084047,340.070293644044));
#23827=CARTESIAN_POINT('Ctrl Pts',(206.974311678662,98.4647376084047,341.870426808548));
#23828=CARTESIAN_POINT('Ctrl Pts',(205.409498490334,98.4022376084047,342.851386355541));
#23829=CARTESIAN_POINT('Ctrl Pts',(203.844685302007,98.3397376084047,343.832345902533));
#23830=CARTESIAN_POINT('Ctrl Pts',(202.044552137503,98.2772376084047,343.419499033524));
#23831=CARTESIAN_POINT('Ctrl Pts',(202.044552137503,99.0272376084047,343.419499033524));
#23832=CARTESIAN_POINT('Ctrl Pts',(200.244418972999,98.9647376084047,343.006652164516));
#23833=CARTESIAN_POINT('Ctrl Pts',(199.263459426007,98.9022376084047,341.441838976189));
#23834=CARTESIAN_POINT('Ctrl Pts',(198.282499879015,98.8397376084047,339.877025787862));
#23835=CARTESIAN_POINT('Ctrl Pts',(198.695346748023,98.7772376084047,338.076892623358));
#23836=CARTESIAN_POINT('Ctrl Pts',(199.108193617031,98.7147376084047,336.276759458854));
#23837=CARTESIAN_POINT('Ctrl Pts',(200.673006805358,98.6522376084047,335.295799911861));
#23838=CARTESIAN_POINT('Ctrl Pts',(202.237819993686,98.5897376084047,334.314840364869));
#23839=CARTESIAN_POINT('Ctrl Pts',(204.03795315819,98.5272376084047,334.727687233877));
#23840=CARTESIAN_POINT('Ctrl Pts',(205.838086322694,98.4647376084047,335.140534102886));
#23841=CARTESIAN_POINT('Ctrl Pts',(206.819045869686,98.4022376084047,336.705347291213));
#23842=CARTESIAN_POINT('Ctrl Pts',(207.800005416678,98.3397376084047,338.27016047954));
#23843=CARTESIAN_POINT('Ctrl Pts',(207.38715854767,98.2772376084047,340.070293644044));
#23844=CARTESIAN_POINT('Ctrl Pts',(206.974311678662,98.2147376084047,341.870426808548));
#23845=CARTESIAN_POINT('Ctrl Pts',(205.409498490334,98.1522376084047,342.851386355541));
#23846=CARTESIAN_POINT('Ctrl Pts',(203.844685302007,98.0897376084047,343.832345902533));
#23847=CARTESIAN_POINT('Ctrl Pts',(202.044552137503,98.0272376084047,343.419499033524));
#23848=CARTESIAN_POINT('Origin',(203.041252647847,101.652237608405,339.0735931337));
#23849=CARTESIAN_POINT('',(202.044552137503,100.277237608405,343.419499033524));
#23850=CARTESIAN_POINT('',(202.044552137503,100.027237608405,343.419499033524));
#23851=CARTESIAN_POINT('',(202.044552137504,101.652237608405,343.419499033523));
#23852=CARTESIAN_POINT('Ctrl Pts',(202.044552137503,100.277237608405,343.419499033524));
#23853=CARTESIAN_POINT('Ctrl Pts',(200.244418972999,100.214737608405,343.006652164516));
#23854=CARTESIAN_POINT('Ctrl Pts',(199.263459426007,100.152237608405,341.441838976189));
#23855=CARTESIAN_POINT('Ctrl Pts',(198.282499879015,100.089737608405,339.877025787862));
#23856=CARTESIAN_POINT('Ctrl Pts',(198.695346748023,100.027237608405,338.076892623358));
#23857=CARTESIAN_POINT('Ctrl Pts',(199.108193617031,99.9647376084047,336.276759458854));
#23858=CARTESIAN_POINT('Ctrl Pts',(200.673006805358,99.9022376084047,335.295799911861));
#23859=CARTESIAN_POINT('Ctrl Pts',(202.237819993686,99.8397376084047,334.314840364869));
#23860=CARTESIAN_POINT('Ctrl Pts',(204.03795315819,99.7772376084047,334.727687233877));
#23861=CARTESIAN_POINT('Ctrl Pts',(205.838086322694,99.7147376084047,335.140534102886));
#23862=CARTESIAN_POINT('Ctrl Pts',(206.819045869686,99.6522376084047,336.705347291213));
#23863=CARTESIAN_POINT('Ctrl Pts',(207.800005416678,99.5897376084047,338.27016047954));
#23864=CARTESIAN_POINT('Ctrl Pts',(207.38715854767,99.5272376084047,340.070293644044));
#23865=CARTESIAN_POINT('Ctrl Pts',(206.974311678662,99.4647376084047,341.870426808548));
#23866=CARTESIAN_POINT('Ctrl Pts',(205.409498490334,99.4022376084047,342.851386355541));
#23867=CARTESIAN_POINT('Ctrl Pts',(203.844685302007,99.3397376084047,343.832345902533));
#23868=CARTESIAN_POINT('Ctrl Pts',(202.044552137503,99.2772376084047,343.419499033524));
#23869=CARTESIAN_POINT('Ctrl Pts',(202.044552137503,100.027237608405,343.419499033524));
#23870=CARTESIAN_POINT('Ctrl Pts',(200.244418972999,99.9647376084047,343.006652164516));
#23871=CARTESIAN_POINT('Ctrl Pts',(199.263459426007,99.9022376084047,341.441838976189));
#23872=CARTESIAN_POINT('Ctrl Pts',(198.282499879015,99.8397376084047,339.877025787862));
#23873=CARTESIAN_POINT('Ctrl Pts',(198.695346748023,99.7772376084047,338.076892623358));
#23874=CARTESIAN_POINT('Ctrl Pts',(199.108193617031,99.7147376084047,336.276759458854));
#23875=CARTESIAN_POINT('Ctrl Pts',(200.673006805358,99.6522376084047,335.295799911861));
#23876=CARTESIAN_POINT('Ctrl Pts',(202.237819993686,99.5897376084047,334.314840364869));
#23877=CARTESIAN_POINT('Ctrl Pts',(204.03795315819,99.5272376084047,334.727687233877));
#23878=CARTESIAN_POINT('Ctrl Pts',(205.838086322694,99.4647376084047,335.140534102886));
#23879=CARTESIAN_POINT('Ctrl Pts',(206.819045869686,99.4022376084047,336.705347291213));
#23880=CARTESIAN_POINT('Ctrl Pts',(207.800005416678,99.3397376084047,338.27016047954));
#23881=CARTESIAN_POINT('Ctrl Pts',(207.38715854767,99.2772376084047,340.070293644044));
#23882=CARTESIAN_POINT('Ctrl Pts',(206.974311678662,99.2147376084047,341.870426808548));
#23883=CARTESIAN_POINT('Ctrl Pts',(205.409498490334,99.1522376084047,342.851386355541));
#23884=CARTESIAN_POINT('Ctrl Pts',(203.844685302007,99.0897376084047,343.832345902533));
#23885=CARTESIAN_POINT('Ctrl Pts',(202.044552137503,99.0272376084047,343.419499033524));
#23886=CARTESIAN_POINT('Origin',(203.041252647846,100.739737607039,339.073593133701));
#23887=CARTESIAN_POINT('',(207.914727694784,88.9647376097703,340.191287620971));
#23888=CARTESIAN_POINT('',(207.914727694784,88.8397376070391,340.191287620971));
#23889=CARTESIAN_POINT('',(207.914727694784,100.739737607039,340.191287620971));
#23890=CARTESIAN_POINT('',(207.914727694784,87.9647376097703,340.191287620971));
#23891=CARTESIAN_POINT('Ctrl Pts',(207.914727694784,88.9647376097703,340.191287620971));
#23892=CARTESIAN_POINT('Ctrl Pts',(207.770753734705,88.9453011777326,340.819056219497));
#23893=CARTESIAN_POINT('Ctrl Pts',(207.506770801709,88.9244834292568,341.413375945422));
#23894=CARTESIAN_POINT('Ctrl Pts',(206.767868521896,88.8824038680257,342.468698351296));
#23895=CARTESIAN_POINT('Ctrl Pts',(206.30024443967,88.8615432713098,342.919816661895));
#23896=CARTESIAN_POINT('Ctrl Pts',(205.201281739421,88.8217871525201,343.63181433124));
#23897=CARTESIAN_POINT('Ctrl Pts',(204.575887476526,88.8005368278284,343.878602026753));
#23898=CARTESIAN_POINT('Ctrl Pts',(203.286672824674,88.7577611328256,344.10890345328));
#23899=CARTESIAN_POINT('Ctrl Pts',(202.636859979253,88.7368875976579,344.098640860192));
#23900=CARTESIAN_POINT('Ctrl Pts',(201.355999128455,88.6971060741293,343.827800694488));
#23901=CARTESIAN_POINT('Ctrl Pts',(200.739055575249,88.6759104064177,343.561639678486));
#23902=CARTESIAN_POINT('Ctrl Pts',(199.663036126355,88.6331442992501,342.815574264922));
#23903=CARTESIAN_POINT('Ctrl Pts',(199.209615349934,88.6122569948317,342.349777136382));
#23904=CARTESIAN_POINT('Ctrl Pts',(198.493072284917,88.5724483372744,341.254430931273));
#23905=CARTESIAN_POINT('Ctrl Pts',(198.243690702334,88.5513105760968,340.630993961543));
#23906=CARTESIAN_POINT('Ctrl Pts',(198.007154195593,88.5085548963122,339.343453425775));
#23907=CARTESIAN_POINT('Ctrl Pts',(198.014285869939,88.4876529600333,338.693287385656));
#23908=CARTESIAN_POINT('Ctrl Pts',(198.278942152579,88.4478153546861,337.411729351262));
#23909=CARTESIAN_POINT('Ctrl Pts',(198.541659664048,88.4267388277125,336.794305791636));
#23910=CARTESIAN_POINT('Ctrl Pts',(199.281733177753,88.3839944866977,335.714843116983));
#23911=CARTESIAN_POINT('Ctrl Pts',(199.745420114066,88.3630770264696,335.258788929538));
#23912=CARTESIAN_POINT('Ctrl Pts',(200.836607730856,88.3232085762271,334.537042480549));
#23913=CARTESIAN_POINT('Ctrl Pts',(201.457803398381,88.3021966711763,334.284696586011));
#23914=CARTESIAN_POINT('Ctrl Pts',(202.743405108092,88.2594646574403,334.041028494398));
#23915=CARTESIAN_POINT('Ctrl Pts',(203.393957507691,88.2385307547311,334.044570031733));
#23916=CARTESIAN_POINT('Ctrl Pts',(204.676297004713,88.1986294812628,334.302146514328));
#23917=CARTESIAN_POINT('Ctrl Pts',(205.294264394291,88.1776856240901,334.560933524853));
#23918=CARTESIAN_POINT('Ctrl Pts',(206.37763782029,88.1349670086806,335.294148511304));
#23919=CARTESIAN_POINT('Ctrl Pts',(206.836690788396,88.1140157223278,335.755405346023));
#23920=CARTESIAN_POINT('Ctrl Pts',(207.564369000081,88.0740795693206,336.841827957796));
#23921=CARTESIAN_POINT('Ctrl Pts',(207.820087736203,88.0532071983605,337.460467803297));
#23922=CARTESIAN_POINT('Ctrl Pts',(208.071877720026,88.0105031403483,338.743830305215));
#23923=CARTESIAN_POINT('Ctrl Pts',(208.072436481244,87.9895335112199,339.394799672281));
#23924=CARTESIAN_POINT('Ctrl Pts',(207.938701912113,87.968107885949,340.082599871997));
#23925=CARTESIAN_POINT('Ctrl Pts',(207.927163070987,87.9664163810168,340.137065741634));
#23926=CARTESIAN_POINT('Ctrl Pts',(207.914727694784,87.9647376097703,340.191287620971));
#23927=CARTESIAN_POINT('',(207.914727694784,85.7397376070391,340.191287620971));
#23928=CARTESIAN_POINT('',(207.914727694784,100.739737607039,340.191287620971));
#23929=CARTESIAN_POINT('Origin',(203.041252647846,85.7397376070391,339.073593133701));
#23930=CARTESIAN_POINT('',(204.158947135117,87.2147376097703,334.200118086763));
#23931=CARTESIAN_POINT('Ctrl Pts',(207.914727694784,87.9647376097703,340.191287620971));
#23932=CARTESIAN_POINT('Ctrl Pts',(207.779340168193,87.946460343118,340.781616856755));
#23933=CARTESIAN_POINT('Ctrl Pts',(207.53769820905,87.9269437466332,341.342944322924));
#23934=CARTESIAN_POINT('Ctrl Pts',(206.843213031075,87.8860746366299,342.384380270813));
#23935=CARTESIAN_POINT('Ctrl Pts',(206.38474502582,87.8650856931962,342.846831028044));
#23936=CARTESIAN_POINT('Ctrl Pts',(205.303760064132,87.8250733241061,343.581239138041));
#23937=CARTESIAN_POINT('Ctrl Pts',(204.68802080038,87.8043541348048,343.840776520152));
#23938=CARTESIAN_POINT('Ctrl Pts',(203.407235979897,87.7616830481099,344.101770828163));
#23939=CARTESIAN_POINT('Ctrl Pts',(202.755823948159,87.74067381298,344.106991129162));
#23940=CARTESIAN_POINT('Ctrl Pts',(201.471656924595,87.7006199795155,343.866645597679));
#23941=CARTESIAN_POINT('Ctrl Pts',(200.852390116532,87.6799823415197,343.617372251638));
#23942=CARTESIAN_POINT('Ctrl Pts',(199.759636945518,87.6373298715157,342.900841860573));
#23943=CARTESIAN_POINT('Ctrl Pts',(199.293358206015,87.6162993689764,342.445561511859));
#23944=CARTESIAN_POINT('Ctrl Pts',(198.551355972455,87.5762017622807,341.370752937042));
#23945=CARTESIAN_POINT('Ctrl Pts',(198.287519423439,87.5556488164053,340.758287651802));
#23946=CARTESIAN_POINT('Ctrl Pts',(198.016152199308,87.5130165270529,339.480458695237));
#23947=CARTESIAN_POINT('Ctrl Pts',(198.005659980213,87.4919637916292,338.828586140853));
#23948=CARTESIAN_POINT('Ctrl Pts',(198.23566858912,87.451820062317,337.543373246385));
#23949=CARTESIAN_POINT('Ctrl Pts',(198.479269848345,87.4313547653813,336.923342329837));
#23950=CARTESIAN_POINT('Ctrl Pts',(199.185797327074,87.3887443333827,335.825055199215));
#23951=CARTESIAN_POINT('Ctrl Pts',(199.637451092009,87.3676684194138,335.354491635781));
#23952=CARTESIAN_POINT('Ctrl Pts',(200.705281337784,87.327476190036,334.6039724502));
#23953=CARTESIAN_POINT('Ctrl Pts',(201.314073893669,87.3071012622527,334.335326173143));
#23954=CARTESIAN_POINT('Ctrl Pts',(202.322427028207,87.2734064507242,334.111428557303));
#23955=CARTESIAN_POINT('Ctrl Pts',(202.695363361447,87.2611781225391,334.071578327997));
#23956=CARTESIAN_POINT('Ctrl Pts',(203.436005015253,87.2373458911319,334.075724784825));
#23957=CARTESIAN_POINT('Ctrl Pts',(203.801439960117,87.2258064397917,334.118126531495));
#23958=CARTESIAN_POINT('Ctrl Pts',(204.158947135117,87.2147376097703,334.200118086763));
#23959=CARTESIAN_POINT('',(204.158947135117,88.0897376070391,334.200118086763));
#23960=CARTESIAN_POINT('',(204.158947135117,87.6522376084047,334.200118086763));
#23961=CARTESIAN_POINT('Ctrl Pts',(204.158947135117,88.0897376070391,334.200118086763));
#23962=CARTESIAN_POINT('Ctrl Pts',(203.54376721609,88.108784279197,334.059031244714));
#23963=CARTESIAN_POINT('Ctrl Pts',(202.907424402043,88.1291528952381,334.035698514464));
#23964=CARTESIAN_POINT('Ctrl Pts',(201.658010954093,88.1704358529046,334.227232493023));
#23965=CARTESIAN_POINT('Ctrl Pts',(201.056254175817,88.1909801212834,334.44105583193));
#23966=CARTESIAN_POINT('Ctrl Pts',(199.95737379632,88.2298802575433,335.086005660858));
#23967=CARTESIAN_POINT('Ctrl Pts',(199.471903535416,88.2500471815186,335.513960251011));
#23968=CARTESIAN_POINT('Ctrl Pts',(198.673788261365,88.2927299786094,336.549836946009));
#23969=CARTESIAN_POINT('Ctrl Pts',(198.37666142415,88.3144309354573,337.153766384104));
#23970=CARTESIAN_POINT('Ctrl Pts',(198.043129582088,88.3543991722063,338.418037257362));
#23971=CARTESIAN_POINT('Ctrl Pts',(198.000324105281,88.3745056169959,339.063645207031));
#23972=CARTESIAN_POINT('Ctrl Pts',(198.164036244939,88.4171703698358,340.36065777686));
#23973=CARTESIAN_POINT('Ctrl Pts',(198.378711301086,88.4388754227734,340.998310722234));
#23974=CARTESIAN_POINT('Ctrl Pts',(199.03269180681,88.4788846944295,342.130102793843));
#23975=CARTESIAN_POINT('Ctrl Pts',(199.457114736403,88.4989280935846,342.618284039044));
#23976=CARTESIAN_POINT('Ctrl Pts',(200.486811363997,88.5415733489109,343.423106824859));
#23977=CARTESIAN_POINT('Ctrl Pts',(201.088166405913,88.5632824904017,343.724286290855));
#23978=CARTESIAN_POINT('Ctrl Pts',(202.349249899138,88.6033352439291,344.06676520106));
#23979=CARTESIAN_POINT('Ctrl Pts',(202.994240055269,88.6233131629387,344.114276293583));
#23980=CARTESIAN_POINT('Ctrl Pts',(204.291632762956,88.6659373688183,343.960272214956));
#23981=CARTESIAN_POINT('Ctrl Pts',(204.930381417393,88.6876505466125,343.750592929646));
#23982=CARTESIAN_POINT('Ctrl Pts',(206.066495555729,88.7277492840862,343.105759577051));
#23983=CARTESIAN_POINT('Ctrl Pts',(206.557754177849,88.7476594657781,342.68534264916));
#23984=CARTESIAN_POINT('Ctrl Pts',(207.370150628802,88.7902609688187,341.662675323108));
#23985=CARTESIAN_POINT('Ctrl Pts',(207.675900131243,88.8119780788274,341.064270729581));
#23986=CARTESIAN_POINT('Ctrl Pts',(207.877155278121,88.8348930549401,340.346560173747));
#23987=CARTESIAN_POINT('Ctrl Pts',(207.896880887269,88.8373282945415,340.269104924431));
#23988=CARTESIAN_POINT('Ctrl Pts',(207.914727694784,88.8397376070391,340.191287620971));
#23989=CARTESIAN_POINT('Origin',(203.041252647846,100.739737607039,339.073593133701));
#23990=CARTESIAN_POINT('',(207.91472769442,89.9647376096719,340.191287622561));
#23991=CARTESIAN_POINT('',(207.914727694784,89.8397376070391,340.191287620971));
#23992=CARTESIAN_POINT('',(207.914727694784,100.739737607039,340.191287620971));
#23993=CARTESIAN_POINT('Ctrl Pts',(207.914727694055,89.9647376096719,340.19128762415));
#23994=CARTESIAN_POINT('Ctrl Pts',(207.765836313037,89.9446373276548,340.840497615063));
#23995=CARTESIAN_POINT('Ctrl Pts',(207.488691142175,89.9230721417589,341.453535818966));
#23996=CARTESIAN_POINT('Ctrl Pts',(206.723968003099,89.8803105231624,342.516118973487));
#23997=CARTESIAN_POINT('Ctrl Pts',(206.25123333942,89.859527679405,342.960682232891));
#23998=CARTESIAN_POINT('Ctrl Pts',(205.142071735324,89.8199224731142,343.659758184998));
#23999=CARTESIAN_POINT('Ctrl Pts',(204.511116747618,89.7983389472792,343.899148565792));
#24000=CARTESIAN_POINT('Ctrl Pts',(203.217243112099,89.7555097258034,344.111698106939));
#24001=CARTESIAN_POINT('Ctrl Pts',(202.568513826031,89.7347193400774,344.092562469778));
#24002=CARTESIAN_POINT('Ctrl Pts',(201.289709194899,89.6950996203709,343.804145989652));
#24003=CARTESIAN_POINT('Ctrl Pts',(200.674156782173,89.6735487572462,343.528144091416));
#24004=CARTESIAN_POINT('Ctrl Pts',(199.608064700761,89.6307244318617,342.765042758847));
#24005=CARTESIAN_POINT('Ctrl Pts',(199.162199994239,89.6099259509072,342.293312188139));
#24006=CARTESIAN_POINT('Ctrl Pts',(198.460560629068,89.5702906244146,341.186164222411));
#24007=CARTESIAN_POINT('Ctrl Pts',(198.219699953616,89.5487747405038,340.556311920956));
#24008=CARTESIAN_POINT('Ctrl Pts',(198.003625675874,89.5059557392046,339.263350691311));
#24009=CARTESIAN_POINT('Ctrl Pts',(198.021004392555,89.4851485762116,338.614397131199));
#24010=CARTESIAN_POINT('Ctrl Pts',(198.305934471926,89.4454964780859,337.335175835121));
#24011=CARTESIAN_POINT('Ctrl Pts',(198.579978018731,89.4240180164272,336.719344213792));
#24012=CARTESIAN_POINT('Ctrl Pts',(199.339699623022,89.3812048051796,335.651266291293));
#24013=CARTESIAN_POINT('Ctrl Pts',(199.810260907171,89.360388338936,335.20389445849));
#24014=CARTESIAN_POINT('Ctrl Pts',(200.915070081928,89.3207182299794,334.499285318589));
#24015=CARTESIAN_POINT('Ctrl Pts',(201.543644603275,89.2992797606034,334.25672303268));
#24016=CARTESIAN_POINT('Ctrl Pts',(202.835541442451,89.256472846674,334.036567182181));
#24017=CARTESIAN_POINT('Ctrl Pts',(203.48474907395,89.2356464209134,334.051908390896));
#24018=CARTESIAN_POINT('Ctrl Pts',(204.764447665162,89.1959569849016,334.332799148957));
#24019=CARTESIAN_POINT('Ctrl Pts',(205.380600721626,89.174561203976,334.604577695675));
#24020=CARTESIAN_POINT('Ctrl Pts',(206.450969076925,89.1317611395162,335.36038385866));
#24021=CARTESIAN_POINT('Ctrl Pts',(206.900081924164,89.1109240625106,335.829585646961));
#24022=CARTESIAN_POINT('Ctrl Pts',(207.608123444597,89.0712139037832,336.931683747536));
#24023=CARTESIAN_POINT('Ctrl Pts',(207.852650079897,89.0498636311976,337.558781077251));
#24024=CARTESIAN_POINT('Ctrl Pts',(208.077520715676,89.0070710170895,338.849437926982));
#24025=CARTESIAN_POINT('Ctrl Pts',(208.064537138292,88.9862225615405,339.498931492889));
#24026=CARTESIAN_POINT('Ctrl Pts',(207.92423497449,88.9660411934147,340.149208900489));
#24027=CARTESIAN_POINT('Ctrl Pts',(207.919548623402,88.9653884333734,340.170266961399));
#24028=CARTESIAN_POINT('Ctrl Pts',(207.914727694784,88.9647376097703,340.191287620971));
#24029=CARTESIAN_POINT('Ctrl Pts',(207.914727694784,88.8397376070391,340.191287620971));
#24030=CARTESIAN_POINT('Ctrl Pts',(208.039783122405,88.8566200441031,339.646009360289));
#24031=CARTESIAN_POINT('Ctrl Pts',(208.072570540725,88.8745745972925,339.08302195561));
#24032=CARTESIAN_POINT('Ctrl Pts',(207.938295616732,88.9145428019993,337.864761677801));
#24033=CARTESIAN_POINT('Ctrl Pts',(207.734267589585,88.9362636808166,337.224819805819));
#24034=CARTESIAN_POINT('Ctrl Pts',(207.099781432225,88.9764620461028,336.083865485545));
#24035=CARTESIAN_POINT('Ctrl Pts',(206.683879353213,88.9962309428581,335.589135578386));
#24036=CARTESIAN_POINT('Ctrl Pts',(205.669157623561,89.0387816650799,334.768248217967));
#24037=CARTESIAN_POINT('Ctrl Pts',(205.07411610365,89.0605060822714,334.457383359739));
#24038=CARTESIAN_POINT('Ctrl Pts',(203.820831313731,89.1007581284528,334.093409377673));
#24039=CARTESIAN_POINT('Ctrl Pts',(203.177317914083,89.1204540948528,334.034595137357));
#24040=CARTESIAN_POINT('Ctrl Pts',(201.879157737075,89.1629765301353,334.165338091881));
#24041=CARTESIAN_POINT('Ctrl Pts',(201.23793384196,89.1847041804466,334.363017924715));
#24042=CARTESIAN_POINT('Ctrl Pts',(200.091603706288,89.2250124793616,334.985879532102));
#24043=CARTESIAN_POINT('Ctrl Pts',(199.592985793183,89.244634498187,335.396729857411));
#24044=CARTESIAN_POINT('Ctrl Pts',(198.762654773095,89.2871265777634,336.40253314374));
#24045=CARTESIAN_POINT('Ctrl Pts',(198.446111687749,89.3088570734383,336.993765169786));
#24046=CARTESIAN_POINT('Ctrl Pts',(198.06945739481,89.3492241660787,338.242354716365));
#24047=CARTESIAN_POINT('Ctrl Pts',(198.003974576252,89.3687716758309,338.885001849879));
#24048=CARTESIAN_POINT('Ctrl Pts',(198.121036203777,89.4112312310817,340.183519585841));
#24049=CARTESIAN_POINT('Ctrl Pts',(198.311640785712,89.4329640945147,340.826099870704));
#24050=CARTESIAN_POINT('Ctrl Pts',(198.921542813813,89.4733924677716,341.97834606647));
#24051=CARTESIAN_POINT('Ctrl Pts',(199.326785715225,89.4928654224372,342.481284614558));
#24052=CARTESIAN_POINT('Ctrl Pts',(200.322657070839,89.5352901897899,343.322026523897));
#24053=CARTESIAN_POINT('Ctrl Pts',(200.909604638288,89.5570248467713,343.644814478036));
#24054=CARTESIAN_POINT('Ctrl Pts',(202.152920910627,89.5975169085681,344.035486130514));
#24055=CARTESIAN_POINT('Ctrl Pts',(202.794614536233,89.6169158355446,344.108343155427));
#24056=CARTESIAN_POINT('Ctrl Pts',(204.093446611738,89.6593034633917,344.006370656474));
#24057=CARTESIAN_POINT('Ctrl Pts',(204.737436987694,89.6810392372306,343.823582864136));
#24058=CARTESIAN_POINT('Ctrl Pts',(205.896128026944,89.7215972903815,343.22800597391));
#24059=CARTESIAN_POINT('Ctrl Pts',(206.40382650992,89.740923344727,342.828932689881));
#24060=CARTESIAN_POINT('Ctrl Pts',(207.255934687688,89.7832714025403,341.844025663645));
#24061=CARTESIAN_POINT('Ctrl Pts',(207.585520870882,89.8050075093724,341.261857912909));
#24062=CARTESIAN_POINT('Ctrl Pts',(207.839739270826,89.8304444167043,340.487071034736));
#24063=CARTESIAN_POINT('Ctrl Pts',(207.880650046621,89.8351371369807,340.339876139457));
#24064=CARTESIAN_POINT('Ctrl Pts',(207.914727694784,89.8397376070391,340.191287620971));
#24065=CARTESIAN_POINT('Origin',(203.041252647846,100.739737607039,339.073593133701));
#24066=CARTESIAN_POINT('',(207.914727694784,90.9647376097703,340.191287620971));
#24067=CARTESIAN_POINT('',(207.914727694784,90.8397376070391,340.191287620971));
#24068=CARTESIAN_POINT('',(207.914727694784,100.739737607039,340.191287620971));
#24069=CARTESIAN_POINT('Ctrl Pts',(207.914727694784,90.9647376097703,340.191287620971));
#24070=CARTESIAN_POINT('Ctrl Pts',(207.911315614514,90.9642769801797,340.206165289461));
#24071=CARTESIAN_POINT('Ctrl Pts',(207.907834706666,90.9638153823686,340.221030386257));
#24072=CARTESIAN_POINT('Ctrl Pts',(207.748995822073,90.9431175509878,340.885614180962));
#24073=CARTESIAN_POINT('Ctrl Pts',(207.465064048657,90.9214503419892,341.497658974635));
#24074=CARTESIAN_POINT('Ctrl Pts',(206.688739812019,90.8786533272244,342.55332217813));
#24075=CARTESIAN_POINT('Ctrl Pts',(206.211987656894,90.858050405444,342.992649373643));
#24076=CARTESIAN_POINT('Ctrl Pts',(205.0964906552,90.8183824836142,343.680372545011));
#24077=CARTESIAN_POINT('Ctrl Pts',(204.463211692172,90.7967181428265,343.913467941326));
#24078=CARTESIAN_POINT('Ctrl Pts',(203.167915983234,90.7539132949477,344.113112254686));
#24079=CARTESIAN_POINT('Ctrl Pts',(202.520014328993,90.7332767213144,344.087672267514));
#24080=CARTESIAN_POINT('Ctrl Pts',(201.244282853357,90.6936279488897,343.787133415081));
#24081=CARTESIAN_POINT('Ctrl Pts',(200.631132545857,90.6719663189768,343.50505100369));
#24082=CARTESIAN_POINT('Ctrl Pts',(199.572735897812,90.6291542589892,342.731775884857));
#24083=CARTESIAN_POINT('Ctrl Pts',(199.131829275079,90.6084862284796,342.256233206372));
#24084=CARTESIAN_POINT('Ctrl Pts',(198.440557748886,90.5688552399164,341.142481984388));
#24085=CARTESIAN_POINT('Ctrl Pts',(198.205526680641,90.5471961660466,340.509693352836));
#24086=CARTESIAN_POINT('Ctrl Pts',(198.002092924037,90.5043774669823,339.21460737477));
#24087=CARTESIAN_POINT('Ctrl Pts',(198.025705648113,90.4836800703889,338.566463229518));
#24088=CARTESIAN_POINT('Ctrl Pts',(198.322776246166,90.444065584652,337.289553462054));
#24089=CARTESIAN_POINT('Ctrl Pts',(198.603268531205,90.4224089156099,336.675458761662));
#24090=CARTESIAN_POINT('Ctrl Pts',(199.373922787544,90.3795841059849,335.614719441325));
#24091=CARTESIAN_POINT('Ctrl Pts',(199.848427824991,90.3588593286175,335.172457490587));
#24092=CARTESIAN_POINT('Ctrl Pts',(200.960678185243,90.3192601458917,334.478145342542));
#24093=CARTESIAN_POINT('Ctrl Pts',(201.593042050042,90.2976057349498,334.241455871552));
#24094=CARTESIAN_POINT('Ctrl Pts',(202.887943831758,90.2547753020222,334.034773284165));
#24095=CARTESIAN_POINT('Ctrl Pts',(203.536295954121,90.234025023694,334.056819976455));
#24096=CARTESIAN_POINT('Ctrl Pts',(204.814211375342,90.1944400219056,334.350918809372));
#24097=CARTESIAN_POINT('Ctrl Pts',(205.429111504593,90.1727877274885,334.630047356649));
#24098=CARTESIAN_POINT('Ctrl Pts',(206.49179462128,90.1299545299613,335.398411252325));
#24099=CARTESIAN_POINT('Ctrl Pts',(206.935236426321,90.1091852393959,335.872006985988));
#24100=CARTESIAN_POINT('Ctrl Pts',(207.632104259007,90.0696060505826,336.982899331542));
#24101=CARTESIAN_POINT('Ctrl Pts',(207.870226988821,90.0479636513252,337.614803975402));
#24102=CARTESIAN_POINT('Ctrl Pts',(208.079739104538,90.005125784942,338.909458833918));
#24103=CARTESIAN_POINT('Ctrl Pts',(208.059091403677,89.9843499624347,339.557991247767));
#24104=CARTESIAN_POINT('Ctrl Pts',(207.915713008852,89.9648708373616,340.186984826092));
#24105=CARTESIAN_POINT('Ctrl Pts',(207.915221055665,89.9648042133088,340.189136423161));
#24106=CARTESIAN_POINT('Ctrl Pts',(207.914727694055,89.9647376096719,340.19128762415));
#24107=CARTESIAN_POINT('Ctrl Pts',(207.914727694784,89.8397376070391,340.191287620971));
#24108=CARTESIAN_POINT('Ctrl Pts',(208.023215162931,89.854383375624,339.718250512049));
#24109=CARTESIAN_POINT('Ctrl Pts',(208.062435766932,89.8698590586585,339.231140777883));
#24110=CARTESIAN_POINT('Ctrl Pts',(207.986989240129,89.9071947273622,338.084683157661));
#24111=CARTESIAN_POINT('Ctrl Pts',(207.812754309931,89.9289302729595,337.439255866093));
#24112=CARTESIAN_POINT('Ctrl Pts',(207.232863968651,89.969626661502,336.273621397437));
#24113=CARTESIAN_POINT('Ctrl Pts',(206.84051399295,89.9888131813776,335.7607285162));
#24114=CARTESIAN_POINT('Ctrl Pts',(205.867595136952,90.0310745515505,334.896341406658));
#24115=CARTESIAN_POINT('Ctrl Pts',(205.290711644538,90.0528085299448,334.559436652983));
#24116=CARTESIAN_POINT('Ctrl Pts',(204.059760957976,90.093576916516,334.136778324456));
#24117=CARTESIAN_POINT('Ctrl Pts',(203.420228210987,90.1126982392496,334.047074883442));
#24118=CARTESIAN_POINT('Ctrl Pts',(202.120991259532,90.1549124009898,334.114749265968));
#24119=CARTESIAN_POINT('Ctrl Pts',(201.474132624673,90.1766436952053,334.279724492657));
#24120=CARTESIAN_POINT('Ctrl Pts',(200.301106772013,90.217485691699,334.842612445414));
#24121=CARTESIAN_POINT('Ctrl Pts',(199.782603329716,90.2365458797191,335.227711231833));
#24122=CARTESIAN_POINT('Ctrl Pts',(198.905101251835,90.278710225717,336.187659101803));
#24123=CARTESIAN_POINT('Ctrl Pts',(198.560411951696,90.3004376108674,336.758759251106));
#24124=CARTESIAN_POINT('Ctrl Pts',(198.119921305086,90.3413545916701,337.982611312581));
#24125=CARTESIAN_POINT('Ctrl Pts',(198.02080853357,90.3603584786334,338.620947320342));
#24126=CARTESIAN_POINT('Ctrl Pts',(198.069441093885,90.4024704041232,339.920224927786));
#24127=CARTESIAN_POINT('Ctrl Pts',(198.224505503012,90.4241925530731,340.568472890227));
#24128=CARTESIAN_POINT('Ctrl Pts',(198.769167220228,90.4651856326072,341.749266742395));
#24129=CARTESIAN_POINT('Ctrl Pts',(199.146531472698,90.4841388126341,342.27376378772));
#24130=CARTESIAN_POINT('Ctrl Pts',(200.092602516096,90.5261957384747,343.165105483259));
#24131=CARTESIAN_POINT('Ctrl Pts',(200.6574427396,90.5479112301913,343.517969530997));
#24132=CARTESIAN_POINT('Ctrl Pts',(201.873612083517,90.5889812433873,343.977348334716));
#24133=CARTESIAN_POINT('Ctrl Pts',(202.510685454206,90.6078900436021,344.086446491198));
#24134=CARTESIAN_POINT('Ctrl Pts',(203.809864421873,90.6498894410831,344.057923331698));
#24135=CARTESIAN_POINT('Ctrl Pts',(204.459421447231,90.6715967717128,343.913337592328));
#24136=CARTESIAN_POINT('Ctrl Pts',(205.648269371093,90.7127442580518,343.387985290973));
#24137=CARTESIAN_POINT('Ctrl Pts',(206.17909464918,90.7316156938061,343.018775424987));
#24138=CARTESIAN_POINT('Ctrl Pts',(207.084856353885,90.7735551107592,342.087372923418));
#24139=CARTESIAN_POINT('Ctrl Pts',(207.446189989066,90.7952527073595,341.529227748421));
#24140=CARTESIAN_POINT('Ctrl Pts',(207.782744424956,90.8242100641158,340.680741423644));
#24141=CARTESIAN_POINT('Ctrl Pts',(207.85812863934,90.8320967552217,340.438076065871));
#24142=CARTESIAN_POINT('Ctrl Pts',(207.914727694784,90.8397376070391,340.191287620971));
#24143=CARTESIAN_POINT('Origin',(203.041252647846,100.739737607039,339.073593133701));
#24144=CARTESIAN_POINT('',(207.914727694784,91.9647376097702,340.191287620971));
#24145=CARTESIAN_POINT('',(207.914727694784,91.8397376070391,340.191287620971));
#24146=CARTESIAN_POINT('',(207.914727694784,100.739737607039,340.191287620971));
#24147=CARTESIAN_POINT('Ctrl Pts',(207.914727694784,91.9647376097703,340.191287620971));
#24148=CARTESIAN_POINT('Ctrl Pts',(207.904254565996,91.9633237412082,340.236953527346));
#24149=CARTESIAN_POINT('Ctrl Pts',(207.893133690911,91.9619008454671,340.282497930865));
#24150=CARTESIAN_POINT('Ctrl Pts',(207.714105944956,91.940122244649,340.973325472129));
#24151=CARTESIAN_POINT('Ctrl Pts',(207.419431766777,91.9184267450767,341.57879400991));
#24152=CARTESIAN_POINT('Ctrl Pts',(206.625372232688,91.8757217952659,342.61838696805));
#24153=CARTESIAN_POINT('Ctrl Pts',(206.141534760899,91.8554776998392,343.048469769076));
#24154=CARTESIAN_POINT('Ctrl Pts',(205.015891675147,91.815596502115,343.715318372967));
#24155=CARTESIAN_POINT('Ctrl Pts',(204.379845146041,91.7939049779004,343.937020373372));
#24156=CARTESIAN_POINT('Ctrl Pts',(203.083428523973,91.7511850254589,344.114413409457));
#24157=CARTESIAN_POINT('Ctrl Pts',(202.436948534698,91.730886764099,344.078228661387));
#24158=CARTESIAN_POINT('Ctrl Pts',(201.168252151569,91.6910389414042,343.757281372481));
#24159=CARTESIAN_POINT('Ctrl Pts',(200.560755003687,91.6693512961696,343.46587485997));
#24160=CARTESIAN_POINT('Ctrl Pts',(199.516238464375,91.6266174911885,342.677214788824));
#24161=CARTESIAN_POINT('Ctrl Pts',(199.083330651644,91.6062677997654,342.195543722738));
#24162=CARTESIAN_POINT('Ctrl Pts',(198.410083905223,91.5664512462118,341.072987920166));
#24163=CARTESIAN_POINT('Ctrl Pts',(198.184888851631,91.5447673641103,340.43776840419));
#24164=CARTESIAN_POINT('Ctrl Pts',(198.000683309217,91.5020207752774,339.141674950375));
#24165=CARTESIAN_POINT('Ctrl Pts',(198.033575491245,91.4816223761694,338.494760123088));
#24166=CARTESIAN_POINT('Ctrl Pts',(198.348266638407,91.4418350779639,337.223888606625));
#24167=CARTESIAN_POINT('Ctrl Pts',(198.636820966877,91.4201548280399,336.614641057529));
#24168=CARTESIAN_POINT('Ctrl Pts',(199.420771582785,91.3773964471176,335.565852361434));
#24169=CARTESIAN_POINT('Ctrl Pts',(199.900559811442,91.3569520271025,335.130488175659));
#24170=CARTESIAN_POINT('Ctrl Pts',(201.020421611829,91.3171920645888,334.451691747877));
#24171=CARTESIAN_POINT('Ctrl Pts',(201.654908567266,91.295515304612,334.223467461566));
#24172=CARTESIAN_POINT('Ctrl Pts',(202.950707148227,91.2527460509195,334.03334736297));
#24173=CARTESIAN_POINT('Ctrl Pts',(203.597999806697,91.2322582427972,334.063383117562));
#24174=CARTESIAN_POINT('Ctrl Pts',(204.870744491466,91.192523791354,334.372648356914));
#24175=CARTESIAN_POINT('Ctrl Pts',(205.481497664974,91.1708503711545,334.658724598177));
#24176=CARTESIAN_POINT('Ctrl Pts',(206.533979223132,91.1280710959943,335.438585899667));
#24177=CARTESIAN_POINT('Ctrl Pts',(206.971470652013,91.1075424636214,335.916744200083));
#24178=CARTESIAN_POINT('Ctrl Pts',(207.655062876658,91.0678317935738,337.034265884231));
#24179=CARTESIAN_POINT('Ctrl Pts',(207.88590435845,91.0461615579108,337.668108405244));
#24180=CARTESIAN_POINT('Ctrl Pts',(208.078863787454,91.003871830217,338.948539322099));
#24181=CARTESIAN_POINT('Ctrl Pts',(208.054814952644,90.9836493384277,339.580466181525));
#24182=CARTESIAN_POINT('Ctrl Pts',(207.914727694784,90.9647376097703,340.191287620971));
#24183=CARTESIAN_POINT('Ctrl Pts',(207.914727694784,90.8397376070391,340.191287620971));
#24184=CARTESIAN_POINT('Ctrl Pts',(208.00079559222,90.8513567417646,339.816006401218));
#24185=CARTESIAN_POINT('Ctrl Pts',(208.04341648959,90.8635181561768,339.431223786886));
#24186=CARTESIAN_POINT('Ctrl Pts',(208.037342853879,90.8971966995547,338.386599953585));
#24187=CARTESIAN_POINT('Ctrl Pts',(207.903693993538,90.9188829362989,337.73585134799));
#24188=CARTESIAN_POINT('Ctrl Pts',(207.398546275849,90.9601857510994,336.538769603378));
#24189=CARTESIAN_POINT('Ctrl Pts',(207.037829385965,90.9790059298629,336.001344521028));
#24190=CARTESIAN_POINT('Ctrl Pts',(206.121737554768,91.0208184701916,335.080754684404));
#24191=CARTESIAN_POINT('Ctrl Pts',(205.570661670986,91.042491686754,334.710767762962));
#24192=CARTESIAN_POINT('Ctrl Pts',(204.37140152303,91.0838717256542,334.211232479903));
#24193=CARTESIAN_POINT('Ctrl Pts',(203.737001858586,91.1026790128869,334.080820427013));
#24194=CARTESIAN_POINT('Ctrl Pts',(202.438507526252,91.1444249449932,334.066786989316));
#24195=CARTESIAN_POINT('Ctrl Pts',(201.786717910239,91.1660834667067,334.1891731859));
#24196=CARTESIAN_POINT('Ctrl Pts',(200.581339502808,91.2075400168075,334.673451125967));
#24197=CARTESIAN_POINT('Ctrl Pts',(200.037118864543,91.2263434015514,335.025432819567));
#24198=CARTESIAN_POINT('Ctrl Pts',(199.101485417345,91.2680208475195,335.925752043778));
#24199=CARTESIAN_POINT('Ctrl Pts',(198.722782861348,91.2896630068129,336.469463462791));
#24200=CARTESIAN_POINT('Ctrl Pts',(198.20246699672,91.3311950492952,337.659656524762));
#24201=CARTESIAN_POINT('Ctrl Pts',(198.060968683261,91.3500037497455,338.292674017094));
#24202=CARTESIAN_POINT('Ctrl Pts',(198.025012185414,91.3916110384711,339.590565086089));
#24203=CARTESIAN_POINT('Ctrl Pts',(198.135959196406,91.4132351970082,340.243219103971));
#24204=CARTESIAN_POINT('Ctrl Pts',(198.59896480335,91.4548414274877,341.456836241764));
#24205=CARTESIAN_POINT('Ctrl Pts',(198.94207630356,91.473664751609,342.007962310047));
#24206=CARTESIAN_POINT('Ctrl Pts',(199.826364104401,91.515200448587,342.95865178267));
#24207=CARTESIAN_POINT('Ctrl Pts',(200.362510056219,91.5368050177093,343.346007517477));
#24208=CARTESIAN_POINT('Ctrl Pts',(201.543367467538,91.5784838632738,343.887206904971));
#24209=CARTESIAN_POINT('Ctrl Pts',(202.174991719712,91.59733108359,344.039892574598));
#24210=CARTESIAN_POINT('Ctrl Pts',(203.472109271237,91.6387940062626,344.097816099371));
#24211=CARTESIAN_POINT('Ctrl Pts',(204.125434244662,91.6603774719498,343.998326498988));
#24212=CARTESIAN_POINT('Ctrl Pts',(205.347115042016,91.7021270925556,343.556713039399));
#24213=CARTESIAN_POINT('Ctrl Pts',(205.90516388146,91.7210073554214,343.222494051428));
#24214=CARTESIAN_POINT('Ctrl Pts',(206.870719457898,91.7623965702574,342.354280424769));
#24215=CARTESIAN_POINT('Ctrl Pts',(207.266544924304,91.7839575123391,341.825796270456));
#24216=CARTESIAN_POINT('Ctrl Pts',(207.709836503838,91.8169485008814,340.901684117415));
#24217=CARTESIAN_POINT('Ctrl Pts',(207.832182807031,91.8285940773342,340.551207487534));
#24218=CARTESIAN_POINT('Ctrl Pts',(207.914727694784,91.8397376070391,340.191287620971));
#24219=CARTESIAN_POINT('Origin',(203.041252647846,100.739737607039,339.073593133701));
#24220=CARTESIAN_POINT('',(207.914727694784,92.9647376097703,340.191287620971));
#24221=CARTESIAN_POINT('',(207.914727694784,92.8397376070391,340.191287620971));
#24222=CARTESIAN_POINT('',(207.914727694784,100.739737607039,340.191287620971));
#24223=CARTESIAN_POINT('Ctrl Pts',(207.914727694784,92.9647376097703,340.191287620971));
#24224=CARTESIAN_POINT('Ctrl Pts',(207.892227982976,92.9617001568921,340.289392948778));
#24225=CARTESIAN_POINT('Ctrl Pts',(207.866744237917,92.9586217814126,340.386913603745));
#24226=CARTESIAN_POINT('Ctrl Pts',(207.650868691199,92.9349863231015,341.121293124528));
#24227=CARTESIAN_POINT('Ctrl Pts',(207.338208134411,92.9132597503841,341.715138681599));
#24228=CARTESIAN_POINT('Ctrl Pts',(206.514336473059,92.8707273127763,342.727051367469));
#24229=CARTESIAN_POINT('Ctrl Pts',(206.018381055642,92.8510060114433,343.141360532428));
#24230=CARTESIAN_POINT('Ctrl Pts',(204.875727022238,92.8107728045649,343.772186534325));
#24231=CARTESIAN_POINT('Ctrl Pts',(204.235374813868,92.7890495793809,343.974215619768));
#24232=CARTESIAN_POINT('Ctrl Pts',(202.93746924036,92.7464895458046,344.113380838905));
#24233=CARTESIAN_POINT('Ctrl Pts',(202.293421719787,92.7266957605897,344.058664024676));
#24234=CARTESIAN_POINT('Ctrl Pts',(201.03728664979,92.6865153427722,343.702482201109));
#24235=CARTESIAN_POINT('Ctrl Pts',(200.43993545088,92.6647957436461,343.395119864489));
#24236=CARTESIAN_POINT('Ctrl Pts',(199.41976437803,92.6222100439426,342.580047896261));
#24237=CARTESIAN_POINT('Ctrl Pts',(199.000767362234,92.6023453107654,342.087697910815));
#24238=CARTESIAN_POINT('Ctrl Pts',(198.359183863117,92.5622151020548,340.950057974279));
#24239=CARTESIAN_POINT('Ctrl Pts',(198.151279548677,92.540499335381,340.310929267508));
#24240=CARTESIAN_POINT('Ctrl Pts',(198.000721208541,92.4978897947837,339.013410133542));
#24241=CARTESIAN_POINT('Ctrl Pts',(198.049904086809,92.4779559666251,338.368639047898));
#24242=CARTESIAN_POINT('Ctrl Pts',(198.395562021898,92.4378734031648,337.108696346758));
#24243=CARTESIAN_POINT('Ctrl Pts',(198.69817850748,92.4161616109913,336.508263606751));
#24244=CARTESIAN_POINT('Ctrl Pts',(199.505381623403,92.3735299504441,335.48077035533));
#24245=CARTESIAN_POINT('Ctrl Pts',(199.994528170868,92.3535291417961,335.057604361251));
#24246=CARTESIAN_POINT('Ctrl Pts',(201.127679077017,92.3134916923056,334.406490428141));
#24247=CARTESIAN_POINT('Ctrl Pts',(201.765679529091,92.2917839599802,334.193380929935));
#24248=CARTESIAN_POINT('Ctrl Pts',(203.062815096665,92.2491317975486,334.032712656847));
#24249=CARTESIAN_POINT('Ctrl Pts',(203.708229251426,92.2290663322601,334.076992835882));
#24250=CARTESIAN_POINT('Ctrl Pts',(204.97150497861,92.1890715123517,334.413328425462));
#24251=CARTESIAN_POINT('Ctrl Pts',(205.574631065039,92.1673678758902,334.711726536329));
#24252=CARTESIAN_POINT('Ctrl Pts',(206.608574463218,92.1246967290659,335.511945063808));
#24253=CARTESIAN_POINT('Ctrl Pts',(207.03542325672,92.1045690921455,335.998263962301));
#24254=CARTESIAN_POINT('Ctrl Pts',(207.694927150099,92.0646144765212,337.12742654897));
#24255=CARTESIAN_POINT('Ctrl Pts',(207.912618599103,92.0429149295889,337.764399278767));
#24256=CARTESIAN_POINT('Ctrl Pts',(208.076116420636,92.0017575456216,339.014647340122));
#24257=CARTESIAN_POINT('Ctrl Pts',(208.047426427959,91.9826518902931,339.612682311334));
#24258=CARTESIAN_POINT('Ctrl Pts',(207.914727694784,91.9647376097703,340.191287620971));
#24259=CARTESIAN_POINT('Ctrl Pts',(207.914727694784,91.8397376070391,340.191287620971));
#24260=CARTESIAN_POINT('Ctrl Pts',(207.975755026631,91.8479762745539,339.925190595062));
#24261=CARTESIAN_POINT('Ctrl Pts',(208.015023379492,91.8564989753866,339.65394854609));
#24262=CARTESIAN_POINT('Ctrl Pts',(208.071915560571,91.8860128619997,338.727998026453));
#24263=CARTESIAN_POINT('Ctrl Pts',(207.98374299771,91.9075499725715,338.074201598698));
#24264=CARTESIAN_POINT('Ctrl Pts',(207.563354323306,91.9494347389235,336.844741368962));
#24265=CARTESIAN_POINT('Ctrl Pts',(207.237935160857,91.9684073028415,336.279842850259));
#24266=CARTESIAN_POINT('Ctrl Pts',(206.385622568559,92.009647402592,335.299803740156));
#24267=CARTESIAN_POINT('Ctrl Pts',(205.864787174727,92.0311595024063,334.8958023824));
#24268=CARTESIAN_POINT('Ctrl Pts',(204.702911587947,92.0731082695322,334.31365047058));
#24269=CARTESIAN_POINT('Ctrl Pts',(204.074041625411,92.0921391997607,334.138867997609));
#24270=CARTESIAN_POINT('Ctrl Pts',(202.778922520765,92.133304456027,334.038041146075));
#24271=CARTESIAN_POINT('Ctrl Pts',(202.124849705415,92.1547905081741,334.115187128895));
#24272=CARTESIAN_POINT('Ctrl Pts',(200.88798696223,92.1968006991891,334.514795833626));
#24273=CARTESIAN_POINT('Ctrl Pts',(200.31640011974,92.2158973817219,334.831616638204));
#24274=CARTESIAN_POINT('Ctrl Pts',(199.322431386889,92.2569879799097,335.668407568756));
#24275=CARTESIAN_POINT('Ctrl Pts',(198.910642365424,92.2784471004846,336.181714864627));
#24276=CARTESIAN_POINT('Ctrl Pts',(198.308941897931,92.3205160311824,337.334203367042));
#24277=CARTESIAN_POINT('Ctrl Pts',(198.123526783317,92.3396851833687,337.96174198073));
#24278=CARTESIAN_POINT('Ctrl Pts',(198.002294507203,92.3807015847452,339.255684549381));
#24279=CARTESIAN_POINT('Ctrl Pts',(198.068838247974,92.4021330503188,339.909852568494));
#24280=CARTESIAN_POINT('Ctrl Pts',(198.448365079681,92.4442579602656,341.15366757279));
#24281=CARTESIAN_POINT('Ctrl Pts',(198.756887665259,92.4635055704234,341.731701476214));
#24282=CARTESIAN_POINT('Ctrl Pts',(199.578721882776,92.5044485024553,342.738902330108));
#24283=CARTESIAN_POINT('Ctrl Pts',(200.084721682248,92.5258517542947,343.158016148845));
#24284=CARTESIAN_POINT('Ctrl Pts',(201.228058569042,92.5680298368164,343.778352321079));
#24285=CARTESIAN_POINT('Ctrl Pts',(201.85431352362,92.5873611212353,343.973960747681));
#24286=CARTESIAN_POINT('Ctrl Pts',(203.147001786061,92.628231564393,344.114605122069));
#24287=CARTESIAN_POINT('Ctrl Pts',(203.801105129643,92.6496062094924,344.058127463367));
#24288=CARTESIAN_POINT('Ctrl Pts',(205.051370084647,92.6918346399555,343.697766670287));
#24289=CARTESIAN_POINT('Ctrl Pts',(205.635541779686,92.711254017264,343.397157636541));
#24290=CARTESIAN_POINT('Ctrl Pts',(206.655165884056,92.7520531887422,342.589558218914));
#24291=CARTESIAN_POINT('Ctrl Pts',(207.081088435159,92.7733989978353,342.090558066796));
#24292=CARTESIAN_POINT('Ctrl Pts',(207.634658915025,92.8100866730409,341.105996354396));
#24293=CARTESIAN_POINT('Ctrl Pts',(207.807904347327,92.8253164941396,340.657068676701));
#24294=CARTESIAN_POINT('Ctrl Pts',(207.914727694784,92.8397376070391,340.191287620971));
#24295=CARTESIAN_POINT('Origin',(203.041252647846,100.739737607039,339.073593133701));
#24296=CARTESIAN_POINT('',(207.914727694784,93.9647376097703,340.191287620971));
#24297=CARTESIAN_POINT('',(207.914727694784,93.8397376070391,340.191287620971));
#24298=CARTESIAN_POINT('',(207.914727694784,100.739737607039,340.191287620971));
#24299=CARTESIAN_POINT('Ctrl Pts',(207.914727694784,93.9647376097703,340.191287620971));
#24300=CARTESIAN_POINT('Ctrl Pts',(207.873804939263,93.9592130527181,340.369722810693));
#24301=CARTESIAN_POINT('Ctrl Pts',(207.823038515332,93.9535568412456,340.546103814389));
#24302=CARTESIAN_POINT('Ctrl Pts',(207.544859034738,93.9270509333428,341.344009870334));
#24303=CARTESIAN_POINT('Ctrl Pts',(207.205454880507,93.9053185785856,341.9190550229));
#24304=CARTESIAN_POINT('Ctrl Pts',(206.336863308448,93.8630878112972,342.887834418589));
#24305=CARTESIAN_POINT('Ctrl Pts',(205.822178923424,93.8439443821288,343.277867828257));
#24306=CARTESIAN_POINT('Ctrl Pts',(204.654171934117,93.8032010656026,343.85233561752));
#24307=CARTESIAN_POINT('Ctrl Pts',(204.008273922891,93.78146642501,344.023616034488));
#24308=CARTESIAN_POINT('Ctrl Pts',(202.709131222029,93.7391893468591,344.103418851654));
#24309=CARTESIAN_POINT('Ctrl Pts',(202.0688352615,93.7199794957506,344.019686859139));
#24310=CARTESIAN_POINT('Ctrl Pts',(200.833450820258,93.679307569546,343.608359267027));
#24311=CARTESIAN_POINT('Ctrl Pts',(200.25295671188,93.6575717219641,343.276433212799));
#24312=CARTESIAN_POINT('Ctrl Pts',(199.271861312971,93.6152509109054,342.420404293397));
#24313=CARTESIAN_POINT('Ctrl Pts',(198.874928115931,93.5959716030076,341.911053208444));
#24314=CARTESIAN_POINT('Ctrl Pts',(198.284335982435,93.5553691749377,340.750142830051));
#24315=CARTESIAN_POINT('Ctrl Pts',(198.104266929115,93.5336330876967,340.105683711802));
#24316=CARTESIAN_POINT('Ctrl Pts',(198.00753666247,93.4912710785197,338.806761983362));
#24317=CARTESIAN_POINT('Ctrl Pts',(198.08296068611,93.4719200173456,338.165399182987));
#24318=CARTESIAN_POINT('Ctrl Pts',(198.478510104806,93.4313850179656,336.92393853915));
#24319=CARTESIAN_POINT('Ctrl Pts',(198.803462998129,93.4096495469072,336.338499897794));
#24320=CARTESIAN_POINT('Ctrl Pts',(199.64782067779,93.3672488157421,335.346102693374));
#24321=CARTESIAN_POINT('Ctrl Pts',(200.152268500491,93.3478244087075,334.942816948992));
#24322=CARTESIAN_POINT('Ctrl Pts',(201.306566580844,93.3073546185777,334.337451817897));
#24323=CARTESIAN_POINT('Ctrl Pts',(201.949603581291,93.2856205100925,334.149323412115));
#24324=CARTESIAN_POINT('Ctrl Pts',(203.248230013819,93.2431834613731,334.037044497523));
#24325=CARTESIAN_POINT('Ctrl Pts',(203.890574709682,93.2236847761094,334.104862394107));
#24326=CARTESIAN_POINT('Ctrl Pts',(205.137503667319,93.18327785308,334.485956033074));
#24327=CARTESIAN_POINT('Ctrl Pts',(205.727387109702,93.1615457478529,334.804480598285));
#24328=CARTESIAN_POINT('Ctrl Pts',(206.73005323215,93.1190747036848,335.638112022245));
#24329=CARTESIAN_POINT('Ctrl Pts',(207.139130334014,93.0995014172781,336.138095670888));
#24330=CARTESIAN_POINT('Ctrl Pts',(207.757900090983,93.059154923242,337.28630252403));
#24331=CARTESIAN_POINT('Ctrl Pts',(207.95334570219,93.037425361389,337.927962978038));
#24332=CARTESIAN_POINT('Ctrl Pts',(208.069986967232,92.998210224646,339.125819186543));
#24333=CARTESIAN_POINT('Ctrl Pts',(208.034997750192,92.980974023333,339.666874983528));
#24334=CARTESIAN_POINT('Ctrl Pts',(207.914727694784,92.9647376097703,340.191287620971));
#24335=CARTESIAN_POINT('Ctrl Pts',(207.914727694784,92.8397376070391,340.191287620971));
#24336=CARTESIAN_POINT('Ctrl Pts',(207.953046404109,92.8449106188056,340.024206834718));
#24337=CARTESIAN_POINT('Ctrl Pts',(207.982817119989,92.8501997477775,339.854964028943));
#24338=CARTESIAN_POINT('Ctrl Pts',(208.08314124294,92.8759153768596,339.039608838099));
#24339=CARTESIAN_POINT('Ctrl Pts',(208.036107293269,92.8972322796717,338.385703867311));
#24340=CARTESIAN_POINT('Ctrl Pts',(207.693822250953,92.9395529881538,337.129522094079));
#24341=CARTESIAN_POINT('Ctrl Pts',(207.400674455767,92.9591585874978,336.539575623612));
#24342=CARTESIAN_POINT('Ctrl Pts',(206.606464645449,92.9998197178356,335.508414682625));
#24343=CARTESIAN_POINT('Ctrl Pts',(206.114085262997,93.0211077959075,335.076231426297));
#24344=CARTESIAN_POINT('Ctrl Pts',(204.987923137303,93.0634705184885,334.421989120271));
#24345=CARTESIAN_POINT('Ctrl Pts',(204.364051254315,93.0831726677721,334.207677672862));
#24346=CARTESIAN_POINT('Ctrl Pts',(203.073975604662,93.1237674003411,334.031805317889));
#24347=CARTESIAN_POINT('Ctrl Pts',(202.420374276277,93.145026877801,334.070077356855));
#24348=CARTESIAN_POINT('Ctrl Pts',(201.158820074663,93.187428952141,334.395504361998));
#24349=CARTESIAN_POINT('Ctrl Pts',(200.563500273469,93.2072289376568,334.681692667663));
#24350=CARTESIAN_POINT('Ctrl Pts',(199.521733604888,93.2477592306827,335.463445609985));
#24351=CARTESIAN_POINT('Ctrl Pts',(199.083850134906,93.2689904633737,335.949636063369));
#24352=CARTESIAN_POINT('Ctrl Pts',(198.41453404593,93.3114293120859,337.067938843608));
#24353=CARTESIAN_POINT('Ctrl Pts',(198.191837186309,93.3313277163342,337.690726855008));
#24354=CARTESIAN_POINT('Ctrl Pts',(198.000336637975,93.3717956559147,338.979504392752));
#24355=CARTESIAN_POINT('Ctrl Pts',(198.030562126869,93.392999119289,339.632725119442));
#24356=CARTESIAN_POINT('Ctrl Pts',(198.340429254254,93.4354722618472,340.899112857338));
#24357=CARTESIAN_POINT('Ctrl Pts',(198.620191065518,93.455469014206,341.499381269254));
#24358=CARTESIAN_POINT('Ctrl Pts',(199.390472404057,93.4958767908359,342.550807705861));
#24359=CARTESIAN_POINT('Ctrl Pts',(199.870940433053,93.517053067019,342.993835149602));
#24360=CARTESIAN_POINT('Ctrl Pts',(200.981943010181,93.5595581289031,343.676915049404));
#24361=CARTESIAN_POINT('Ctrl Pts',(201.603725719806,93.5796525620978,343.907309212695));
#24362=CARTESIAN_POINT('Ctrl Pts',(202.89124454375,93.6200024477401,344.113064218841));
#24363=CARTESIAN_POINT('Ctrl Pts',(203.544034043296,93.641152212143,344.090159679816));
#24364=CARTESIAN_POINT('Ctrl Pts',(204.814735265088,93.6836869314197,343.794517611611));
#24365=CARTESIAN_POINT('Ctrl Pts',(205.41951827782,93.7038778417882,343.5206350808));
#24366=CARTESIAN_POINT('Ctrl Pts',(206.479669165915,93.7441721678624,342.760819666309));
#24367=CARTESIAN_POINT('Ctrl Pts',(206.927301992097,93.7652961756821,342.285590081629));
#24368=CARTESIAN_POINT('Ctrl Pts',(207.572078650103,93.804752097779,341.261893830787));
#24369=CARTESIAN_POINT('Ctrl Pts',(207.789164667609,93.8227866442205,340.738779164257));
#24370=CARTESIAN_POINT('Ctrl Pts',(207.914727694784,93.8397376070391,340.191287620971));
#24371=CARTESIAN_POINT('Origin',(203.041252647846,100.739737607039,339.073593133701));
#24372=CARTESIAN_POINT('',(207.914727694784,94.9647376097703,340.191287620971));
#24373=CARTESIAN_POINT('',(207.914727694784,94.8397376070391,340.191287620971));
#24374=CARTESIAN_POINT('',(207.914727694784,100.739737607039,340.191287620971));
#24375=CARTESIAN_POINT('Ctrl Pts',(207.914727694784,94.9647376097703,340.191287620971));
#24376=CARTESIAN_POINT('Ctrl Pts',(207.849665529396,94.9559542412007,340.474977701877));
#24377=CARTESIAN_POINT('Ctrl Pts',(207.759811904417,94.9468502670507,340.753082234696));
#24378=CARTESIAN_POINT('Ctrl Pts',(207.389785636598,94.9165716596823,341.627400591467));
#24379=CARTESIAN_POINT('Ctrl Pts',(207.016947381176,94.894907871297,342.17609468672));
#24380=CARTESIAN_POINT('Ctrl Pts',(206.091448578882,94.8531387028617,343.087066397982));
#24381=CARTESIAN_POINT('Ctrl Pts',(205.551817251161,94.8343279625663,343.444946375562));
#24382=CARTESIAN_POINT('Ctrl Pts',(204.352021531765,94.7929745410165,343.943325616105));
#24383=CARTESIAN_POINT('Ctrl Pts',(203.700914252711,94.7712966367118,344.07331772725));
#24384=CARTESIAN_POINT('Ctrl Pts',(202.40211293344,94.7294615526946,344.07386083302));
#24385=CARTESIAN_POINT('Ctrl Pts',(201.766796617286,94.7106348898926,343.950778730699));
#24386=CARTESIAN_POINT('Ctrl Pts',(200.561643350943,94.6693588660483,343.46502551495));
#24387=CARTESIAN_POINT('Ctrl Pts',(200.005773851085,94.6476685179065,343.100874619319));
#24388=CARTESIAN_POINT('Ctrl Pts',(199.079319175464,94.6057696364642,342.19029639937));
#24389=CARTESIAN_POINT('Ctrl Pts',(198.712855715638,94.5869185538863,341.657337824743));
#24390=CARTESIAN_POINT('Ctrl Pts',(198.194027083786,94.5457202173699,340.465809699669));
#24391=CARTESIAN_POINT('Ctrl Pts',(198.052975944774,94.5240190759957,339.815848082118));
#24392=CARTESIAN_POINT('Ctrl Pts',(198.031231811742,94.4820586634371,338.51673499509));
#24393=CARTESIAN_POINT('Ctrl Pts',(198.143708038422,94.4631751514099,337.880087191142));
#24394=CARTESIAN_POINT('Ctrl Pts',(198.60946696214,94.4220544753107,336.666551603344));
#24395=CARTESIAN_POINT('Ctrl Pts',(198.965075297147,94.4003441502341,336.10385695742));
#24396=CARTESIAN_POINT('Ctrl Pts',(199.86107981855,94.3583245940889,335.162505522918));
#24397=CARTESIAN_POINT('Ctrl Pts',(200.387613677733,94.3394012193826,334.787767126957));
#24398=CARTESIAN_POINT('Ctrl Pts',(201.571016569693,94.298357864262,334.249313254273));
#24399=CARTESIAN_POINT('Ctrl Pts',(202.21970361048,94.2766399062661,334.097620224748));
#24400=CARTESIAN_POINT('Ctrl Pts',(203.518965300925,94.2345636881629,334.055459895413));
#24401=CARTESIAN_POINT('Ctrl Pts',(204.15689484424,94.2155936670697,334.157780847878));
#24402=CARTESIAN_POINT('Ctrl Pts',(205.378295284628,94.1746269898073,334.604344431639));
#24403=CARTESIAN_POINT('Ctrl Pts',(205.947397761897,94.1529028755505,334.95167017361));
#24404=CARTESIAN_POINT('Ctrl Pts',(206.902899459118,94.1107725445201,335.833627778178));
#24405=CARTESIAN_POINT('Ctrl Pts',(207.285517675167,94.0917497990019,336.35405246242));
#24406=CARTESIAN_POINT('Ctrl Pts',(207.842570099924,94.0508588661002,337.529582916972));
#24407=CARTESIAN_POINT('Ctrl Pts',(208.004370268359,94.0291299852868,338.176902674053));
#24408=CARTESIAN_POINT('Ctrl Pts',(208.057243536243,93.9929070890982,339.292622106622));
#24409=CARTESIAN_POINT('Ctrl Pts',(208.016331894512,93.978454139632,339.748263576678));
#24410=CARTESIAN_POINT('Ctrl Pts',(207.914727694784,93.9647376097703,340.191287620971));
#24411=CARTESIAN_POINT('Ctrl Pts',(207.914727694784,93.8397376070391,340.191287620971));
#24412=CARTESIAN_POINT('Ctrl Pts',(207.935967918546,93.8426050294909,340.098674029625));
#24413=CARTESIAN_POINT('Ctrl Pts',(207.954588856772,93.8455090974102,340.005364892963));
#24414=CARTESIAN_POINT('Ctrl Pts',(208.078884475172,93.8683852535681,339.274122305723));
#24415=CARTESIAN_POINT('Ctrl Pts',(208.062584791422,93.8894843264772,338.62179155748));
#24416=CARTESIAN_POINT('Ctrl Pts',(207.779834645017,93.9320720445258,337.34726825639));
#24417=CARTESIAN_POINT('Ctrl Pts',(207.511284980159,93.9524504634837,336.738401830215));
#24418=CARTESIAN_POINT('Ctrl Pts',(206.75007369525,93.9932226693162,335.65496881214));
#24419=CARTESIAN_POINT('Ctrl Pts',(206.262967114288,94.0149436030176,335.192503985698));
#24420=CARTESIAN_POINT('Ctrl Pts',(205.157177240321,94.0575202620966,334.498311406653));
#24421=CARTESIAN_POINT('Ctrl Pts',(204.554237298208,94.0773596066746,334.265145804384));
#24422=CARTESIAN_POINT('Ctrl Pts',(203.26880863012,94.1175076261342,334.034648111059));
#24423=CARTESIAN_POINT('Ctrl Pts',(202.596978886693,94.1392247945297,334.049121097658));
#24424=CARTESIAN_POINT('Ctrl Pts',(201.322527127607,94.181825940921,334.33476443115));
#24425=CARTESIAN_POINT('Ctrl Pts',(200.730071495465,94.201735081733,334.593760553116));
#24426=CARTESIAN_POINT('Ctrl Pts',(199.654655314064,94.2418345342463,335.335400052225));
#24427=CARTESIAN_POINT('Ctrl Pts',(199.187619668244,94.2635477724379,335.818967168767));
#24428=CARTESIAN_POINT('Ctrl Pts',(198.483717999202,94.3061716474694,336.9196265378));
#24429=CARTESIAN_POINT('Ctrl Pts',(198.245453322367,94.3261485581309,337.520872530092));
#24430=CARTESIAN_POINT('Ctrl Pts',(198.004245813119,94.3662019884901,338.805172568024));
#24431=CARTESIAN_POINT('Ctrl Pts',(198.013314859826,94.3879111915484,339.477667365453));
#24432=CARTESIAN_POINT('Ctrl Pts',(198.289069313759,94.4305561402753,340.755148662006));
#24433=CARTESIAN_POINT('Ctrl Pts',(198.543545720082,94.4505985666671,341.349871025278));
#24434=CARTESIAN_POINT('Ctrl Pts',(199.277301834465,94.4906084776871,342.431643005062));
#24435=CARTESIAN_POINT('Ctrl Pts',(199.757703001535,94.5123135926319,342.902701650533));
#24436=CARTESIAN_POINT('Ctrl Pts',(200.853785712487,94.5549780616054,343.615183736526));
#24437=CARTESIAN_POINT('Ctrl Pts',(201.453535775631,94.5750835715499,343.857957267027));
#24438=CARTESIAN_POINT('Ctrl Pts',(202.736805082043,94.6150524111144,344.108615782547));
#24439=CARTESIAN_POINT('Ctrl Pts',(203.409851783221,94.6367534297841,344.104320766872));
#24440=CARTESIAN_POINT('Ctrl Pts',(204.689975400976,94.679435964273,343.837304914196));
#24441=CARTESIAN_POINT('Ctrl Pts',(205.286697065872,94.6996019930009,343.586811426813));
#24442=CARTESIAN_POINT('Ctrl Pts',(206.374039189645,94.739532143181,342.860012590828));
#24443=CARTESIAN_POINT('Ctrl Pts',(206.848618578616,94.7612290955408,342.382421692139));
#24444=CARTESIAN_POINT('Ctrl Pts',(207.544595588626,94.8025025722738,341.326856142823));
#24445=CARTESIAN_POINT('Ctrl Pts',(207.781276655283,94.8217217654369,340.773173206348));
#24446=CARTESIAN_POINT('Ctrl Pts',(207.914727694784,94.8397376070391,340.191287620971));
#24447=CARTESIAN_POINT('Origin',(203.041252647846,100.739737607039,339.073593133701));
#24448=CARTESIAN_POINT('',(207.914727694784,95.9647376097703,340.191287620971));
#24449=CARTESIAN_POINT('',(207.914727694784,95.8397376070391,340.191287620971));
#24450=CARTESIAN_POINT('',(207.914727694784,100.739737607039,340.191287620971));
#24451=CARTESIAN_POINT('Ctrl Pts',(207.914727694784,95.9647376097703,340.191287620971));
#24452=CARTESIAN_POINT('Ctrl Pts',(207.824263172267,95.9525249322641,340.585739412711));
#24453=CARTESIAN_POINT('Ctrl Pts',(207.686054272076,95.9397175076353,340.968582041799));
#24454=CARTESIAN_POINT('Ctrl Pts',(207.20512380531,95.9053149036476,341.918957645222));
#24455=CARTESIAN_POINT('Ctrl Pts',(206.794450792268,95.8836127170631,342.44218957209));
#24456=CARTESIAN_POINT('Ctrl Pts',(205.807483630078,95.8424225905177,343.287698268786));
#24457=CARTESIAN_POINT('Ctrl Pts',(205.245149638245,95.8235684514315,343.607195840309));
#24458=CARTESIAN_POINT('Ctrl Pts',(204.014103711322,95.7816629611206,344.02200347778));
#24459=CARTESIAN_POINT('Ctrl Pts',(203.354969091086,95.7599713954899,344.106961722735));
#24460=CARTESIAN_POINT('Ctrl Pts',(202.058642119951,95.7187035695358,344.017842980232));
#24461=CARTESIAN_POINT('Ctrl Pts',(201.433368033154,95.6998747209822,343.851232320508));
#24462=CARTESIAN_POINT('Ctrl Pts',(200.2650806948,95.6580327952419,343.283741113733));
#24463=CARTESIAN_POINT('Ctrl Pts',(199.735999749879,95.6363534977267,342.882502476767));
#24464=CARTESIAN_POINT('Ctrl Pts',(198.87415919352,95.5950082285125,341.910306276557));
#24465=CARTESIAN_POINT('Ctrl Pts',(198.544931499865,95.5761962200961,341.352782574673));
#24466=CARTESIAN_POINT('Ctrl Pts',(198.109971183988,95.5344199939846,340.129152463659));
#24467=CARTESIAN_POINT('Ctrl Pts',(198.014078349114,95.5127546353721,339.472677632615));
#24468=CARTESIAN_POINT('Ctrl Pts',(198.080882444736,95.4713324948658,338.175326953219));
#24469=CARTESIAN_POINT('Ctrl Pts',(198.237066249138,95.4525284799068,337.546521770783));
#24470=CARTESIAN_POINT('Ctrl Pts',(198.784812691329,95.4108199169436,336.369203664002));
#24471=CARTESIAN_POINT('Ctrl Pts',(199.176290275722,95.389170170719,335.834291671704));
#24472=CARTESIAN_POINT('Ctrl Pts',(200.133192131337,95.3476720410362,334.955832806825));
#24473=CARTESIAN_POINT('Ctrl Pts',(200.68578868709,95.3288668896484,334.616626099003));
#24474=CARTESIAN_POINT('Ctrl Pts',(201.901705512363,95.2872277570585,334.16119097772));
#24475=CARTESIAN_POINT('Ctrl Pts',(202.555289211908,95.2655952775083,334.054220280177));
#24476=CARTESIAN_POINT('Ctrl Pts',(203.853482080545,95.2240223401788,334.098281489444));
#24477=CARTESIAN_POINT('Ctrl Pts',(204.485888896634,95.2052067610264,334.243844829991));
#24478=CARTESIAN_POINT('Ctrl Pts',(205.672192442344,95.1636386066622,334.771538039933));
#24479=CARTESIAN_POINT('Ctrl Pts',(206.212829695502,95.1420250074677,335.153054898725));
#24480=CARTESIAN_POINT('Ctrl Pts',(207.107967541355,95.1003787086922,336.094329255662));
#24481=CARTESIAN_POINT('Ctrl Pts',(207.457275026156,95.0815434134856,336.641941425247));
#24482=CARTESIAN_POINT('Ctrl Pts',(207.933233032709,95.0400475274432,337.849945808571));
#24483=CARTESIAN_POINT('Ctrl Pts',(208.051270303984,95.0184543591605,338.50044057598));
#24484=CARTESIAN_POINT('Ctrl Pts',(208.034882521879,94.986195370895,339.504782372743));
#24485=CARTESIAN_POINT('Ctrl Pts',(207.992537096821,94.9752418506327,339.852015857925));
#24486=CARTESIAN_POINT('Ctrl Pts',(207.914727694784,94.9647376097703,340.191287620971));
#24487=CARTESIAN_POINT('Ctrl Pts',(207.914727694784,94.8397376070391,340.191287620971));
#24488=CARTESIAN_POINT('Ctrl Pts',(207.924478876109,94.8410540129572,340.148769616808));
#24489=CARTESIAN_POINT('Ctrl Pts',(207.933678816981,94.842378252787,340.106101453216));
#24490=CARTESIAN_POINT('Ctrl Pts',(208.074323715298,94.8640459954571,339.409617319055));
#24491=CARTESIAN_POINT('Ctrl Pts',(208.074220596045,94.8857389434083,338.736113468209));
#24492=CARTESIAN_POINT('Ctrl Pts',(207.814880178946,94.9284536222466,337.453695970922));
#24493=CARTESIAN_POINT('Ctrl Pts',(207.567876777328,94.9487326644126,336.855221071499));
#24494=CARTESIAN_POINT('Ctrl Pts',(206.84718163009,94.9885922760571,335.763021977389));
#24495=CARTESIAN_POINT('Ctrl Pts',(206.372068480412,95.010281307781,335.285376670134));
#24496=CARTESIAN_POINT('Ctrl Pts',(205.283606284448,95.0530102443135,334.558772549594));
#24497=CARTESIAN_POINT('Ctrl Pts',(204.686316632632,95.0733417029364,334.308571751955));
#24498=CARTESIAN_POINT('Ctrl Pts',(203.404811224976,95.1131692964387,334.042386023179));
#24499=CARTESIAN_POINT('Ctrl Pts',(202.730929048368,95.1348545212918,334.038828048661));
#24500=CARTESIAN_POINT('Ctrl Pts',(201.446528139775,95.177596617987,334.291462750351));
#24501=CARTESIAN_POINT('Ctrl Pts',(200.846523620691,95.1979777630694,334.535423125413));
#24502=CARTESIAN_POINT('Ctrl Pts',(199.750108106285,95.2377753857359,335.250791257824));
#24503=CARTESIAN_POINT('Ctrl Pts',(199.269804452855,95.2594569296941,335.723732747906));
#24504=CARTESIAN_POINT('Ctrl Pts',(198.537473854873,95.3022111675649,336.8090732653));
#24505=CARTESIAN_POINT('Ctrl Pts',(198.284258664357,95.3226392971829,337.405365613395));
#24506=CARTESIAN_POINT('Ctrl Pts',(198.011786296759,95.3624089027797,338.686132005916));
#24507=CARTESIAN_POINT('Ctrl Pts',(198.005045724529,95.3840869044169,339.360327242861));
#24508=CARTESIAN_POINT('Ctrl Pts',(198.251849241647,95.4268523385324,340.6464372243));
#24509=CARTESIAN_POINT('Ctrl Pts',(198.493167953972,95.4473247985227,341.247770309472));
#24510=CARTESIAN_POINT('Ctrl Pts',(199.203908026909,95.4870682459829,342.347832116528));
#24511=CARTESIAN_POINT('Ctrl Pts',(199.674955959615,95.5087428529601,342.830432130254));
#24512=CARTESIAN_POINT('Ctrl Pts',(200.757578011136,95.5515186079928,343.567722277944));
#24513=CARTESIAN_POINT('Ctrl Pts',(201.353006720452,95.5720328081105,343.823549536321));
#24514=CARTESIAN_POINT('Ctrl Pts',(202.633122059699,95.6117518612847,344.101462174638));
#24515=CARTESIAN_POINT('Ctrl Pts',(203.307576481301,95.6334232273167,344.110958177241));
#24516=CARTESIAN_POINT('Ctrl Pts',(204.595154818141,95.6762084931767,343.869204754764));
#24517=CARTESIAN_POINT('Ctrl Pts',(205.197637349002,95.6967619200548,343.630170553606));
#24518=CARTESIAN_POINT('Ctrl Pts',(206.30084191883,95.7364582483519,342.923435407913));
#24519=CARTESIAN_POINT('Ctrl Pts',(206.785419220041,95.7581265306177,342.454031136491));
#24520=CARTESIAN_POINT('Ctrl Pts',(207.519374714258,95.8004811281553,341.38485900205));
#24521=CARTESIAN_POINT('Ctrl Pts',(207.774213604633,95.8207682561783,340.803970174115));
#24522=CARTESIAN_POINT('Ctrl Pts',(207.914727694784,95.8397376070391,340.191287620971));
#24523=CARTESIAN_POINT('Origin',(203.041252647846,100.739737607039,339.073593133701));
#24524=CARTESIAN_POINT('',(207.914727694784,96.9647376097703,340.191287620971));
#24525=CARTESIAN_POINT('',(207.914727695617,96.8397376072638,340.191287617342));
#24526=CARTESIAN_POINT('',(207.914727694784,100.739737607039,340.191287620971));
#24527=CARTESIAN_POINT('Ctrl Pts',(207.914727694784,96.9647376097703,340.191287620971));
#24528=CARTESIAN_POINT('Ctrl Pts',(207.802758576459,96.9496218196826,340.679505743544));
#24529=CARTESIAN_POINT('Ctrl Pts',(207.617885049872,96.9336271777375,341.148895869011));
#24530=CARTESIAN_POINT('Ctrl Pts',(207.033046171459,96.8957326294959,342.156559782157));
#24531=CARTESIAN_POINT('Ctrl Pts',(206.589773997112,96.873996568844,342.657882666583));
#24532=CARTESIAN_POINT('Ctrl Pts',(205.551746357524,96.8334013638026,343.44473295342));
#24533=CARTESIAN_POINT('Ctrl Pts',(204.972328379496,96.8141145725655,343.729815324878));
#24534=CARTESIAN_POINT('Ctrl Pts',(203.715974179417,96.7717892909509,344.071920067185));
#24535=CARTESIAN_POINT('Ctrl Pts',(203.048772405948,96.7500533743099,344.117252401768));
#24536=CARTESIAN_POINT('Ctrl Pts',(201.757683954315,96.7093888818263,343.948209884819));
#24537=CARTESIAN_POINT('Ctrl Pts',(201.145037418942,96.6901718243182,343.744119645876));
#24538=CARTESIAN_POINT('Ctrl Pts',(200.010917971376,96.6478900055346,343.10534129423));
#24539=CARTESIAN_POINT('Ctrl Pts',(199.504486762997,96.6261551884195,342.669318414581));
#24540=CARTESIAN_POINT('Ctrl Pts',(198.704275191607,96.5854194963093,341.64265857057));
#24541=CARTESIAN_POINT('Ctrl Pts',(198.411418202559,96.5662692169798,341.067111015307));
#24542=CARTESIAN_POINT('Ctrl Pts',(198.052703007714,96.5240334352275,339.816339987299));
#24543=CARTESIAN_POINT('Ctrl Pts',(197.998299814888,96.50230078477,339.150771078765));
#24544=CARTESIAN_POINT('Ctrl Pts',(198.149161486812,96.4614921819654,337.858277818631));
#24545=CARTESIAN_POINT('Ctrl Pts',(198.344699968257,96.4424049656356,337.242760738268));
#24546=CARTESIAN_POINT('Ctrl Pts',(198.967183994334,96.4002178223554,336.100610832859));
#24547=CARTESIAN_POINT('Ctrl Pts',(199.39532605161,96.378488515302,335.588782491954));
#24548=CARTESIAN_POINT('Ctrl Pts',(200.409639746461,96.3376055173355,334.774257765139));
#24549=CARTESIAN_POINT('Ctrl Pts',(200.981029093973,96.3185768779145,334.473032872092));
#24550=CARTESIAN_POINT('Ctrl Pts',(202.225700550231,96.2764409817612,334.096558489346));
#24551=CARTESIAN_POINT('Ctrl Pts',(202.889386226885,96.254716299989,334.032466287752));
#24552=CARTESIAN_POINT('Ctrl Pts',(204.183246902875,96.2137576725481,334.163838007811));
#24553=CARTESIAN_POINT('Ctrl Pts',(204.801842125211,96.1947823566162,334.350228466268));
#24554=CARTESIAN_POINT('Ctrl Pts',(205.952429364643,96.152700301268,334.955295933928));
#24555=CARTESIAN_POINT('Ctrl Pts',(206.469882603075,96.130981624657,335.374966376931));
#24556=CARTESIAN_POINT('Ctrl Pts',(207.299557325334,96.0899464045161,336.376016829161));
#24557=CARTESIAN_POINT('Ctrl Pts',(207.609688134916,96.0710184111409,336.942988721906));
#24558=CARTESIAN_POINT('Ctrl Pts',(208.004923802077,96.0289927512247,338.181070053893));
#24559=CARTESIAN_POINT('Ctrl Pts',(208.079237868111,96.0072815478085,338.842611471355));
#24560=CARTESIAN_POINT('Ctrl Pts',(208.003131952573,95.9790228405794,339.732835166694));
#24561=CARTESIAN_POINT('Ctrl Pts',(207.966858318546,95.9717752249422,339.963982845851));
#24562=CARTESIAN_POINT('Ctrl Pts',(207.914727694784,95.9647376097703,340.191287620971));
#24563=CARTESIAN_POINT('Ctrl Pts',(207.914727694784,95.8397376070391,340.191287620971));
#24564=CARTESIAN_POINT('Ctrl Pts',(207.917733844739,95.8401434361853,340.178179927447));
#24565=CARTESIAN_POINT('Ctrl Pts',(207.920687659849,95.8405500173302,340.16505772174));
#24566=CARTESIAN_POINT('Ctrl Pts',(208.067676524099,95.861185965235,339.499537617138));
#24567=CARTESIAN_POINT('Ctrl Pts',(208.079549757705,95.8828513221919,338.824868410798));
#24568=CARTESIAN_POINT('Ctrl Pts',(207.842154541268,95.9256534193295,337.536031690224));
#24569=CARTESIAN_POINT('Ctrl Pts',(207.605089455537,95.9462781151005,336.932558046077));
#24570=CARTESIAN_POINT('Ctrl Pts',(206.901808138952,95.9859336316715,335.826652492034));
#24571=CARTESIAN_POINT('Ctrl Pts',(206.433825071212,96.0075962212339,335.34037734793));
#24572=CARTESIAN_POINT('Ctrl Pts',(205.355596669194,96.0504057487236,334.595124501188));
#24573=CARTESIAN_POINT('Ctrl Pts',(204.761554490437,96.0710626810747,334.335100588781));
#24574=CARTESIAN_POINT('Ctrl Pts',(203.48250572603,96.1106999312182,334.048461908613));
#24575=CARTESIAN_POINT('Ctrl Pts',(202.807658305392,96.1323599092629,334.034543937213));
#24576=CARTESIAN_POINT('Ctrl Pts',(201.517745444591,96.1751762771804,334.268189510977));
#24577=CARTESIAN_POINT('Ctrl Pts',(200.913419707451,96.1958633175214,334.503562189406));
#24578=CARTESIAN_POINT('Ctrl Pts',(199.805198588,96.235483612383,335.20387374646));
#24579=CARTESIAN_POINT('Ctrl Pts',(199.317469007499,96.2571411315419,335.670632076405));
#24580=CARTESIAN_POINT('Ctrl Pts',(198.569056120019,96.2999637957029,336.74710683773));
#24581=CARTESIAN_POINT('Ctrl Pts',(198.307365685623,96.3206789206186,337.340598748464));
#24582=CARTESIAN_POINT('Ctrl Pts',(198.017266886641,96.3602834889125,338.619216989787));
#24583=CARTESIAN_POINT('Ctrl Pts',(198.00159474125,96.3819386976183,339.294212494069));
#24584=CARTESIAN_POINT('Ctrl Pts',(198.232022732549,96.4247671562484,340.585043979386));
#24585=CARTESIAN_POINT('Ctrl Pts',(198.465944416523,96.4455084479489,341.190100444113));
#24586=CARTESIAN_POINT('Ctrl Pts',(199.163708936799,96.4850984393755,342.300302492973));
#24587=CARTESIAN_POINT('Ctrl Pts',(199.629414875849,96.5067514811264,342.789275472743));
#24588=CARTESIAN_POINT('Ctrl Pts',(200.704383676333,96.5495852717304,343.540393904999));
#24589=CARTESIAN_POINT('Ctrl Pts',(201.297404439508,96.5703509173616,343.803511674489));
#24590=CARTESIAN_POINT('Ctrl Pts',(202.575650815693,96.6099274061719,344.096571660111));
#24591=CARTESIAN_POINT('Ctrl Pts',(203.250769555504,96.6315784189847,344.113745348026));
#24592=CARTESIAN_POINT('Ctrl Pts',(204.542310650037,96.6744146825828,343.88608507479));
#24593=CARTESIAN_POINT('Ctrl Pts',(205.14800052983,96.6951880189483,343.653432514059));
#24594=CARTESIAN_POINT('Ctrl Pts',(206.259678905628,96.7347749658355,342.957982630121));
#24595=CARTESIAN_POINT('Ctrl Pts',(206.749582166859,96.7563997669483,342.493414757975));
#24596=CARTESIAN_POINT('Ctrl Pts',(207.503033771944,96.7992350732268,341.420048159803));
#24597=CARTESIAN_POINT('Ctrl Pts',(207.767488036637,96.8200152451585,340.827475204036));
#24598=CARTESIAN_POINT('Ctrl Pts',(207.913228308978,96.8395355905515,340.197810353621));
#24599=CARTESIAN_POINT('Ctrl Pts',(207.913979658144,96.8396366223653,340.194549279651));
#24600=CARTESIAN_POINT('Ctrl Pts',(207.914727696449,96.8397376072639,340.191287613713));
#24601=CARTESIAN_POINT('Origin',(203.041252647846,100.739737607039,339.073593133701));
#24602=CARTESIAN_POINT('',(207.914727694784,97.9647376097703,340.191287620971));
#24603=CARTESIAN_POINT('',(207.914727694784,97.8397376070391,340.191287620971));
#24604=CARTESIAN_POINT('',(207.914727694784,100.739737607039,340.191287620971));
#24605=CARTESIAN_POINT('Ctrl Pts',(207.914727694784,97.9647376097703,340.191287620971));
#24606=CARTESIAN_POINT('Ctrl Pts',(207.787344310009,97.9475408993404,340.746716456103));
#24607=CARTESIAN_POINT('Ctrl Pts',(207.565819195648,97.9292362257558,341.276822047888));
#24608=CARTESIAN_POINT('Ctrl Pts',(206.901920889685,97.8889040001007,342.319839977017));
#24609=CARTESIAN_POINT('Ctrl Pts',(206.43604964038,97.8671886475898,342.804314532998));
#24610=CARTESIAN_POINT('Ctrl Pts',(205.362471371289,97.8270635922768,343.548222783882));
#24611=CARTESIAN_POINT('Ctrl Pts',(204.770668362569,97.807191468124,343.808521014367));
#24612=CARTESIAN_POINT('Ctrl Pts',(203.497095441832,97.7646031657314,344.097007748173));
#24613=CARTESIAN_POINT('Ctrl Pts',(202.825464906029,97.7428839628591,344.113034782473));
#24614=CARTESIAN_POINT('Ctrl Pts',(201.539719183794,97.7027089703224,343.88561945709));
#24615=CARTESIAN_POINT('Ctrl Pts',(200.936291916441,97.682907612388,343.653919449903));
#24616=CARTESIAN_POINT('Ctrl Pts',(199.829036312802,97.6403447783789,342.962518401829));
#24617=CARTESIAN_POINT('Ctrl Pts',(199.340920528111,97.6186219243762,342.501371361285));
#24618=CARTESIAN_POINT('Ctrl Pts',(198.58786600622,97.5783944155194,341.435242719625));
#24619=CARTESIAN_POINT('Ctrl Pts',(198.322311749214,97.5586653959233,340.846072140563));
#24620=CARTESIAN_POINT('Ctrl Pts',(198.022373280032,97.5161299491114,339.5760737029));
#24621=CARTESIAN_POINT('Ctrl Pts',(198.000086686688,97.4944037145157,338.90528166429));
#24622=CARTESIAN_POINT('Ctrl Pts',(198.21507454351,97.4541211107053,337.618292996073));
#24623=CARTESIAN_POINT('Ctrl Pts',(198.440874064337,97.4344656325874,337.012901703184));
#24624=CARTESIAN_POINT('Ctrl Pts',(199.121033095641,97.3919595955806,335.899785438682));
#24625=CARTESIAN_POINT('Ctrl Pts',(199.576857259965,97.3702303299924,335.407643650929));
#24626=CARTESIAN_POINT('Ctrl Pts',(200.634604874495,97.3298900735479,334.644393824861));
#24627=CARTESIAN_POINT('Ctrl Pts',(201.220838033555,97.3103089114501,334.37296716565));
#24628=CARTESIAN_POINT('Ctrl Pts',(202.486792604429,97.267834408313,334.060284171213));
#24629=CARTESIAN_POINT('Ctrl Pts',(203.156583106232,97.2461025479247,334.031030878434));
#24630=CARTESIAN_POINT('Ctrl Pts',(204.44489054434,97.2057021245588,334.232163093726));
#24631=CARTESIAN_POINT('Ctrl Pts',(205.052470447681,97.1861955643755,334.451399251097));
#24632=CARTESIAN_POINT('Ctrl Pts',(206.172029626128,97.1437548165742,335.119048848787));
#24633=CARTESIAN_POINT('Ctrl Pts',(206.668579130893,97.1220208912257,335.568920805684));
#24634=CARTESIAN_POINT('Ctrl Pts',(207.443095964537,97.0815578542201,336.617310321601));
#24635=CARTESIAN_POINT('Ctrl Pts',(207.721030489256,97.0621256342267,337.200292870474));
#24636=CARTESIAN_POINT('Ctrl Pts',(208.047773151692,97.0197209546451,338.461705833607));
#24637=CARTESIAN_POINT('Ctrl Pts',(208.084711340844,96.9979855941344,339.130307545868));
#24638=CARTESIAN_POINT('Ctrl Pts',(207.970544832191,96.9730848870396,339.922698137084));
#24639=CARTESIAN_POINT('Ctrl Pts',(207.945365996894,96.9688737693673,340.057695657771));
#24640=CARTESIAN_POINT('Ctrl Pts',(207.914727694784,96.9647376097703,340.191287620971));
#24641=CARTESIAN_POINT('Ctrl Pts',(207.914727696449,96.8397376072638,340.191287613713));
#24642=CARTESIAN_POINT('Ctrl Pts',(208.063328933394,96.8597987201314,339.543342729492));
#24643=CARTESIAN_POINT('Ctrl Pts',(208.08124770444,96.8813197613063,338.872133546454));
#24644=CARTESIAN_POINT('Ctrl Pts',(207.857183886755,96.9240413712455,337.583545012411));
#24645=CARTESIAN_POINT('Ctrl Pts',(207.625856930496,96.9448288876363,336.977191066835));
#24646=CARTESIAN_POINT('Ctrl Pts',(206.93304948772,96.9844430827078,335.864220560912));
#24647=CARTESIAN_POINT('Ctrl Pts',(206.469956438707,97.0060063639469,335.373555488612));
#24648=CARTESIAN_POINT('Ctrl Pts',(205.398715375365,97.0488325593009,334.617596147755));
#24649=CARTESIAN_POINT('Ctrl Pts',(204.806648547122,97.0696279611766,334.351625580777));
#24650=CARTESIAN_POINT('Ctrl Pts',(203.530305761832,97.1092573479852,334.052970476787));
#24651=CARTESIAN_POINT('Ctrl Pts',(202.856178857879,97.1307865267325,334.032590951377));
#24652=CARTESIAN_POINT('Ctrl Pts',(201.564004220546,97.1736075615292,334.253698191725));
#24653=CARTESIAN_POINT('Ctrl Pts',(200.956882423605,97.1944114231065,334.483482987031));
#24654=CARTESIAN_POINT('Ctrl Pts',(199.842414909669,97.2340571395576,335.173220322507));
#24655=CARTESIAN_POINT('Ctrl Pts',(199.350867401544,97.2555498199762,335.634602701572));
#24656=CARTESIAN_POINT('Ctrl Pts',(198.592002627439,97.298365242755,336.703373002197));
#24657=CARTESIAN_POINT('Ctrl Pts',(198.324273365712,97.3191781723567,337.294847654029));
#24658=CARTESIAN_POINT('Ctrl Pts',(198.022141535132,97.3588414296567,338.569990487973));
#24659=CARTESIAN_POINT('Ctrl Pts',(197.999789315069,97.380295088947,339.243486651965));
#24660=CARTESIAN_POINT('Ctrl Pts',(198.216804747761,97.4231044082145,340.535988376863));
#24661=CARTESIAN_POINT('Ctrl Pts',(198.444798541592,97.4439270490012,341.143995608951));
#24662=CARTESIAN_POINT('Ctrl Pts',(199.130975740103,97.4836091344146,342.260193371317));
#24663=CARTESIAN_POINT('Ctrl Pts',(199.590378227264,97.5050211231525,342.752760609713));
#24664=CARTESIAN_POINT('Ctrl Pts',(200.656281796591,97.5478238038946,343.514983608002));
#24665=CARTESIAN_POINT('Ctrl Pts',(201.247064215775,97.5686568343686,343.784748201602));
#24666=CARTESIAN_POINT('Ctrl Pts',(202.520812401028,97.6083591137349,344.090902697033));
#24667=CARTESIAN_POINT('Ctrl Pts',(203.193578172053,97.6297266576778,344.115534002417));
#24668=CARTESIAN_POINT('Ctrl Pts',(204.486448535759,97.672522117612,343.903250727198));
#24669=CARTESIAN_POINT('Ctrl Pts',(205.09547356045,97.693366251844,343.677332749677));
#24670=CARTESIAN_POINT('Ctrl Pts',(206.213665650385,97.7330901717824,342.995274731163));
#24671=CARTESIAN_POINT('Ctrl Pts',(206.707408045531,97.7544103753982,342.538157922658));
#24672=CARTESIAN_POINT('Ctrl Pts',(207.473501983227,97.7971979809594,341.475573328025));
#24673=CARTESIAN_POINT('Ctrl Pts',(207.745616027229,97.8180539684817,340.885599218779));
#24674=CARTESIAN_POINT('Ctrl Pts',(207.904004576751,97.8383099149618,340.237295052471));
#24675=CARTESIAN_POINT('Ctrl Pts',(207.909448526219,97.8390249212105,340.214306340814));
#24676=CARTESIAN_POINT('Ctrl Pts',(207.914727694784,97.8397376070391,340.191287620971));
#24677=CARTESIAN_POINT('Origin',(203.041252647846,100.739737607039,339.073593133701));
#24678=CARTESIAN_POINT('',(207.914727694784,98.9647376097703,340.191287620971));
#24679=CARTESIAN_POINT('',(207.914727694784,98.8397376070391,340.191287620971));
#24680=CARTESIAN_POINT('',(207.914727694784,100.739737607039,340.191287620971));
#24681=CARTESIAN_POINT('Ctrl Pts',(207.914727694784,98.9647376097703,340.191287620971));
#24682=CARTESIAN_POINT('Ctrl Pts',(207.777720932146,98.946241746843,340.788677199773));
#24683=CARTESIAN_POINT('Ctrl Pts',(207.531967934148,98.9264853686005,341.356088920239));
#24684=CARTESIAN_POINT('Ctrl Pts',(206.816955231582,98.8846656052097,342.418639843526));
#24685=CARTESIAN_POINT('Ctrl Pts',(206.337323742344,98.8629821131841,342.892132496792));
#24686=CARTESIAN_POINT('Ctrl Pts',(205.241974815253,98.8231687433469,343.608850647877));
#24687=CARTESIAN_POINT('Ctrl Pts',(204.642357902887,98.8028137788264,343.853581963425));
#24688=CARTESIAN_POINT('Ctrl Pts',(203.358458006767,98.7600785743928,344.107916703837));
#24689=CARTESIAN_POINT('Ctrl Pts',(202.684669887813,98.7383913324243,344.105286778262));
#24690=CARTESIAN_POINT('Ctrl Pts',(201.402951603227,98.6985469105573,343.84093487211));
#24691=CARTESIAN_POINT('Ctrl Pts',(200.80537116807,98.678243087483,343.591612575252));
#24692=CARTESIAN_POINT('Ctrl Pts',(199.716002334855,98.6355216189368,342.866677931433));
#24693=CARTESIAN_POINT('Ctrl Pts',(199.240259038187,98.6138305093857,342.389809004803));
#24694=CARTESIAN_POINT('Ctrl Pts',(198.518014230854,98.5739529391946,341.298840423343));
#24695=CARTESIAN_POINT('Ctrl Pts',(198.270125087002,98.5537029931734,340.700810587759));
#24696=CARTESIAN_POINT('Ctrl Pts',(198.008835158704,98.5109964017973,339.418973330549));
#24697=CARTESIAN_POINT('Ctrl Pts',(198.007667454863,98.4893013260074,338.745583151298));
#24698=CARTESIAN_POINT('Ctrl Pts',(198.264512112369,98.4493884220293,337.463006106893));
#24699=CARTESIAN_POINT('Ctrl Pts',(198.510241726302,98.4291950789849,336.864235846117));
#24700=CARTESIAN_POINT('Ctrl Pts',(199.228346402579,98.3865045914073,335.771173993807));
#24701=CARTESIAN_POINT('Ctrl Pts',(199.702032695211,98.3648054745532,335.292866694799));
#24702=CARTESIAN_POINT('Ctrl Pts',(200.787961132659,98.3248549668108,334.564297820753));
#24703=CARTESIAN_POINT('Ctrl Pts',(201.384174238201,98.304720913041,334.312791512603));
#24704=CARTESIAN_POINT('Ctrl Pts',(202.663628399212,98.2620478454922,334.043551398921));
#24705=CARTESIAN_POINT('Ctrl Pts',(203.336537802058,98.2403446419795,334.038041373913));
#24706=CARTESIAN_POINT('Ctrl Pts',(204.6200724226,98.2003541822505,334.286295452556));
#24707=CARTESIAN_POINT('Ctrl Pts',(205.220203173367,98.1802820300518,334.527921049304));
#24708=CARTESIAN_POINT('Ctrl Pts',(206.317454637024,98.1376277923591,335.238219079962));
#24709=CARTESIAN_POINT('Ctrl Pts',(206.798665037818,98.1159204917686,335.708255199108));
#24710=CARTESIAN_POINT('Ctrl Pts',(207.534431521013,98.0758876616242,336.788410847114));
#24711=CARTESIAN_POINT('Ctrl Pts',(207.790059825899,98.0558799103887,337.382555301657));
#24712=CARTESIAN_POINT('Ctrl Pts',(208.068337373195,98.0132460095855,338.659267602543));
#24713=CARTESIAN_POINT('Ctrl Pts',(208.078785073144,97.9915346431374,339.331596807135));
#24714=CARTESIAN_POINT('Ctrl Pts',(207.944503674349,97.9689676904175,340.05492519118));
#24715=CARTESIAN_POINT('Ctrl Pts',(207.930321147104,97.9668427201395,340.123295605584));
#24716=CARTESIAN_POINT('Ctrl Pts',(207.914727694784,97.9647376097703,340.191287620971));
#24717=CARTESIAN_POINT('Ctrl Pts',(207.914727694784,97.8397376070391,340.191287620971));
#24718=CARTESIAN_POINT('Ctrl Pts',(208.058182547195,97.8591039597311,339.56578248379));
#24719=CARTESIAN_POINT('Ctrl Pts',(208.07993750736,97.8798428986119,338.918208288944));
#24720=CARTESIAN_POINT('Ctrl Pts',(207.876844768975,97.921849972268,337.648264029656));
#24721=CARTESIAN_POINT('Ctrl Pts',(207.653327094259,97.9427185975742,337.038073358269));
#24722=CARTESIAN_POINT('Ctrl Pts',(206.976022784969,97.982490470181,335.91758985581));
#24723=CARTESIAN_POINT('Ctrl Pts',(206.521536947544,98.0037068514112,335.42249745158));
#24724=CARTESIAN_POINT('Ctrl Pts',(205.462785275897,98.0464766207395,334.651955691748));
#24725=CARTESIAN_POINT('Ctrl Pts',(204.873753760568,98.0673587023253,334.377137639582));
#24726=CARTESIAN_POINT('Ctrl Pts',(203.603496057517,98.10715705557,334.060999305767));
#24727=CARTESIAN_POINT('Ctrl Pts',(202.932545649898,98.1283167494464,334.030727003283));
#24728=CARTESIAN_POINT('Ctrl Pts',(201.638805561778,98.1710764119139,334.231275804564));
#24729=CARTESIAN_POINT('Ctrl Pts',(201.027285562879,98.1919728007889,334.452025495068));
#24730=CARTESIAN_POINT('Ctrl Pts',(199.904178929685,98.2317994170826,335.123860172382));
#24731=CARTESIAN_POINT('Ctrl Pts',(199.407541238451,98.2528991230827,335.57532779236));
#24732=CARTESIAN_POINT('Ctrl Pts',(198.631907392309,98.295647794643,336.629665876014));
#24733=CARTESIAN_POINT('Ctrl Pts',(198.353987917779,98.316559372242,337.217599990389));
#24734=CARTESIAN_POINT('Ctrl Pts',(198.031724659258,98.3564161178684,338.485695774884));
#24735=CARTESIAN_POINT('Ctrl Pts',(197.998002447511,98.3774524682769,339.155530828702));
#24736=CARTESIAN_POINT('Ctrl Pts',(198.191359714666,98.4201891897461,340.449772811658));
#24737=CARTESIAN_POINT('Ctrl Pts',(198.408927445719,98.4411168651635,341.062801411641));
#24738=CARTESIAN_POINT('Ctrl Pts',(199.074490349552,98.4810056885441,342.188898326382));
#24739=CARTESIAN_POINT('Ctrl Pts',(199.522508907796,98.5019752688356,342.687297558801));
#24740=CARTESIAN_POINT('Ctrl Pts',(200.571781851861,98.5446990005184,343.468736769743));
#24741=CARTESIAN_POINT('Ctrl Pts',(201.158440861306,98.5656437069934,343.75019947828));
#24742=CARTESIAN_POINT('Ctrl Pts',(202.424048234059,98.6055666358783,344.07945836568));
#24743=CARTESIAN_POINT('Ctrl Pts',(203.092608024152,98.6264660090367,344.117111082783));
#24744=CARTESIAN_POINT('Ctrl Pts',(204.387394029372,98.6691756252586,343.931960667624));
#24745=CARTESIAN_POINT('Ctrl Pts',(205.002125100582,98.690138315837,343.718037509402));
#24746=CARTESIAN_POINT('Ctrl Pts',(206.131614507215,98.7300974532906,343.059637825064));
#24747=CARTESIAN_POINT('Ctrl Pts',(206.632012430995,98.7509231883392,342.615543230054));
#24748=CARTESIAN_POINT('Ctrl Pts',(207.42003869431,98.7936174719612,341.572060645236));
#24749=CARTESIAN_POINT('Ctrl Pts',(207.705531099556,98.8145991142706,340.986879656359));
#24750=CARTESIAN_POINT('Ctrl Pts',(207.887254109002,98.8361536439949,340.306386204824));
#24751=CARTESIAN_POINT('Ctrl Pts',(207.901506963965,98.8379528132061,340.248933876262));
#24752=CARTESIAN_POINT('Ctrl Pts',(207.914727694784,98.8397376070391,340.191287620971));
#24753=CARTESIAN_POINT('Origin',(203.041252647846,100.739737607039,339.073593133701));
#24754=CARTESIAN_POINT('',(207.914727692943,99.9647376092732,340.191287628998));
#24755=CARTESIAN_POINT('',(207.914727694784,99.8397376070391,340.191287620971));
#24756=CARTESIAN_POINT('',(207.914727694784,100.739737607039,340.191287620971));
#24757=CARTESIAN_POINT('Ctrl Pts',(207.914727691102,99.9647376092732,340.191287637025));
#24758=CARTESIAN_POINT('Ctrl Pts',(207.772226000692,99.9454999333533,340.812636699557));
#24759=CARTESIAN_POINT('Ctrl Pts',(207.512177670137,99.9249116561356,341.401134030297));
#24760=CARTESIAN_POINT('Ctrl Pts',(206.767415734281,99.8822557941594,342.473938918684));
#24761=CARTESIAN_POINT('Ctrl Pts',(206.280052374215,99.8605969813808,342.94100626745));
#24762=CARTESIAN_POINT('Ctrl Pts',(205.172414462498,99.8209677950671,343.642066565408));
#24763=CARTESIAN_POINT('Ctrl Pts',(204.568303547233,99.8002965657112,343.877865874889));
#24764=CARTESIAN_POINT('Ctrl Pts',(203.278661492023,99.7574837781782,344.112457012639));
#24765=CARTESIAN_POINT('Ctrl Pts',(202.603858439339,99.735822425517,344.099054622666));
#24766=CARTESIAN_POINT('Ctrl Pts',(201.324683937858,99.6961755945932,343.813433082381));
#24767=CARTESIAN_POINT('Ctrl Pts',(200.730480054175,99.6755355963093,343.553898797219));
#24768=CARTESIAN_POINT('Ctrl Pts',(199.651737388951,99.632729958152,342.809574598577));
#24769=CARTESIAN_POINT('Ctrl Pts',(199.183395314978,99.6110659111106,342.323727313663));
#24770=CARTESIAN_POINT('Ctrl Pts',(198.479242320269,99.5714000791075,341.218502623156));
#24771=CARTESIAN_POINT('Ctrl Pts',(198.241680356331,99.5507934959721,340.615279102861));
#24772=CARTESIAN_POINT('Ctrl Pts',(198.003184949077,99.5079956229591,339.326759280724));
#24773=CARTESIAN_POINT('Ctrl Pts',(198.014458134513,99.4863287244055,338.652143518686));
#24774=CARTESIAN_POINT('Ctrl Pts',(198.295878414244,99.4466424476291,337.372453614684));
#24775=CARTESIAN_POINT('Ctrl Pts',(198.553391574092,99.4260715654506,336.777582057841));
#24776=CARTESIAN_POINT('Ctrl Pts',(199.293881381493,99.3832821245836,335.696721190546));
#24777=CARTESIAN_POINT('Ctrl Pts',(199.777959926478,99.3616122161077,335.226901158811));
#24778=CARTESIAN_POINT('Ctrl Pts',(200.880371479858,99.3219039609348,334.519154046494));
#24779=CARTESIAN_POINT('Ctrl Pts',(201.482563588122,99.3013711628205,334.279542718545));
#24780=CARTESIAN_POINT('Ctrl Pts',(202.76977183055,99.2585908761615,334.036512880947));
#24781=CARTESIAN_POINT('Ctrl Pts',(203.44416178828,99.2369177997395,334.045312525477));
#24782=CARTESIAN_POINT('Ctrl Pts',(204.724442646349,99.1971859403622,334.321850504282));
#24783=CARTESIAN_POINT('Ctrl Pts',(205.320089637049,99.1766937002196,334.577017428622));
#24784=CARTESIAN_POINT('Ctrl Pts',(206.403400096601,99.1339233488994,335.31305403556));
#24785=CARTESIAN_POINT('Ctrl Pts',(206.874927747583,99.1122469489044,335.79507416393));
#24786=CARTESIAN_POINT('Ctrl Pts',(207.586838848766,99.0724897656359,336.894214834667));
#24787=CARTESIAN_POINT('Ctrl Pts',(207.828825798982,99.0520406392946,337.49521178462));
#24788=CARTESIAN_POINT('Ctrl Pts',(208.077105239224,99.0092810676856,338.780890563379));
#24789=CARTESIAN_POINT('Ctrl Pts',(208.071170113211,98.9876011932843,339.455007960196));
#24790=CARTESIAN_POINT('Ctrl Pts',(207.927190449723,98.966454936529,340.135864050133));
#24791=CARTESIAN_POINT('Ctrl Pts',(207.921075822522,98.9655946046969,340.163607926315));
#24792=CARTESIAN_POINT('Ctrl Pts',(207.914727694784,98.9647376097703,340.191287620971));
#24793=CARTESIAN_POINT('Ctrl Pts',(207.914727694784,98.8397376070391,340.191287620971));
#24794=CARTESIAN_POINT('Ctrl Pts',(208.049234382686,98.8578959607898,339.604799099645));
#24795=CARTESIAN_POINT('Ctrl Pts',(208.076885361511,98.8772793791297,338.99831557964));
#24796=CARTESIAN_POINT('Ctrl Pts',(207.909025166348,98.9180229753005,337.761651286256));
#24797=CARTESIAN_POINT('Ctrl Pts',(207.699259005141,98.9390245453775,337.145011250203));
#24798=CARTESIAN_POINT('Ctrl Pts',(207.049003838244,98.9790626822083,336.011694015816));
#24799=CARTESIAN_POINT('Ctrl Pts',(206.609350999,98.999731041669,335.509040267232));
#24800=CARTESIAN_POINT('Ctrl Pts',(205.572458381145,99.0423906159896,334.713580437515));
#24801=CARTESIAN_POINT('Ctrl Pts',(204.98898562304,99.0634130911169,334.423528734006));
#24802=CARTESIAN_POINT('Ctrl Pts',(203.729493197537,99.1034941366792,334.077317783523));
#24803=CARTESIAN_POINT('Ctrl Pts',(203.064028612122,99.1240789539438,334.030183023473));
#24804=CARTESIAN_POINT('Ctrl Pts',(201.768052178728,99.1667189425487,334.195478139589));
#24805=CARTESIAN_POINT('Ctrl Pts',(201.149287222279,99.1877632930759,334.400525569592));
#24806=CARTESIAN_POINT('Ctrl Pts',(200.011677601723,99.2278895830345,335.041567981417));
#24807=CARTESIAN_POINT('Ctrl Pts',(199.506492864002,99.2483878268878,335.476221651959));
#24808=CARTESIAN_POINT('Ctrl Pts',(198.702695460361,99.2910065954628,336.505652435701));
#24809=CARTESIAN_POINT('Ctrl Pts',(198.40751551838,99.3120737756058,337.087157847669));
#24810=CARTESIAN_POINT('Ctrl Pts',(198.051185060294,99.3522476785371,338.342942483846));
#24811=CARTESIAN_POINT('Ctrl Pts',(197.998417906508,99.3726565343252,339.006556835035));
#24812=CARTESIAN_POINT('Ctrl Pts',(198.1518825264,99.4152523336181,340.303158655062));
#24813=CARTESIAN_POINT('Ctrl Pts',(198.351602925608,99.4363432712621,340.92426942185));
#24814=CARTESIAN_POINT('Ctrl Pts',(198.982284772655,99.476567175061,342.066658951876));
#24815=CARTESIAN_POINT('Ctrl Pts',(199.411348093172,99.4968840997243,342.57466469062));
#24816=CARTESIAN_POINT('Ctrl Pts',(200.432378756558,99.5394550628214,343.387749359463));
#24817=CARTESIAN_POINT('Ctrl Pts',(201.011627979659,99.5605706483865,343.688659209056));
#24818=CARTESIAN_POINT('Ctrl Pts',(202.263218809242,99.6008469448783,344.056296410767));
#24819=CARTESIAN_POINT('Ctrl Pts',(202.924764336384,99.621069725327,344.115332894066));
#24820=CARTESIAN_POINT('Ctrl Pts',(204.221990579288,99.6636138660953,343.975066633394));
#24821=CARTESIAN_POINT('Ctrl Pts',(204.845666986157,99.6847549405606,343.781322539685));
#24822=CARTESIAN_POINT('Ctrl Pts',(205.993337998062,99.7250860083536,343.162215832264));
#24823=CARTESIAN_POINT('Ctrl Pts',(206.504465036478,99.7452128223663,342.739358964637));
#24824=CARTESIAN_POINT('Ctrl Pts',(207.327815493964,99.78772803532,341.727722708046));
#24825=CARTESIAN_POINT('Ctrl Pts',(207.635079777938,99.8088953775479,341.151047887576));
#24826=CARTESIAN_POINT('Ctrl Pts',(207.858203404946,99.8325988852204,340.419266196908));
#24827=CARTESIAN_POINT('Ctrl Pts',(207.88849335847,99.8361959812164,340.305677004524));
#24828=CARTESIAN_POINT('Ctrl Pts',(207.914727694784,99.8397376070391,340.191287620971));
#24829=CARTESIAN_POINT('Origin',(203.041252647846,100.739737607039,339.073593133701));
#24830=CARTESIAN_POINT('',(204.158947135117,100.089737607039,334.200118086763));
#24831=CARTESIAN_POINT('Ctrl Pts',(207.914727694784,99.8397376070391,340.191287620971));
#24832=CARTESIAN_POINT('Ctrl Pts',(208.034767752977,99.8559429710617,339.667877838696));
#24833=CARTESIAN_POINT('Ctrl Pts',(208.069878022306,99.8731477517474,339.127777149765));
#24834=CARTESIAN_POINT('Ctrl Pts',(207.955567219792,99.9117971036651,337.94709393426));
#24835=CARTESIAN_POINT('Ctrl Pts',(207.768480675938,99.9329914172117,337.320640552275));
#24836=CARTESIAN_POINT('Ctrl Pts',(207.16221135957,99.9734390149761,336.167184155024));
#24837=CARTESIAN_POINT('Ctrl Pts',(206.746189859031,99.9933703048699,335.652631237103));
#24838=CARTESIAN_POINT('Ctrl Pts',(205.939101240561,100.027590364906,334.979846171942));
#24839=CARTESIAN_POINT('Ctrl Pts',(205.606479924445,100.040537817989,334.763616001554));
#24840=CARTESIAN_POINT('Ctrl Pts',(204.903851201034,100.065797691061,334.417277154942));
#24841=CARTESIAN_POINT('Ctrl Pts',(204.537074450298,100.078030353952,334.286838714568));
#24842=CARTESIAN_POINT('Ctrl Pts',(204.158947135116,100.089737607039,334.200118086763));
#24843=CARTESIAN_POINT('',(207.277649300794,100.089737607039,336.417855307993));
#24844=CARTESIAN_POINT('Origin',(203.041252647846,100.089737607039,339.073593133701));
#24845=CARTESIAN_POINT('Ctrl Pts',(207.277649300794,100.089737607039,336.417855307994));
#24846=CARTESIAN_POINT('Ctrl Pts',(207.62501622021,100.070001614885,336.971970266372));
#24847=CARTESIAN_POINT('Ctrl Pts',(207.860302304862,100.048852917176,337.588869716441));
#24848=CARTESIAN_POINT('Ctrl Pts',(208.080080674944,100.006125505448,338.878361907358));
#24849=CARTESIAN_POINT('Ctrl Pts',(208.062383836499,99.9849574354711,339.538574593748));
#24850=CARTESIAN_POINT('Ctrl Pts',(207.916957879617,99.9650397665077,340.181529749979));
#24851=CARTESIAN_POINT('Ctrl Pts',(207.91584640822,99.9648886356732,340.186409703085));
#24852=CARTESIAN_POINT('Ctrl Pts',(207.914727691102,99.9647376092732,340.191287637025));
#24853=CARTESIAN_POINT('Origin',(203.041252647846,100.739737607039,339.073593133701));
#24854=CARTESIAN_POINT('',(212.788202741722,85.7397376070391,341.308982108241));
#24855=CARTESIAN_POINT('Origin',(203.041252647846,85.7397376070391,339.073593133701));
#24856=CARTESIAN_POINT('',(212.788202741722,70.2397376070391,341.308982108241));
#24857=CARTESIAN_POINT('',(212.788202741722,100.739737607039,341.308982108241));
#24858=CARTESIAN_POINT('',(205.276641622387,70.2397376070391,329.326643039825));
#24859=CARTESIAN_POINT('Origin',(203.041252647846,70.2397376070391,339.073593133701));
#24860=CARTESIAN_POINT('',(193.294302553971,70.2397376070391,336.83820415916));
#24861=CARTESIAN_POINT('Origin',(203.041252647846,70.2397376070391,339.073593133701));
#24862=CARTESIAN_POINT('',(200.805863673306,70.2397376070391,348.820543227576));
#24863=CARTESIAN_POINT('Origin',(203.041252647846,70.2397376070391,339.073593133701));
#24864=CARTESIAN_POINT('Origin',(203.041252647846,70.2397376070391,339.073593133701));
#24865=CARTESIAN_POINT('Origin',(216.141286203533,40.2397376070391,326.688556967428));
#24866=CARTESIAN_POINT('',(210.105735972273,35.2397376070391,353.005322220892));
#24867=CARTESIAN_POINT('Origin',(210.105735972273,40.2397376070391,353.005322220892));
#24868=CARTESIAN_POINT('',(209.435119279911,35.2397376070391,355.929407249055));
#24869=CARTESIAN_POINT('',(216.141286203533,35.2397376070391,326.688556967428));
#24870=CARTESIAN_POINT('Origin',(209.435119279911,40.2397376070391,355.929407249055));
#24871=CARTESIAN_POINT('Origin',(216.141286203533,40.2397376070391,326.688556967428));
#24872=CARTESIAN_POINT('',(216.141286203533,35.2397376070391,326.688556967428));
#24873=CARTESIAN_POINT('Origin',(216.141286203533,40.2397376070391,326.688556967428));
#24874=CARTESIAN_POINT('',(215.470669511171,35.2397376070391,329.612641995591));
#24875=CARTESIAN_POINT('',(216.141286203533,35.2397376070391,326.688556967428));
#24876=CARTESIAN_POINT('Origin',(215.470669511171,40.2397376070391,329.612641995591));
#24877=CARTESIAN_POINT('Origin',(203.041252647846,100.739737607039,339.073593133701));
#24878=CARTESIAN_POINT('',(198.322260569661,100.248231256093,337.991328141994));
#24879=CARTESIAN_POINT('Ctrl Pts',(204.158947135117,100.089737607039,334.200118086763));
#24880=CARTESIAN_POINT('Ctrl Pts',(203.567986347669,100.101286651919,334.076434599289));
#24881=CARTESIAN_POINT('Ctrl Pts',(203.076964148285,100.11133952839,334.083193431931));
#24882=CARTESIAN_POINT('Ctrl Pts',(202.269604552341,100.128117897055,334.15059440257));
#24883=CARTESIAN_POINT('Ctrl Pts',(201.816482456597,100.137815372571,334.253306792782));
#24884=CARTESIAN_POINT('Ctrl Pts',(200.812021118434,100.159974179144,334.634292946593));
#24885=CARTESIAN_POINT('Ctrl Pts',(200.244344607109,100.17228394124,334.970269554068));
#24886=CARTESIAN_POINT('Ctrl Pts',(199.282907777807,100.199611537441,335.881659458326));
#24887=CARTESIAN_POINT('Ctrl Pts',(198.91269334307,100.213147705628,336.402192829191));
#24888=CARTESIAN_POINT('Ctrl Pts',(198.510734686059,100.233619853094,337.29194862115));
#24889=CARTESIAN_POINT('Ctrl Pts',(198.397399007679,100.240963808763,337.631191678964));
#24890=CARTESIAN_POINT('Ctrl Pts',(198.322260569661,100.248231256093,337.991328141994));
#24891=CARTESIAN_POINT('',(198.801329357011,100.739737607039,338.101198929776));
#24892=CARTESIAN_POINT('',(198.801329357011,100.739737607039,338.101198929776));
#24893=CARTESIAN_POINT('Origin',(203.041252647846,100.739737607039,339.073593133701));
#24894=CARTESIAN_POINT('',(207.107563775619,100.631003482039,337.244543159099));
#24895=CARTESIAN_POINT('Ctrl Pts',(198.322260569661,100.248231256093,337.991328141994));
#24896=CARTESIAN_POINT('Ctrl Pts',(198.265865587261,100.253685822026,338.261627738713));
#24897=CARTESIAN_POINT('Ctrl Pts',(198.231285693129,100.259483012085,338.543751260379));
#24898=CARTESIAN_POINT('Ctrl Pts',(198.205299560629,100.278651810169,339.458060951051));
#24899=CARTESIAN_POINT('Ctrl Pts',(198.308913933128,100.292192634244,340.07813647236));
#24900=CARTESIAN_POINT('Ctrl Pts',(198.735959685609,100.318070364889,341.214213314114));
#24901=CARTESIAN_POINT('Ctrl Pts',(199.058786882686,100.33037409878,341.76423347003));
#24902=CARTESIAN_POINT('Ctrl Pts',(199.726641142822,100.351123698728,342.473696291465));
#24903=CARTESIAN_POINT('Ctrl Pts',(199.956597002958,100.357752877431,342.674907245237));
#24904=CARTESIAN_POINT('Ctrl Pts',(200.684813343231,100.377376238089,343.197053078148));
#24905=CARTESIAN_POINT('Ctrl Pts',(201.22575207331,100.390328845839,343.448271766013));
#24906=CARTESIAN_POINT('Ctrl Pts',(202.379327369579,100.415014798707,343.739752840505));
#24907=CARTESIAN_POINT('Ctrl Pts',(202.976464577814,100.427516491142,343.773223792695));
#24908=CARTESIAN_POINT('Ctrl Pts',(204.172185811973,100.454347635149,343.610258087121));
#24909=CARTESIAN_POINT('Ctrl Pts',(204.755653114925,100.468015172787,343.408876554908));
#24910=CARTESIAN_POINT('Ctrl Pts',(205.542558502781,100.487313364515,342.948631399366));
#24911=CARTESIAN_POINT('Ctrl Pts',(205.786240387277,100.493517003125,342.772350110457));
#24912=CARTESIAN_POINT('Ctrl Pts',(206.443763515596,100.512731222331,342.189020750292));
#24913=CARTESIAN_POINT('Ctrl Pts',(206.799360258044,100.525914732775,341.726717280771));
#24914=CARTESIAN_POINT('Ctrl Pts',(207.328428666458,100.552463745409,340.675326282134));
#24915=CARTESIAN_POINT('Ctrl Pts',(207.491421017174,100.564937188876,340.089059350026));
#24916=CARTESIAN_POINT('Ctrl Pts',(207.560618501709,100.586849760216,339.103391640685));
#24917=CARTESIAN_POINT('Ctrl Pts',(207.537661983056,100.595710021862,338.715638501893));
#24918=CARTESIAN_POINT('Ctrl Pts',(207.393266348567,100.613507459,337.958136842933));
#24919=CARTESIAN_POINT('Ctrl Pts',(207.273057797548,100.622370230913,337.591420948307));
#24920=CARTESIAN_POINT('Ctrl Pts',(207.107563775619,100.631003482039,337.244543159099));
#24921=CARTESIAN_POINT('',(201.212202673244,100.631003482039,335.007282005928));
#24922=CARTESIAN_POINT('Origin',(203.041252647846,100.631003482039,339.073593133701));
#24923=CARTESIAN_POINT('Ctrl Pts',(201.212202673245,100.631003482039,335.007282005928));
#24924=CARTESIAN_POINT('Ctrl Pts',(201.692997247517,100.585063473448,334.740644369554));
#24925=CARTESIAN_POINT('Ctrl Pts',(202.2181597904,100.538067764303,334.563560685677));
#24926=CARTESIAN_POINT('Ctrl Pts',(203.34458799318,100.443271815276,334.400105891955));
#24927=CARTESIAN_POINT('Ctrl Pts',(203.930685093604,100.399102406969,334.431026796414));
#24928=CARTESIAN_POINT('Ctrl Pts',(205.043083613764,100.310330549729,334.698222656967));
#24929=CARTESIAN_POINT('Ctrl Pts',(205.558128812846,100.265685149075,334.920866681284));
#24930=CARTESIAN_POINT('Ctrl Pts',(206.260185161977,100.199312659861,335.381164329575));
#24931=CARTESIAN_POINT('Ctrl Pts',(206.482421957023,100.177253987256,335.556461106809));
#24932=CARTESIAN_POINT('Ctrl Pts',(206.970346125787,100.126107413338,336.015937249671));
#24933=CARTESIAN_POINT('Ctrl Pts',(207.163692240569,100.103490234527,336.261964855603));
#24934=CARTESIAN_POINT('Ctrl Pts',(207.277649300794,100.089737607039,336.417855307993));
#24935=CARTESIAN_POINT('Origin',(225.888236297409,70.2397376070391,328.923945941969));
#24936=CARTESIAN_POINT('',(220.299763861057,70.2397376070391,353.291321176658));
#24937=CARTESIAN_POINT('',(224.770541810138,70.2397376070391,333.797420988906));
#24938=CARTESIAN_POINT('',(225.888236297409,70.2397376070391,328.923945941969));
#24939=CARTESIAN_POINT('',(224.770541810138,70.2397376070391,333.797420988906));
#24940=CARTESIAN_POINT('',(220.299763861057,70.2397376070391,353.291321176658));
#24941=CARTESIAN_POINT('Origin',(225.888236297409,70.2397376070391,328.923945941969));
#24942=CARTESIAN_POINT('',(191.05891357943,70.2397376070391,346.585154253036));
#24943=CARTESIAN_POINT('',(196.647386015782,70.2397376070391,322.217779018347));
#24944=CARTESIAN_POINT('',(220.299763861057,70.2397376070391,353.291321176658));
#24945=CARTESIAN_POINT('Origin',(225.217619605046,31.2397376070391,331.848030970131));
#24946=CARTESIAN_POINT('',(225.145860085501,65.2397376070391,331.831573469348));
#24947=CARTESIAN_POINT('',(224.236987121615,39.9086604301851,331.623130358101));
#24948=CARTESIAN_POINT('',(223.927696189104,31.2884540946096,331.552196831839));
#24949=CARTESIAN_POINT('',(196.724771172371,65.2397376070391,325.313412589385));
#24950=CARTESIAN_POINT('',(195.97676932342,65.2397376070391,325.14186404651));
#24951=CARTESIAN_POINT('',(207.280643844697,37.0155488911437,327.734321813409));
#24952=CARTESIAN_POINT('',(211.465570642183,25.8259327067678,328.694102989291));
#24953=CARTESIAN_POINT('Origin',(215.470669511171,40.2397376070391,329.612641995591));
#24954=CARTESIAN_POINT('Origin',(225.888236297409,31.2397376070391,328.923945941969));
#24955=CARTESIAN_POINT('',(207.951260537059,37.0155488911437,324.810236785247));
#24956=CARTESIAN_POINT('',(197.395387864733,65.2397376070391,322.389327561222));
#24957=CARTESIAN_POINT('',(207.951260537059,37.0155488911437,324.810236785247));
#24958=CARTESIAN_POINT('',(225.816476777863,65.2397376070391,328.907488441185));
#24959=CARTESIAN_POINT('',(225.888236297409,65.2397376070391,328.923945941969));
#24960=CARTESIAN_POINT('',(224.907603813977,39.9086604301851,328.699045329938));
#24961=CARTESIAN_POINT('',(225.888236297409,67.2397376070391,328.923945941969));
#24962=CARTESIAN_POINT('Origin',(216.141286203533,40.2397376070391,326.688556967428));
#24963=CARTESIAN_POINT('Origin',(225.888236297409,70.2397376070391,328.923945941969));
#24964=CARTESIAN_POINT('',(195.529691528511,70.2397376070391,327.091254065285));
#24965=CARTESIAN_POINT('',(224.770541810138,70.2397376070391,333.797420988906));
#24966=CARTESIAN_POINT('',(196.647386015782,70.2397376070391,322.217779018347));
#24967=CARTESIAN_POINT('Origin',(219.182069373787,31.2397376070391,358.164796223596));
#24968=CARTESIAN_POINT('',(219.110309854242,65.2397376070391,358.148338722812));
#24969=CARTESIAN_POINT('',(218.201436890355,39.9086604301851,357.939895611565));
#24970=CARTESIAN_POINT('',(219.182069373787,67.2397376070391,358.164796223596));
#24971=CARTESIAN_POINT('',(190.689220941112,65.2397376070391,351.630177842849));
#24972=CARTESIAN_POINT('',(219.182069373787,65.2397376070391,358.164796223596));
#24973=CARTESIAN_POINT('',(201.245093613437,37.0155488911437,354.051087066874));
#24974=CARTESIAN_POINT('',(201.245093613437,37.0155488911437,354.051087066874));
#24975=CARTESIAN_POINT('Origin',(209.435119279911,40.2397376070391,355.929407249055));
#24976=CARTESIAN_POINT('Origin',(219.852686066149,31.2397376070391,355.240711195433));
#24977=CARTESIAN_POINT('',(191.359837633474,65.2397376070391,348.706092814686));
#24978=CARTESIAN_POINT('',(201.915710305799,37.0155488911437,351.127002038711));
#24979=CARTESIAN_POINT('',(206.100637103286,25.8259327067678,352.086783214593));
#24980=CARTESIAN_POINT('',(219.780926546604,65.2397376070391,355.224253694649));
#24981=CARTESIAN_POINT('',(219.852686066149,65.2397376070391,355.240711195433));
#24982=CARTESIAN_POINT('',(218.872053582717,39.9086604301851,355.015810583403));
#24983=CARTESIAN_POINT('',(218.562762650207,31.2884540946096,354.944877057141));
#24984=CARTESIAN_POINT('Origin',(210.105735972273,40.2397376070391,353.005322220892));
#24985=CARTESIAN_POINT('Origin',(225.217619605046,67.2397376070391,331.848030970131));
#24986=CARTESIAN_POINT('',(224.770541810138,67.2397376070391,333.797420988906));
#24987=CARTESIAN_POINT('',(220.299763861057,67.2397376070391,353.291321176658));
#24988=CARTESIAN_POINT('',(225.217619605046,67.2397376070391,331.848030970131));
#24989=CARTESIAN_POINT('',(191.05891357943,67.2397376070391,346.585154253036));
#24990=CARTESIAN_POINT('',(191.05891357943,67.2397376070391,346.585154253036));
#24991=CARTESIAN_POINT('',(195.529691528511,67.2397376070391,327.091254065285));
#24992=CARTESIAN_POINT('',(195.97676932342,67.2397376070391,325.14186404651));
#24993=CARTESIAN_POINT('',(224.770541810138,67.2397376070391,333.797420988906));
#24994=CARTESIAN_POINT('Origin',(222.535152835598,31.2397376070391,343.544371082782));
#24995=CARTESIAN_POINT('',(225.794925728488,67.2397376070391,329.330807328892));
#24996=CARTESIAN_POINT('',(225.888236297409,67.2397376070391,328.923945941969));
#24997=CARTESIAN_POINT('Origin',(224.770541810138,65.2397376070391,333.797420988906));
#24998=CARTESIAN_POINT('',(219.275379942707,67.2397376070391,357.757934836672));
#24999=CARTESIAN_POINT('Origin',(220.299763861057,65.2397376070391,353.291321176658));
#25000=CARTESIAN_POINT('',(222.535152835598,67.2397376070391,343.544371082782));
#25001=CARTESIAN_POINT('Origin',(193.294302553971,31.2397376070391,336.83820415916));
#25002=CARTESIAN_POINT('',(196.554075446862,67.2397376070391,322.62464040527));
#25003=CARTESIAN_POINT('Origin',(195.529691528511,65.2397376070391,327.091254065285));
#25004=CARTESIAN_POINT('',(196.647386015782,67.2397376070391,322.217779018347));
#25005=CARTESIAN_POINT('',(190.03452966108,67.2397376070391,351.05176791305));
#25006=CARTESIAN_POINT('',(193.294302553971,67.2397376070391,336.83820415916));
#25007=CARTESIAN_POINT('Origin',(191.05891357943,65.2397376070391,346.585154253036));
#25008=CARTESIAN_POINT('Origin',(207.951260537059,37.0155488911437,324.810236785247));
#25009=CARTESIAN_POINT('Origin',(191.806915428346,65.2397376070675,346.756702796012));
#25010=CARTESIAN_POINT('Origin',(191.806915428382,65.2397376070398,346.756702795912));
#25011=CARTESIAN_POINT('',(207.951260537059,37.0155488911437,324.810236785247));
#25012=CARTESIAN_POINT('Origin',(225.888236297409,67.2397376070391,328.923945941969));
#25013=CARTESIAN_POINT('Origin',(220.228004341512,65.2397376070391,353.274863675874));
#25014=CARTESIAN_POINT('',(224.907603813977,39.9086604301851,328.699045329938));
#25015=CARTESIAN_POINT('Origin',(220.228004341512,65.2397376070392,353.274863675875));
#25016=CARTESIAN_POINT('Origin',(216.141286203533,40.2397376070391,326.688556967428));
#25017=CARTESIAN_POINT('Origin',(216.141286203533,40.2397376070391,326.688556967428));
#25018=CARTESIAN_POINT('',(207.951260537059,37.0155488911437,324.810236785247));
#25019=CARTESIAN_POINT('',(224.907603813977,39.9086604301851,328.699045329938));
#25020=CARTESIAN_POINT('Origin',(225.888236297409,67.2397376070391,328.923945941969));
#25021=CARTESIAN_POINT('Origin',(224.698782290593,65.2397376070391,333.780963488123));
#25022=CARTESIAN_POINT('Origin',(224.698782290594,65.2397376070431,333.780963488119));
#25023=CARTESIAN_POINT('Origin',(207.951260537059,37.0155488911437,324.810236785247));
#25024=CARTESIAN_POINT('Origin',(196.27769337772,65.2397376073992,327.262802606412));
#25025=CARTESIAN_POINT('Origin',(196.277693377464,65.2397376070354,327.262802608164));
#25026=CARTESIAN_POINT('Origin',(193.294302553971,85.7397376070391,336.83820415916));
#25027=CARTESIAN_POINT('Origin',(198.167777600909,100.739737607039,337.955898646431));
#25028=CARTESIAN_POINT('Origin',(204.098450146653,87.9334876077219,334.46390266032));
#25029=CARTESIAN_POINT('',(204.098450146653,87.9334876077219,334.46390266032));
#25030=CARTESIAN_POINT('',(204.098450146653,87.3709876090875,334.46390266032));
#25031=CARTESIAN_POINT('Ctrl Pts',(204.03795315819,101.777237608405,334.727687233877));
#25032=CARTESIAN_POINT('Ctrl Pts',(205.838086322694,101.714737608405,335.140534102886));
#25033=CARTESIAN_POINT('Ctrl Pts',(206.819045869686,101.652237608405,336.705347291213));
#25034=CARTESIAN_POINT('Ctrl Pts',(207.800005416678,101.589737608405,338.27016047954));
#25035=CARTESIAN_POINT('Ctrl Pts',(207.38715854767,101.527237608405,340.070293644044));
#25036=CARTESIAN_POINT('Ctrl Pts',(206.974311678662,101.464737608405,341.870426808548));
#25037=CARTESIAN_POINT('Ctrl Pts',(205.409498490334,101.402237608405,342.851386355541));
#25038=CARTESIAN_POINT('Ctrl Pts',(203.844685302007,101.339737608405,343.832345902533));
#25039=CARTESIAN_POINT('Ctrl Pts',(202.044552137503,101.277237608405,343.419499033524));
#25040=CARTESIAN_POINT('Ctrl Pts',(200.244418972999,101.214737608405,343.006652164516));
#25041=CARTESIAN_POINT('Ctrl Pts',(199.263459426007,101.152237608405,341.441838976189));
#25042=CARTESIAN_POINT('Ctrl Pts',(198.282499879015,101.089737608405,339.877025787862));
#25043=CARTESIAN_POINT('Ctrl Pts',(198.695346748023,101.027237608405,338.076892623358));
#25044=CARTESIAN_POINT('Ctrl Pts',(199.108193617031,100.964737608405,336.276759458854));
#25045=CARTESIAN_POINT('Ctrl Pts',(200.673006805358,100.902237608405,335.295799911861));
#25046=CARTESIAN_POINT('Ctrl Pts',(202.237819993686,100.839737608405,334.314840364869));
#25047=CARTESIAN_POINT('Ctrl Pts',(204.03795315819,100.777237608405,334.727687233877));
#25048=CARTESIAN_POINT('Ctrl Pts',(205.838086322694,100.714737608405,335.140534102886));
#25049=CARTESIAN_POINT('Ctrl Pts',(206.819045869686,100.652237608405,336.705347291213));
#25050=CARTESIAN_POINT('Ctrl Pts',(207.800005416678,100.589737608405,338.27016047954));
#25051=CARTESIAN_POINT('Ctrl Pts',(207.38715854767,100.527237608405,340.070293644044));
#25052=CARTESIAN_POINT('Ctrl Pts',(206.974311678662,100.464737608405,341.870426808548));
#25053=CARTESIAN_POINT('Ctrl Pts',(205.409498490334,100.402237608405,342.851386355541));
#25054=CARTESIAN_POINT('Ctrl Pts',(203.844685302007,100.339737608405,343.832345902533));
#25055=CARTESIAN_POINT('Ctrl Pts',(202.044552137503,100.277237608405,343.419499033524));
#25056=CARTESIAN_POINT('Ctrl Pts',(200.244418972999,100.214737608405,343.006652164516));
#25057=CARTESIAN_POINT('Ctrl Pts',(199.263459426007,100.152237608405,341.441838976189));
#25058=CARTESIAN_POINT('Ctrl Pts',(198.282499879015,100.089737608405,339.877025787862));
#25059=CARTESIAN_POINT('Ctrl Pts',(198.695346748023,100.027237608405,338.076892623358));
#25060=CARTESIAN_POINT('Ctrl Pts',(199.108193617031,99.9647376084047,336.276759458854));
#25061=CARTESIAN_POINT('Ctrl Pts',(200.673006805358,99.9022376084047,335.295799911861));
#25062=CARTESIAN_POINT('Ctrl Pts',(202.237819993686,99.8397376084047,334.314840364869));
#25063=CARTESIAN_POINT('Ctrl Pts',(204.03795315819,99.7772376084047,334.727687233877));
#25064=CARTESIAN_POINT('Ctrl Pts',(205.838086322694,99.7147376084047,335.140534102886));
#25065=CARTESIAN_POINT('Ctrl Pts',(206.819045869686,99.6522376084047,336.705347291213));
#25066=CARTESIAN_POINT('Ctrl Pts',(207.800005416678,99.5897376084047,338.27016047954));
#25067=CARTESIAN_POINT('Ctrl Pts',(207.38715854767,99.5272376084047,340.070293644044));
#25068=CARTESIAN_POINT('Ctrl Pts',(206.974311678662,99.4647376084047,341.870426808548));
#25069=CARTESIAN_POINT('Ctrl Pts',(205.409498490334,99.4022376084047,342.851386355541));
#25070=CARTESIAN_POINT('Ctrl Pts',(203.844685302007,99.3397376084047,343.832345902533));
#25071=CARTESIAN_POINT('Ctrl Pts',(202.044552137503,99.2772376084047,343.419499033524));
#25072=CARTESIAN_POINT('Ctrl Pts',(200.244418972999,99.2147376084047,343.006652164516));
#25073=CARTESIAN_POINT('Ctrl Pts',(199.263459426007,99.1522376084047,341.441838976189));
#25074=CARTESIAN_POINT('Ctrl Pts',(198.282499879015,99.0897376084047,339.877025787862));
#25075=CARTESIAN_POINT('Ctrl Pts',(198.695346748023,99.0272376084047,338.076892623358));
#25076=CARTESIAN_POINT('Ctrl Pts',(199.108193617031,98.9647376084047,336.276759458854));
#25077=CARTESIAN_POINT('Ctrl Pts',(200.673006805358,98.9022376084047,335.295799911861));
#25078=CARTESIAN_POINT('Ctrl Pts',(202.237819993686,98.8397376084047,334.314840364869));
#25079=CARTESIAN_POINT('Ctrl Pts',(204.03795315819,98.7772376084047,334.727687233877));
#25080=CARTESIAN_POINT('Ctrl Pts',(205.838086322694,98.7147376084047,335.140534102886));
#25081=CARTESIAN_POINT('Ctrl Pts',(206.819045869686,98.6522376084047,336.705347291213));
#25082=CARTESIAN_POINT('Ctrl Pts',(207.800005416678,98.5897376084047,338.27016047954));
#25083=CARTESIAN_POINT('Ctrl Pts',(207.38715854767,98.5272376084047,340.070293644044));
#25084=CARTESIAN_POINT('Ctrl Pts',(206.974311678662,98.4647376084047,341.870426808548));
#25085=CARTESIAN_POINT('Ctrl Pts',(205.409498490334,98.4022376084047,342.851386355541));
#25086=CARTESIAN_POINT('Ctrl Pts',(203.844685302007,98.3397376084047,343.832345902533));
#25087=CARTESIAN_POINT('Ctrl Pts',(202.044552137503,98.2772376084047,343.419499033524));
#25088=CARTESIAN_POINT('Ctrl Pts',(200.244418972999,98.2147376084047,343.006652164516));
#25089=CARTESIAN_POINT('Ctrl Pts',(199.263459426007,98.1522376084047,341.441838976189));
#25090=CARTESIAN_POINT('Ctrl Pts',(198.282499879015,98.0897376084047,339.877025787862));
#25091=CARTESIAN_POINT('Ctrl Pts',(198.695346748023,98.0272376084047,338.076892623358));
#25092=CARTESIAN_POINT('Ctrl Pts',(199.108193617031,97.9647376084047,336.276759458854));
#25093=CARTESIAN_POINT('Ctrl Pts',(200.673006805358,97.9022376084047,335.295799911861));
#25094=CARTESIAN_POINT('Ctrl Pts',(202.237819993686,97.8397376084047,334.314840364869));
#25095=CARTESIAN_POINT('Ctrl Pts',(204.03795315819,97.7772376084047,334.727687233877));
#25096=CARTESIAN_POINT('Ctrl Pts',(205.838086322694,97.7147376084047,335.140534102886));
#25097=CARTESIAN_POINT('Ctrl Pts',(206.819045869686,97.6522376084047,336.705347291213));
#25098=CARTESIAN_POINT('Ctrl Pts',(207.800005416678,97.5897376084047,338.27016047954));
#25099=CARTESIAN_POINT('Ctrl Pts',(207.38715854767,97.5272376084047,340.070293644044));
#25100=CARTESIAN_POINT('Ctrl Pts',(206.974311678662,97.4647376084047,341.870426808548));
#25101=CARTESIAN_POINT('Ctrl Pts',(205.409498490334,97.4022376084047,342.851386355541));
#25102=CARTESIAN_POINT('Ctrl Pts',(203.844685302007,97.3397376084047,343.832345902533));
#25103=CARTESIAN_POINT('Ctrl Pts',(202.044552137503,97.2772376084047,343.419499033524));
#25104=CARTESIAN_POINT('Ctrl Pts',(200.244418972999,97.2147376084047,343.006652164516));
#25105=CARTESIAN_POINT('Ctrl Pts',(199.263459426007,97.1522376084047,341.441838976189));
#25106=CARTESIAN_POINT('Ctrl Pts',(198.282499879015,97.0897376084047,339.877025787862));
#25107=CARTESIAN_POINT('Ctrl Pts',(198.695346748023,97.0272376084047,338.076892623358));
#25108=CARTESIAN_POINT('Ctrl Pts',(199.108193617031,96.9647376084047,336.276759458854));
#25109=CARTESIAN_POINT('Ctrl Pts',(200.673006805358,96.9022376084047,335.295799911861));
#25110=CARTESIAN_POINT('Ctrl Pts',(202.237819993686,96.8397376084047,334.314840364869));
#25111=CARTESIAN_POINT('Ctrl Pts',(204.03795315819,96.7772376084047,334.727687233877));
#25112=CARTESIAN_POINT('Ctrl Pts',(205.838086322694,96.7147376084047,335.140534102886));
#25113=CARTESIAN_POINT('Ctrl Pts',(206.819045869686,96.6522376084047,336.705347291213));
#25114=CARTESIAN_POINT('Ctrl Pts',(207.800005416678,96.5897376084047,338.27016047954));
#25115=CARTESIAN_POINT('Ctrl Pts',(207.38715854767,96.5272376084047,340.070293644044));
#25116=CARTESIAN_POINT('Ctrl Pts',(206.974311678662,96.4647376084047,341.870426808548));
#25117=CARTESIAN_POINT('Ctrl Pts',(205.409498490334,96.4022376084047,342.851386355541));
#25118=CARTESIAN_POINT('Ctrl Pts',(203.844685302007,96.3397376084047,343.832345902533));
#25119=CARTESIAN_POINT('Ctrl Pts',(202.044552137503,96.2772376084047,343.419499033524));
#25120=CARTESIAN_POINT('Ctrl Pts',(200.244418972999,96.2147376084047,343.006652164516));
#25121=CARTESIAN_POINT('Ctrl Pts',(199.263459426007,96.1522376084047,341.441838976189));
#25122=CARTESIAN_POINT('Ctrl Pts',(198.282499879015,96.0897376084047,339.877025787862));
#25123=CARTESIAN_POINT('Ctrl Pts',(198.695346748023,96.0272376084047,338.076892623358));
#25124=CARTESIAN_POINT('Ctrl Pts',(199.108193617031,95.9647376084047,336.276759458854));
#25125=CARTESIAN_POINT('Ctrl Pts',(200.673006805358,95.9022376084047,335.295799911861));
#25126=CARTESIAN_POINT('Ctrl Pts',(202.237819993686,95.8397376084047,334.314840364869));
#25127=CARTESIAN_POINT('Ctrl Pts',(204.03795315819,95.7772376084047,334.727687233877));
#25128=CARTESIAN_POINT('Ctrl Pts',(205.838086322694,95.7147376084047,335.140534102886));
#25129=CARTESIAN_POINT('Ctrl Pts',(206.819045869686,95.6522376084047,336.705347291213));
#25130=CARTESIAN_POINT('Ctrl Pts',(207.800005416678,95.5897376084047,338.27016047954));
#25131=CARTESIAN_POINT('Ctrl Pts',(207.38715854767,95.5272376084047,340.070293644044));
#25132=CARTESIAN_POINT('Ctrl Pts',(206.974311678662,95.4647376084047,341.870426808548));
#25133=CARTESIAN_POINT('Ctrl Pts',(205.409498490334,95.4022376084047,342.851386355541));
#25134=CARTESIAN_POINT('Ctrl Pts',(203.844685302007,95.3397376084047,343.832345902533));
#25135=CARTESIAN_POINT('Ctrl Pts',(202.044552137503,95.2772376084047,343.419499033524));
#25136=CARTESIAN_POINT('Ctrl Pts',(200.244418972999,95.2147376084047,343.006652164516));
#25137=CARTESIAN_POINT('Ctrl Pts',(199.263459426007,95.1522376084047,341.441838976189));
#25138=CARTESIAN_POINT('Ctrl Pts',(198.282499879015,95.0897376084047,339.877025787862));
#25139=CARTESIAN_POINT('Ctrl Pts',(198.695346748023,95.0272376084047,338.076892623358));
#25140=CARTESIAN_POINT('Ctrl Pts',(199.108193617031,94.9647376084047,336.276759458854));
#25141=CARTESIAN_POINT('Ctrl Pts',(200.673006805358,94.9022376084047,335.295799911861));
#25142=CARTESIAN_POINT('Ctrl Pts',(202.237819993686,94.8397376084047,334.314840364869));
#25143=CARTESIAN_POINT('Ctrl Pts',(204.03795315819,94.7772376084047,334.727687233877));
#25144=CARTESIAN_POINT('Ctrl Pts',(205.838086322694,94.7147376084047,335.140534102886));
#25145=CARTESIAN_POINT('Ctrl Pts',(206.819045869686,94.6522376084047,336.705347291213));
#25146=CARTESIAN_POINT('Ctrl Pts',(207.800005416678,94.5897376084047,338.27016047954));
#25147=CARTESIAN_POINT('Ctrl Pts',(207.38715854767,94.5272376084047,340.070293644044));
#25148=CARTESIAN_POINT('Ctrl Pts',(206.974311678662,94.4647376084047,341.870426808548));
#25149=CARTESIAN_POINT('Ctrl Pts',(205.409498490334,94.4022376084047,342.851386355541));
#25150=CARTESIAN_POINT('Ctrl Pts',(203.844685302007,94.3397376084047,343.832345902533));
#25151=CARTESIAN_POINT('Ctrl Pts',(202.044552137503,94.2772376084047,343.419499033524));
#25152=CARTESIAN_POINT('Ctrl Pts',(200.244418972999,94.2147376084047,343.006652164516));
#25153=CARTESIAN_POINT('Ctrl Pts',(199.263459426007,94.1522376084047,341.441838976189));
#25154=CARTESIAN_POINT('Ctrl Pts',(198.282499879015,94.0897376084047,339.877025787862));
#25155=CARTESIAN_POINT('Ctrl Pts',(198.695346748023,94.0272376084047,338.076892623358));
#25156=CARTESIAN_POINT('Ctrl Pts',(199.108193617031,93.9647376084047,336.276759458854));
#25157=CARTESIAN_POINT('Ctrl Pts',(200.673006805358,93.9022376084047,335.295799911861));
#25158=CARTESIAN_POINT('Ctrl Pts',(202.237819993686,93.8397376084047,334.314840364869));
#25159=CARTESIAN_POINT('Ctrl Pts',(204.03795315819,93.7772376084047,334.727687233877));
#25160=CARTESIAN_POINT('Ctrl Pts',(205.838086322694,93.7147376084047,335.140534102886));
#25161=CARTESIAN_POINT('Ctrl Pts',(206.819045869686,93.6522376084047,336.705347291213));
#25162=CARTESIAN_POINT('Ctrl Pts',(207.800005416678,93.5897376084047,338.27016047954));
#25163=CARTESIAN_POINT('Ctrl Pts',(207.38715854767,93.5272376084047,340.070293644044));
#25164=CARTESIAN_POINT('Ctrl Pts',(206.974311678662,93.4647376084047,341.870426808548));
#25165=CARTESIAN_POINT('Ctrl Pts',(205.409498490334,93.4022376084047,342.851386355541));
#25166=CARTESIAN_POINT('Ctrl Pts',(203.844685302007,93.3397376084047,343.832345902533));
#25167=CARTESIAN_POINT('Ctrl Pts',(202.044552137503,93.2772376084047,343.419499033524));
#25168=CARTESIAN_POINT('Ctrl Pts',(200.244418972999,93.2147376084047,343.006652164516));
#25169=CARTESIAN_POINT('Ctrl Pts',(199.263459426007,93.1522376084047,341.441838976189));
#25170=CARTESIAN_POINT('Ctrl Pts',(198.282499879015,93.0897376084047,339.877025787862));
#25171=CARTESIAN_POINT('Ctrl Pts',(198.695346748023,93.0272376084047,338.076892623358));
#25172=CARTESIAN_POINT('Ctrl Pts',(199.108193617031,92.9647376084047,336.276759458854));
#25173=CARTESIAN_POINT('Ctrl Pts',(200.673006805358,92.9022376084047,335.295799911861));
#25174=CARTESIAN_POINT('Ctrl Pts',(202.237819993686,92.8397376084047,334.314840364869));
#25175=CARTESIAN_POINT('Ctrl Pts',(204.03795315819,92.7772376084047,334.727687233877));
#25176=CARTESIAN_POINT('Ctrl Pts',(205.838086322694,92.7147376084047,335.140534102886));
#25177=CARTESIAN_POINT('Ctrl Pts',(206.819045869686,92.6522376084047,336.705347291213));
#25178=CARTESIAN_POINT('Ctrl Pts',(207.800005416678,92.5897376084047,338.27016047954));
#25179=CARTESIAN_POINT('Ctrl Pts',(207.38715854767,92.5272376084047,340.070293644044));
#25180=CARTESIAN_POINT('Ctrl Pts',(206.974311678662,92.4647376084047,341.870426808548));
#25181=CARTESIAN_POINT('Ctrl Pts',(205.409498490334,92.4022376084047,342.851386355541));
#25182=CARTESIAN_POINT('Ctrl Pts',(203.844685302007,92.3397376084047,343.832345902533));
#25183=CARTESIAN_POINT('Ctrl Pts',(202.044552137503,92.2772376084047,343.419499033524));
#25184=CARTESIAN_POINT('Ctrl Pts',(200.244418972999,92.2147376084047,343.006652164516));
#25185=CARTESIAN_POINT('Ctrl Pts',(199.263459426007,92.1522376084047,341.441838976189));
#25186=CARTESIAN_POINT('Ctrl Pts',(198.282499879015,92.0897376084047,339.877025787862));
#25187=CARTESIAN_POINT('Ctrl Pts',(198.695346748023,92.0272376084047,338.076892623358));
#25188=CARTESIAN_POINT('Ctrl Pts',(199.108193617031,91.9647376084047,336.276759458854));
#25189=CARTESIAN_POINT('Ctrl Pts',(200.673006805358,91.9022376084047,335.295799911861));
#25190=CARTESIAN_POINT('Ctrl Pts',(202.237819993686,91.8397376084047,334.314840364869));
#25191=CARTESIAN_POINT('Ctrl Pts',(204.03795315819,91.7772376084047,334.727687233877));
#25192=CARTESIAN_POINT('Ctrl Pts',(205.838086322694,91.7147376084047,335.140534102886));
#25193=CARTESIAN_POINT('Ctrl Pts',(206.819045869686,91.6522376084047,336.705347291213));
#25194=CARTESIAN_POINT('Ctrl Pts',(207.800005416678,91.5897376084047,338.27016047954));
#25195=CARTESIAN_POINT('Ctrl Pts',(207.38715854767,91.5272376084047,340.070293644044));
#25196=CARTESIAN_POINT('Ctrl Pts',(206.974311678662,91.4647376084047,341.870426808548));
#25197=CARTESIAN_POINT('Ctrl Pts',(205.409498490334,91.4022376084047,342.851386355541));
#25198=CARTESIAN_POINT('Ctrl Pts',(203.844685302007,91.3397376084047,343.832345902533));
#25199=CARTESIAN_POINT('Ctrl Pts',(202.044552137503,91.2772376084047,343.419499033524));
#25200=CARTESIAN_POINT('Ctrl Pts',(200.244418972999,91.2147376084047,343.006652164516));
#25201=CARTESIAN_POINT('Ctrl Pts',(199.263459426007,91.1522376084047,341.441838976189));
#25202=CARTESIAN_POINT('Ctrl Pts',(198.282499879015,91.0897376084047,339.877025787862));
#25203=CARTESIAN_POINT('Ctrl Pts',(198.695346748023,91.0272376084047,338.076892623358));
#25204=CARTESIAN_POINT('Ctrl Pts',(199.108193617031,90.9647376084047,336.276759458854));
#25205=CARTESIAN_POINT('Ctrl Pts',(200.673006805358,90.9022376084047,335.295799911861));
#25206=CARTESIAN_POINT('Ctrl Pts',(202.237819993686,90.8397376084047,334.314840364869));
#25207=CARTESIAN_POINT('Ctrl Pts',(204.03795315819,90.7772376084047,334.727687233877));
#25208=CARTESIAN_POINT('Ctrl Pts',(205.838086322694,90.7147376084047,335.140534102886));
#25209=CARTESIAN_POINT('Ctrl Pts',(206.819045869686,90.6522376084047,336.705347291213));
#25210=CARTESIAN_POINT('Ctrl Pts',(207.800005416678,90.5897376084047,338.27016047954));
#25211=CARTESIAN_POINT('Ctrl Pts',(207.38715854767,90.5272376084047,340.070293644044));
#25212=CARTESIAN_POINT('Ctrl Pts',(206.974311678662,90.4647376084047,341.870426808548));
#25213=CARTESIAN_POINT('Ctrl Pts',(205.409498490334,90.4022376084047,342.851386355541));
#25214=CARTESIAN_POINT('Ctrl Pts',(203.844685302007,90.3397376084047,343.832345902533));
#25215=CARTESIAN_POINT('Ctrl Pts',(202.044552137503,90.2772376084047,343.419499033524));
#25216=CARTESIAN_POINT('Ctrl Pts',(200.244418972999,90.2147376084047,343.006652164516));
#25217=CARTESIAN_POINT('Ctrl Pts',(199.263459426007,90.1522376084047,341.441838976189));
#25218=CARTESIAN_POINT('Ctrl Pts',(198.282499879015,90.0897376084047,339.877025787862));
#25219=CARTESIAN_POINT('Ctrl Pts',(198.695346748023,90.0272376084047,338.076892623358));
#25220=CARTESIAN_POINT('Ctrl Pts',(199.108193617031,89.9647376084047,336.276759458854));
#25221=CARTESIAN_POINT('Ctrl Pts',(200.673006805358,89.9022376084047,335.295799911861));
#25222=CARTESIAN_POINT('Ctrl Pts',(202.237819993686,89.8397376084047,334.314840364869));
#25223=CARTESIAN_POINT('Ctrl Pts',(204.03795315819,89.7772376084047,334.727687233877));
#25224=CARTESIAN_POINT('Ctrl Pts',(205.838086322694,89.7147376084047,335.140534102886));
#25225=CARTESIAN_POINT('Ctrl Pts',(206.819045869686,89.6522376084047,336.705347291213));
#25226=CARTESIAN_POINT('Ctrl Pts',(207.800005416678,89.5897376084047,338.27016047954));
#25227=CARTESIAN_POINT('Ctrl Pts',(207.38715854767,89.5272376084047,340.070293644044));
#25228=CARTESIAN_POINT('Ctrl Pts',(206.974311678662,89.4647376084047,341.870426808548));
#25229=CARTESIAN_POINT('Ctrl Pts',(205.409498490334,89.4022376084047,342.851386355541));
#25230=CARTESIAN_POINT('Ctrl Pts',(203.844685302007,89.3397376084047,343.832345902533));
#25231=CARTESIAN_POINT('Ctrl Pts',(202.044552137503,89.2772376084047,343.419499033524));
#25232=CARTESIAN_POINT('Ctrl Pts',(200.244418972999,89.2147376084047,343.006652164516));
#25233=CARTESIAN_POINT('Ctrl Pts',(199.263459426007,89.1522376084047,341.441838976189));
#25234=CARTESIAN_POINT('Ctrl Pts',(198.282499879015,89.0897376084047,339.877025787862));
#25235=CARTESIAN_POINT('Ctrl Pts',(198.695346748023,89.0272376084047,338.076892623358));
#25236=CARTESIAN_POINT('Ctrl Pts',(199.108193617031,88.9647376084047,336.276759458854));
#25237=CARTESIAN_POINT('Ctrl Pts',(200.673006805358,88.9022376084047,335.295799911861));
#25238=CARTESIAN_POINT('Ctrl Pts',(202.237819993686,88.8397376084047,334.314840364869));
#25239=CARTESIAN_POINT('Ctrl Pts',(204.03795315819,88.7772376084047,334.727687233877));
#25240=CARTESIAN_POINT('Ctrl Pts',(205.838086322694,88.7147376084047,335.140534102886));
#25241=CARTESIAN_POINT('Ctrl Pts',(206.819045869686,88.6522376084047,336.705347291213));
#25242=CARTESIAN_POINT('Ctrl Pts',(207.800005416678,88.5897376084047,338.27016047954));
#25243=CARTESIAN_POINT('Ctrl Pts',(207.38715854767,88.5272376084047,340.070293644044));
#25244=CARTESIAN_POINT('Ctrl Pts',(206.974311678662,88.4647376084047,341.870426808548));
#25245=CARTESIAN_POINT('Ctrl Pts',(205.409498490334,88.4022376084047,342.851386355541));
#25246=CARTESIAN_POINT('Ctrl Pts',(203.844685302007,88.3397376084047,343.832345902533));
#25247=CARTESIAN_POINT('Ctrl Pts',(202.044552137503,88.2772376084047,343.419499033524));
#25248=CARTESIAN_POINT('Ctrl Pts',(200.244418972999,88.2147376084047,343.006652164516));
#25249=CARTESIAN_POINT('Ctrl Pts',(199.263459426007,88.1522376084047,341.441838976189));
#25250=CARTESIAN_POINT('Ctrl Pts',(198.282499879015,88.0897376084047,339.877025787862));
#25251=CARTESIAN_POINT('Ctrl Pts',(198.695346748023,88.0272376084047,338.076892623358));
#25252=CARTESIAN_POINT('Ctrl Pts',(199.108193617031,87.9647376084047,336.276759458854));
#25253=CARTESIAN_POINT('Ctrl Pts',(200.673006805358,87.9022376084047,335.295799911861));
#25254=CARTESIAN_POINT('Ctrl Pts',(202.237819993686,87.8397376084047,334.314840364869));
#25255=CARTESIAN_POINT('Ctrl Pts',(204.03795315819,87.7772376084047,334.727687233877));
#25256=CARTESIAN_POINT('Ctrl Pts',(204.158947322422,102.089738090806,334.200117270057));
#25257=CARTESIAN_POINT('Ctrl Pts',(206.177607121041,102.027238090806,334.663081562858));
#25258=CARTESIAN_POINT('Ctrl Pts',(207.277649962667,101.964738090806,336.417854786258));
#25259=CARTESIAN_POINT('Ctrl Pts',(208.377692804292,101.902238090806,338.172628009657));
#25260=CARTESIAN_POINT('Ctrl Pts',(207.914728511491,101.839738090806,340.191287808277));
#25261=CARTESIAN_POINT('Ctrl Pts',(207.451764218689,101.777238090806,342.209947606896));
#25262=CARTESIAN_POINT('Ctrl Pts',(205.69699099529,101.714738090806,343.309990448521));
#25263=CARTESIAN_POINT('Ctrl Pts',(203.94221777189,101.652238090806,344.410033290147));
#25264=CARTESIAN_POINT('Ctrl Pts',(201.923557973271,101.589738090806,343.947068997345));
#25265=CARTESIAN_POINT('Ctrl Pts',(199.904898174651,101.527238090806,343.484104704544));
#25266=CARTESIAN_POINT('Ctrl Pts',(198.804855333026,101.464738090806,341.729331481144));
#25267=CARTESIAN_POINT('Ctrl Pts',(197.704812491401,101.402238090806,339.974558257745));
#25268=CARTESIAN_POINT('Ctrl Pts',(198.167776784202,101.339738090806,337.955898459125));
#25269=CARTESIAN_POINT('Ctrl Pts',(198.630741077004,101.277238090806,335.937238660506));
#25270=CARTESIAN_POINT('Ctrl Pts',(200.385514300403,101.214738090806,334.837195818881));
#25271=CARTESIAN_POINT('Ctrl Pts',(202.140287523803,101.152238090806,333.737152977255));
#25272=CARTESIAN_POINT('Ctrl Pts',(204.158947322422,101.089738090806,334.200117270057));
#25273=CARTESIAN_POINT('Ctrl Pts',(206.177607121041,101.027238090806,334.663081562858));
#25274=CARTESIAN_POINT('Ctrl Pts',(207.277649962667,100.964738090806,336.417854786258));
#25275=CARTESIAN_POINT('Ctrl Pts',(208.377692804292,100.902238090806,338.172628009657));
#25276=CARTESIAN_POINT('Ctrl Pts',(207.914728511491,100.839738090806,340.191287808277));
#25277=CARTESIAN_POINT('Ctrl Pts',(207.451764218689,100.777238090806,342.209947606896));
#25278=CARTESIAN_POINT('Ctrl Pts',(205.69699099529,100.714738090806,343.309990448521));
#25279=CARTESIAN_POINT('Ctrl Pts',(203.94221777189,100.652238090806,344.410033290147));
#25280=CARTESIAN_POINT('Ctrl Pts',(201.923557973271,100.589738090806,343.947068997345));
#25281=CARTESIAN_POINT('Ctrl Pts',(199.904898174651,100.527238090806,343.484104704544));
#25282=CARTESIAN_POINT('Ctrl Pts',(198.804855333026,100.464738090806,341.729331481144));
#25283=CARTESIAN_POINT('Ctrl Pts',(197.704812491401,100.402238090806,339.974558257745));
#25284=CARTESIAN_POINT('Ctrl Pts',(198.167776784202,100.339738090806,337.955898459125));
#25285=CARTESIAN_POINT('Ctrl Pts',(198.630741077004,100.277238090806,335.937238660506));
#25286=CARTESIAN_POINT('Ctrl Pts',(200.385514300403,100.214738090806,334.837195818881));
#25287=CARTESIAN_POINT('Ctrl Pts',(202.140287523803,100.152238090806,333.737152977255));
#25288=CARTESIAN_POINT('Ctrl Pts',(204.158947322422,100.089738090806,334.200117270057));
#25289=CARTESIAN_POINT('Ctrl Pts',(206.177607121041,100.027238090806,334.663081562858));
#25290=CARTESIAN_POINT('Ctrl Pts',(207.277649962667,99.9647380908064,336.417854786258));
#25291=CARTESIAN_POINT('Ctrl Pts',(208.377692804292,99.9022380908064,338.172628009657));
#25292=CARTESIAN_POINT('Ctrl Pts',(207.914728511491,99.8397380908065,340.191287808277));
#25293=CARTESIAN_POINT('Ctrl Pts',(207.451764218689,99.7772380908064,342.209947606896));
#25294=CARTESIAN_POINT('Ctrl Pts',(205.69699099529,99.7147380908064,343.309990448521));
#25295=CARTESIAN_POINT('Ctrl Pts',(203.94221777189,99.6522380908065,344.410033290147));
#25296=CARTESIAN_POINT('Ctrl Pts',(201.923557973271,99.5897380908065,343.947068997345));
#25297=CARTESIAN_POINT('Ctrl Pts',(199.904898174651,99.5272380908065,343.484104704544));
#25298=CARTESIAN_POINT('Ctrl Pts',(198.804855333026,99.4647380908065,341.729331481144));
#25299=CARTESIAN_POINT('Ctrl Pts',(197.704812491401,99.4022380908064,339.974558257745));
#25300=CARTESIAN_POINT('Ctrl Pts',(198.167776784202,99.3397380908064,337.955898459125));
#25301=CARTESIAN_POINT('Ctrl Pts',(198.630741077004,99.2772380908065,335.937238660506));
#25302=CARTESIAN_POINT('Ctrl Pts',(200.385514300403,99.2147380908065,334.837195818881));
#25303=CARTESIAN_POINT('Ctrl Pts',(202.140287523803,99.1522380908065,333.737152977255));
#25304=CARTESIAN_POINT('Ctrl Pts',(204.158947322422,99.0897380908064,334.200117270057));
#25305=CARTESIAN_POINT('Ctrl Pts',(206.177607121041,99.0272380908065,334.663081562858));
#25306=CARTESIAN_POINT('Ctrl Pts',(207.277649962667,98.9647380908064,336.417854786258));
#25307=CARTESIAN_POINT('Ctrl Pts',(208.377692804292,98.9022380908064,338.172628009657));
#25308=CARTESIAN_POINT('Ctrl Pts',(207.914728511491,98.8397380908065,340.191287808277));
#25309=CARTESIAN_POINT('Ctrl Pts',(207.451764218689,98.7772380908064,342.209947606896));
#25310=CARTESIAN_POINT('Ctrl Pts',(205.69699099529,98.7147380908064,343.309990448521));
#25311=CARTESIAN_POINT('Ctrl Pts',(203.94221777189,98.6522380908065,344.410033290147));
#25312=CARTESIAN_POINT('Ctrl Pts',(201.923557973271,98.5897380908064,343.947068997345));
#25313=CARTESIAN_POINT('Ctrl Pts',(199.904898174651,98.5272380908065,343.484104704544));
#25314=CARTESIAN_POINT('Ctrl Pts',(198.804855333026,98.4647380908065,341.729331481144));
#25315=CARTESIAN_POINT('Ctrl Pts',(197.704812491401,98.4022380908064,339.974558257745));
#25316=CARTESIAN_POINT('Ctrl Pts',(198.167776784202,98.3397380908064,337.955898459125));
#25317=CARTESIAN_POINT('Ctrl Pts',(198.630741077004,98.2772380908064,335.937238660506));
#25318=CARTESIAN_POINT('Ctrl Pts',(200.385514300403,98.2147380908065,334.837195818881));
#25319=CARTESIAN_POINT('Ctrl Pts',(202.140287523803,98.1522380908065,333.737152977255));
#25320=CARTESIAN_POINT('Ctrl Pts',(204.158947322422,98.0897380908065,334.200117270057));
#25321=CARTESIAN_POINT('Ctrl Pts',(206.177607121041,98.0272380908065,334.663081562858));
#25322=CARTESIAN_POINT('Ctrl Pts',(207.277649962667,97.9647380908064,336.417854786258));
#25323=CARTESIAN_POINT('Ctrl Pts',(208.377692804292,97.9022380908064,338.172628009657));
#25324=CARTESIAN_POINT('Ctrl Pts',(207.914728511491,97.8397380908065,340.191287808277));
#25325=CARTESIAN_POINT('Ctrl Pts',(207.451764218689,97.7772380908064,342.209947606896));
#25326=CARTESIAN_POINT('Ctrl Pts',(205.69699099529,97.7147380908064,343.309990448521));
#25327=CARTESIAN_POINT('Ctrl Pts',(203.94221777189,97.6522380908065,344.410033290147));
#25328=CARTESIAN_POINT('Ctrl Pts',(201.923557973271,97.5897380908064,343.947068997345));
#25329=CARTESIAN_POINT('Ctrl Pts',(199.904898174651,97.5272380908065,343.484104704544));
#25330=CARTESIAN_POINT('Ctrl Pts',(198.804855333026,97.4647380908065,341.729331481144));
#25331=CARTESIAN_POINT('Ctrl Pts',(197.704812491401,97.4022380908064,339.974558257745));
#25332=CARTESIAN_POINT('Ctrl Pts',(198.167776784202,97.3397380908064,337.955898459125));
#25333=CARTESIAN_POINT('Ctrl Pts',(198.630741077004,97.2772380908065,335.937238660506));
#25334=CARTESIAN_POINT('Ctrl Pts',(200.385514300403,97.2147380908064,334.837195818881));
#25335=CARTESIAN_POINT('Ctrl Pts',(202.140287523803,97.1522380908065,333.737152977255));
#25336=CARTESIAN_POINT('Ctrl Pts',(204.158947322422,97.0897380908065,334.200117270057));
#25337=CARTESIAN_POINT('Ctrl Pts',(206.177607121041,97.0272380908065,334.663081562858));
#25338=CARTESIAN_POINT('Ctrl Pts',(207.277649962667,96.9647380908064,336.417854786258));
#25339=CARTESIAN_POINT('Ctrl Pts',(208.377692804292,96.9022380908064,338.172628009657));
#25340=CARTESIAN_POINT('Ctrl Pts',(207.914728511491,96.8397380908065,340.191287808277));
#25341=CARTESIAN_POINT('Ctrl Pts',(207.451764218689,96.7772380908065,342.209947606896));
#25342=CARTESIAN_POINT('Ctrl Pts',(205.69699099529,96.7147380908065,343.309990448521));
#25343=CARTESIAN_POINT('Ctrl Pts',(203.94221777189,96.6522380908065,344.410033290147));
#25344=CARTESIAN_POINT('Ctrl Pts',(201.923557973271,96.5897380908064,343.947068997345));
#25345=CARTESIAN_POINT('Ctrl Pts',(199.904898174651,96.5272380908065,343.484104704544));
#25346=CARTESIAN_POINT('Ctrl Pts',(198.804855333026,96.4647380908065,341.729331481144));
#25347=CARTESIAN_POINT('Ctrl Pts',(197.704812491401,96.4022380908064,339.974558257745));
#25348=CARTESIAN_POINT('Ctrl Pts',(198.167776784202,96.3397380908064,337.955898459125));
#25349=CARTESIAN_POINT('Ctrl Pts',(198.630741077004,96.2772380908065,335.937238660506));
#25350=CARTESIAN_POINT('Ctrl Pts',(200.385514300403,96.2147380908064,334.837195818881));
#25351=CARTESIAN_POINT('Ctrl Pts',(202.140287523803,96.1522380908065,333.737152977255));
#25352=CARTESIAN_POINT('Ctrl Pts',(204.158947322422,96.0897380908065,334.200117270057));
#25353=CARTESIAN_POINT('Ctrl Pts',(206.177607121041,96.0272380908064,334.663081562858));
#25354=CARTESIAN_POINT('Ctrl Pts',(207.277649962667,95.9647380908064,336.417854786258));
#25355=CARTESIAN_POINT('Ctrl Pts',(208.377692804292,95.9022380908064,338.172628009657));
#25356=CARTESIAN_POINT('Ctrl Pts',(207.914728511491,95.8397380908064,340.191287808277));
#25357=CARTESIAN_POINT('Ctrl Pts',(207.451764218689,95.7772380908065,342.209947606896));
#25358=CARTESIAN_POINT('Ctrl Pts',(205.69699099529,95.7147380908064,343.309990448521));
#25359=CARTESIAN_POINT('Ctrl Pts',(203.94221777189,95.6522380908065,344.410033290147));
#25360=CARTESIAN_POINT('Ctrl Pts',(201.923557973271,95.5897380908064,343.947068997345));
#25361=CARTESIAN_POINT('Ctrl Pts',(199.904898174651,95.5272380908064,343.484104704544));
#25362=CARTESIAN_POINT('Ctrl Pts',(198.804855333026,95.4647380908065,341.729331481144));
#25363=CARTESIAN_POINT('Ctrl Pts',(197.704812491401,95.4022380908064,339.974558257745));
#25364=CARTESIAN_POINT('Ctrl Pts',(198.167776784202,95.3397380908065,337.955898459125));
#25365=CARTESIAN_POINT('Ctrl Pts',(198.630741077004,95.2772380908065,335.937238660506));
#25366=CARTESIAN_POINT('Ctrl Pts',(200.385514300403,95.2147380908064,334.837195818881));
#25367=CARTESIAN_POINT('Ctrl Pts',(202.140287523803,95.1522380908065,333.737152977255));
#25368=CARTESIAN_POINT('Ctrl Pts',(204.158947322422,95.0897380908064,334.200117270057));
#25369=CARTESIAN_POINT('Ctrl Pts',(206.177607121041,95.0272380908064,334.663081562858));
#25370=CARTESIAN_POINT('Ctrl Pts',(207.277649962667,94.9647380908064,336.417854786258));
#25371=CARTESIAN_POINT('Ctrl Pts',(208.377692804292,94.9022380908064,338.172628009657));
#25372=CARTESIAN_POINT('Ctrl Pts',(207.914728511491,94.8397380908064,340.191287808277));
#25373=CARTESIAN_POINT('Ctrl Pts',(207.451764218689,94.7772380908064,342.209947606896));
#25374=CARTESIAN_POINT('Ctrl Pts',(205.69699099529,94.7147380908065,343.309990448521));
#25375=CARTESIAN_POINT('Ctrl Pts',(203.94221777189,94.6522380908065,344.410033290147));
#25376=CARTESIAN_POINT('Ctrl Pts',(201.923557973271,94.5897380908064,343.947068997345));
#25377=CARTESIAN_POINT('Ctrl Pts',(199.904898174651,94.5272380908064,343.484104704544));
#25378=CARTESIAN_POINT('Ctrl Pts',(198.804855333026,94.4647380908064,341.729331481144));
#25379=CARTESIAN_POINT('Ctrl Pts',(197.704812491401,94.4022380908064,339.974558257745));
#25380=CARTESIAN_POINT('Ctrl Pts',(198.167776784202,94.3397380908065,337.955898459125));
#25381=CARTESIAN_POINT('Ctrl Pts',(198.630741077004,94.2772380908064,335.937238660506));
#25382=CARTESIAN_POINT('Ctrl Pts',(200.385514300403,94.2147380908064,334.837195818881));
#25383=CARTESIAN_POINT('Ctrl Pts',(202.140287523803,94.1522380908065,333.737152977255));
#25384=CARTESIAN_POINT('Ctrl Pts',(204.158947322422,94.0897380908065,334.200117270057));
#25385=CARTESIAN_POINT('Ctrl Pts',(206.177607121041,94.0272380908064,334.663081562858));
#25386=CARTESIAN_POINT('Ctrl Pts',(207.277649962667,93.9647380908065,336.417854786258));
#25387=CARTESIAN_POINT('Ctrl Pts',(208.377692804292,93.9022380908064,338.172628009657));
#25388=CARTESIAN_POINT('Ctrl Pts',(207.914728511491,93.8397380908064,340.191287808277));
#25389=CARTESIAN_POINT('Ctrl Pts',(207.451764218689,93.7772380908065,342.209947606896));
#25390=CARTESIAN_POINT('Ctrl Pts',(205.69699099529,93.7147380908065,343.309990448521));
#25391=CARTESIAN_POINT('Ctrl Pts',(203.94221777189,93.6522380908064,344.410033290147));
#25392=CARTESIAN_POINT('Ctrl Pts',(201.923557973271,93.5897380908064,343.947068997345));
#25393=CARTESIAN_POINT('Ctrl Pts',(199.904898174651,93.5272380908064,343.484104704544));
#25394=CARTESIAN_POINT('Ctrl Pts',(198.804855333026,93.4647380908064,341.729331481144));
#25395=CARTESIAN_POINT('Ctrl Pts',(197.704812491401,93.4022380908064,339.974558257745));
#25396=CARTESIAN_POINT('Ctrl Pts',(198.167776784202,93.3397380908065,337.955898459125));
#25397=CARTESIAN_POINT('Ctrl Pts',(198.630741077004,93.2772380908065,335.937238660506));
#25398=CARTESIAN_POINT('Ctrl Pts',(200.385514300403,93.2147380908064,334.837195818881));
#25399=CARTESIAN_POINT('Ctrl Pts',(202.140287523803,93.1522380908065,333.737152977255));
#25400=CARTESIAN_POINT('Ctrl Pts',(204.158947322422,93.0897380908064,334.200117270057));
#25401=CARTESIAN_POINT('Ctrl Pts',(206.177607121041,93.0272380908064,334.663081562858));
#25402=CARTESIAN_POINT('Ctrl Pts',(207.277649962667,92.9647380908065,336.417854786258));
#25403=CARTESIAN_POINT('Ctrl Pts',(208.377692804292,92.9022380908064,338.172628009657));
#25404=CARTESIAN_POINT('Ctrl Pts',(207.914728511491,92.8397380908064,340.191287808277));
#25405=CARTESIAN_POINT('Ctrl Pts',(207.451764218689,92.7772380908065,342.209947606896));
#25406=CARTESIAN_POINT('Ctrl Pts',(205.69699099529,92.7147380908065,343.309990448521));
#25407=CARTESIAN_POINT('Ctrl Pts',(203.94221777189,92.6522380908065,344.410033290147));
#25408=CARTESIAN_POINT('Ctrl Pts',(201.923557973271,92.5897380908064,343.947068997345));
#25409=CARTESIAN_POINT('Ctrl Pts',(199.904898174651,92.5272380908064,343.484104704544));
#25410=CARTESIAN_POINT('Ctrl Pts',(198.804855333026,92.4647380908064,341.729331481144));
#25411=CARTESIAN_POINT('Ctrl Pts',(197.704812491401,92.4022380908064,339.974558257745));
#25412=CARTESIAN_POINT('Ctrl Pts',(198.167776784202,92.3397380908065,337.955898459125));
#25413=CARTESIAN_POINT('Ctrl Pts',(198.630741077004,92.2772380908064,335.937238660506));
#25414=CARTESIAN_POINT('Ctrl Pts',(200.385514300403,92.2147380908064,334.837195818881));
#25415=CARTESIAN_POINT('Ctrl Pts',(202.140287523803,92.1522380908065,333.737152977255));
#25416=CARTESIAN_POINT('Ctrl Pts',(204.158947322422,92.0897380908064,334.200117270057));
#25417=CARTESIAN_POINT('Ctrl Pts',(206.177607121041,92.0272380908064,334.663081562858));
#25418=CARTESIAN_POINT('Ctrl Pts',(207.277649962667,91.9647380908064,336.417854786258));
#25419=CARTESIAN_POINT('Ctrl Pts',(208.377692804292,91.9022380908064,338.172628009657));
#25420=CARTESIAN_POINT('Ctrl Pts',(207.914728511491,91.8397380908064,340.191287808277));
#25421=CARTESIAN_POINT('Ctrl Pts',(207.451764218689,91.7772380908065,342.209947606896));
#25422=CARTESIAN_POINT('Ctrl Pts',(205.69699099529,91.7147380908064,343.309990448521));
#25423=CARTESIAN_POINT('Ctrl Pts',(203.94221777189,91.6522380908064,344.410033290147));
#25424=CARTESIAN_POINT('Ctrl Pts',(201.923557973271,91.5897380908064,343.947068997345));
#25425=CARTESIAN_POINT('Ctrl Pts',(199.904898174651,91.5272380908064,343.484104704544));
#25426=CARTESIAN_POINT('Ctrl Pts',(198.804855333026,91.4647380908064,341.729331481144));
#25427=CARTESIAN_POINT('Ctrl Pts',(197.704812491401,91.4022380908064,339.974558257745));
#25428=CARTESIAN_POINT('Ctrl Pts',(198.167776784202,91.3397380908064,337.955898459125));
#25429=CARTESIAN_POINT('Ctrl Pts',(198.630741077004,91.2772380908065,335.937238660506));
#25430=CARTESIAN_POINT('Ctrl Pts',(200.385514300403,91.2147380908064,334.837195818881));
#25431=CARTESIAN_POINT('Ctrl Pts',(202.140287523803,91.1522380908065,333.737152977255));
#25432=CARTESIAN_POINT('Ctrl Pts',(204.158947322422,91.0897380908064,334.200117270057));
#25433=CARTESIAN_POINT('Ctrl Pts',(206.177607121041,91.0272380908064,334.663081562858));
#25434=CARTESIAN_POINT('Ctrl Pts',(207.277649962667,90.9647380908065,336.417854786258));
#25435=CARTESIAN_POINT('Ctrl Pts',(208.377692804292,90.9022380908064,338.172628009657));
#25436=CARTESIAN_POINT('Ctrl Pts',(207.914728511491,90.8397380908064,340.191287808277));
#25437=CARTESIAN_POINT('Ctrl Pts',(207.451764218689,90.7772380908065,342.209947606896));
#25438=CARTESIAN_POINT('Ctrl Pts',(205.69699099529,90.7147380908064,343.309990448521));
#25439=CARTESIAN_POINT('Ctrl Pts',(203.94221777189,90.6522380908064,344.410033290147));
#25440=CARTESIAN_POINT('Ctrl Pts',(201.923557973271,90.5897380908065,343.947068997345));
#25441=CARTESIAN_POINT('Ctrl Pts',(199.904898174651,90.5272380908064,343.484104704544));
#25442=CARTESIAN_POINT('Ctrl Pts',(198.804855333026,90.4647380908064,341.729331481144));
#25443=CARTESIAN_POINT('Ctrl Pts',(197.704812491401,90.4022380908064,339.974558257745));
#25444=CARTESIAN_POINT('Ctrl Pts',(198.167776784202,90.3397380908064,337.955898459125));
#25445=CARTESIAN_POINT('Ctrl Pts',(198.630741077004,90.2772380908065,335.937238660506));
#25446=CARTESIAN_POINT('Ctrl Pts',(200.385514300403,90.2147380908065,334.837195818881));
#25447=CARTESIAN_POINT('Ctrl Pts',(202.140287523803,90.1522380908065,333.737152977255));
#25448=CARTESIAN_POINT('Ctrl Pts',(204.158947322422,90.0897380908064,334.200117270057));
#25449=CARTESIAN_POINT('Ctrl Pts',(206.177607121041,90.0272380908064,334.663081562858));
#25450=CARTESIAN_POINT('Ctrl Pts',(207.277649962667,89.9647380908065,336.417854786258));
#25451=CARTESIAN_POINT('Ctrl Pts',(208.377692804292,89.9022380908064,338.172628009657));
#25452=CARTESIAN_POINT('Ctrl Pts',(207.914728511491,89.8397380908065,340.191287808277));
#25453=CARTESIAN_POINT('Ctrl Pts',(207.451764218689,89.7772380908064,342.209947606896));
#25454=CARTESIAN_POINT('Ctrl Pts',(205.69699099529,89.7147380908064,343.309990448521));
#25455=CARTESIAN_POINT('Ctrl Pts',(203.94221777189,89.6522380908064,344.410033290147));
#25456=CARTESIAN_POINT('Ctrl Pts',(201.923557973271,89.5897380908065,343.947068997345));
#25457=CARTESIAN_POINT('Ctrl Pts',(199.904898174651,89.5272380908064,343.484104704544));
#25458=CARTESIAN_POINT('Ctrl Pts',(198.804855333026,89.4647380908064,341.729331481144));
#25459=CARTESIAN_POINT('Ctrl Pts',(197.704812491401,89.4022380908064,339.974558257745));
#25460=CARTESIAN_POINT('Ctrl Pts',(198.167776784202,89.3397380908064,337.955898459125));
#25461=CARTESIAN_POINT('Ctrl Pts',(198.630741077004,89.2772380908065,335.937238660506));
#25462=CARTESIAN_POINT('Ctrl Pts',(200.385514300403,89.2147380908065,334.837195818881));
#25463=CARTESIAN_POINT('Ctrl Pts',(202.140287523803,89.1522380908064,333.737152977255));
#25464=CARTESIAN_POINT('Ctrl Pts',(204.158947322422,89.0897380908064,334.200117270057));
#25465=CARTESIAN_POINT('Ctrl Pts',(206.177607121041,89.0272380908065,334.663081562858));
#25466=CARTESIAN_POINT('Ctrl Pts',(207.277649962667,88.9647380908064,336.417854786258));
#25467=CARTESIAN_POINT('Ctrl Pts',(208.377692804292,88.9022380908065,338.172628009657));
#25468=CARTESIAN_POINT('Ctrl Pts',(207.914728511491,88.8397380908064,340.191287808277));
#25469=CARTESIAN_POINT('Ctrl Pts',(207.451764218689,88.7772380908064,342.209947606896));
#25470=CARTESIAN_POINT('Ctrl Pts',(205.69699099529,88.7147380908064,343.309990448521));
#25471=CARTESIAN_POINT('Ctrl Pts',(203.94221777189,88.6522380908064,344.410033290147));
#25472=CARTESIAN_POINT('Ctrl Pts',(201.923557973271,88.5897380908065,343.947068997345));
#25473=CARTESIAN_POINT('Ctrl Pts',(199.904898174651,88.5272380908064,343.484104704544));
#25474=CARTESIAN_POINT('Ctrl Pts',(198.804855333026,88.4647380908065,341.729331481144));
#25475=CARTESIAN_POINT('Ctrl Pts',(197.704812491401,88.4022380908065,339.974558257745));
#25476=CARTESIAN_POINT('Ctrl Pts',(198.167776784202,88.3397380908064,337.955898459125));
#25477=CARTESIAN_POINT('Ctrl Pts',(198.630741077004,88.2772380908065,335.937238660506));
#25478=CARTESIAN_POINT('Ctrl Pts',(200.385514300403,88.2147380908064,334.837195818881));
#25479=CARTESIAN_POINT('Ctrl Pts',(202.140287523803,88.1522380908064,333.737152977255));
#25480=CARTESIAN_POINT('Ctrl Pts',(204.158947322422,88.0897380908064,334.200117270057));
#25481=CARTESIAN_POINT('Ctrl Pts',(207.107563775619,100.631003482039,337.244543159099));
#25482=CARTESIAN_POINT('Ctrl Pts',(207.721960531643,100.577922561033,338.610459017374));
#25483=CARTESIAN_POINT('Ctrl Pts',(207.38715854767,100.527237608405,340.070293644044));
#25484=CARTESIAN_POINT('Ctrl Pts',(206.974311678662,100.464737608405,341.870426808548));
#25485=CARTESIAN_POINT('Ctrl Pts',(205.409498490334,100.402237608405,342.851386355541));
#25486=CARTESIAN_POINT('Ctrl Pts',(203.844685302007,100.339737608405,343.832345902533));
#25487=CARTESIAN_POINT('Ctrl Pts',(202.044552137503,100.277237608405,343.419499033524));
#25488=CARTESIAN_POINT('Origin',(203.041252647847,101.652237608405,339.0735931337));
#25489=CARTESIAN_POINT('Ctrl Pts',(201.212202673244,100.631003482039,335.007282005928));
#25490=CARTESIAN_POINT('Ctrl Pts',(202.578118531519,100.577922561033,334.392885249905));
#25491=CARTESIAN_POINT('Ctrl Pts',(204.03795315819,100.527237608405,334.727687233877));
#25492=CARTESIAN_POINT('Ctrl Pts',(205.838086322694,100.464737608405,335.140534102886));
#25493=CARTESIAN_POINT('Ctrl Pts',(206.819045869686,100.402237608405,336.705347291213));
#25494=CARTESIAN_POINT('Ctrl Pts',(207.800005416678,100.339737608405,338.27016047954));
#25495=CARTESIAN_POINT('Ctrl Pts',(207.38715854767,100.277237608405,340.070293644044));
#25496=CARTESIAN_POINT('Ctrl Pts',(206.974311678662,100.214737608405,341.870426808548));
#25497=CARTESIAN_POINT('Ctrl Pts',(205.409498490334,100.152237608405,342.851386355541));
#25498=CARTESIAN_POINT('Ctrl Pts',(203.844685302007,100.089737608405,343.832345902533));
#25499=CARTESIAN_POINT('Ctrl Pts',(202.044552137503,100.027237608405,343.419499033524));
#25500=CARTESIAN_POINT('Ctrl Pts',(204.158947135117,101.21473760977,334.200118086763));
#25501=CARTESIAN_POINT('Ctrl Pts',(206.177606595445,101.15223760977,334.66308230198));
#25502=CARTESIAN_POINT('Ctrl Pts',(207.277649252723,101.08973760977,336.417855231311));
#25503=CARTESIAN_POINT('Ctrl Pts',(208.377691910001,101.02723760977,338.172628160643));
#25504=CARTESIAN_POINT('Ctrl Pts',(207.914727694784,100.96473760977,340.191287620971));
#25505=CARTESIAN_POINT('Ctrl Pts',(207.451763479567,100.90223760977,342.2099470813));
#25506=CARTESIAN_POINT('Ctrl Pts',(205.696990550236,100.83973760977,343.309989738578));
#25507=CARTESIAN_POINT('Ctrl Pts',(203.942217620905,100.77723760977,344.410032395856));
#25508=CARTESIAN_POINT('Ctrl Pts',(201.923558160576,100.71473760977,343.947068180639));
#25509=CARTESIAN_POINT('Ctrl Pts',(199.904898700248,100.65223760977,343.484103965422));
#25510=CARTESIAN_POINT('Ctrl Pts',(198.80485604297,100.58973760977,341.72933103609));
#25511=CARTESIAN_POINT('Ctrl Pts',(197.704813385692,100.52723760977,339.974558106759));
#25512=CARTESIAN_POINT('Ctrl Pts',(198.167777600909,100.46473760977,337.955898646431));
#25513=CARTESIAN_POINT('Ctrl Pts',(198.630741816126,100.40223760977,335.937239186102));
#25514=CARTESIAN_POINT('Ctrl Pts',(200.385514745457,100.33973760977,334.837196528824));
#25515=CARTESIAN_POINT('Ctrl Pts',(202.140287674788,100.27723760977,333.737153871546));
#25516=CARTESIAN_POINT('Ctrl Pts',(204.158947135117,100.21473760977,334.200118086763));
#25517=CARTESIAN_POINT('Ctrl Pts',(206.177606595445,100.15223760977,334.66308230198));
#25518=CARTESIAN_POINT('Ctrl Pts',(207.277649252723,100.08973760977,336.417855231311));
#25519=CARTESIAN_POINT('Ctrl Pts',(208.377691910001,100.02723760977,338.172628160643));
#25520=CARTESIAN_POINT('Ctrl Pts',(207.914727694784,99.9647376097703,340.191287620971));
#25521=CARTESIAN_POINT('Ctrl Pts',(207.451763479567,99.9022376097703,342.2099470813));
#25522=CARTESIAN_POINT('Ctrl Pts',(205.696990550236,99.8397376097703,343.309989738578));
#25523=CARTESIAN_POINT('Ctrl Pts',(203.942217620905,99.7772376097703,344.410032395856));
#25524=CARTESIAN_POINT('Ctrl Pts',(201.923558160576,99.7147376097703,343.947068180639));
#25525=CARTESIAN_POINT('Ctrl Pts',(199.904898700248,99.6522376097703,343.484103965422));
#25526=CARTESIAN_POINT('Ctrl Pts',(198.80485604297,99.5897376097703,341.72933103609));
#25527=CARTESIAN_POINT('Ctrl Pts',(197.704813385692,99.5272376097703,339.974558106759));
#25528=CARTESIAN_POINT('Ctrl Pts',(198.167777600909,99.4647376097703,337.955898646431));
#25529=CARTESIAN_POINT('Ctrl Pts',(198.630741816126,99.4022376097703,335.937239186102));
#25530=CARTESIAN_POINT('Ctrl Pts',(200.385514745457,99.3397376097703,334.837196528824));
#25531=CARTESIAN_POINT('Ctrl Pts',(202.140287674788,99.2772376097703,333.737153871546));
#25532=CARTESIAN_POINT('Ctrl Pts',(204.158947135117,99.2147376097703,334.200118086763));
#25533=CARTESIAN_POINT('Ctrl Pts',(206.177606595445,99.1522376097703,334.66308230198));
#25534=CARTESIAN_POINT('Ctrl Pts',(207.277649252723,99.0897376097703,336.417855231311));
#25535=CARTESIAN_POINT('Ctrl Pts',(208.377691910001,99.0272376097703,338.172628160643));
#25536=CARTESIAN_POINT('Ctrl Pts',(207.914727694784,98.9647376097703,340.191287620971));
#25537=CARTESIAN_POINT('Ctrl Pts',(207.451763479567,98.9022376097703,342.2099470813));
#25538=CARTESIAN_POINT('Ctrl Pts',(205.696990550236,98.8397376097703,343.309989738578));
#25539=CARTESIAN_POINT('Ctrl Pts',(203.942217620905,98.7772376097703,344.410032395856));
#25540=CARTESIAN_POINT('Ctrl Pts',(201.923558160576,98.7147376097703,343.947068180639));
#25541=CARTESIAN_POINT('Ctrl Pts',(199.904898700248,98.6522376097703,343.484103965422));
#25542=CARTESIAN_POINT('Ctrl Pts',(198.80485604297,98.5897376097703,341.72933103609));
#25543=CARTESIAN_POINT('Ctrl Pts',(197.704813385692,98.5272376097703,339.974558106759));
#25544=CARTESIAN_POINT('Ctrl Pts',(198.167777600909,98.4647376097703,337.955898646431));
#25545=CARTESIAN_POINT('Ctrl Pts',(198.630741816126,98.4022376097703,335.937239186102));
#25546=CARTESIAN_POINT('Ctrl Pts',(200.385514745457,98.3397376097703,334.837196528824));
#25547=CARTESIAN_POINT('Ctrl Pts',(202.140287674788,98.2772376097703,333.737153871546));
#25548=CARTESIAN_POINT('Ctrl Pts',(204.158947135117,98.2147376097703,334.200118086763));
#25549=CARTESIAN_POINT('Ctrl Pts',(206.177606595445,98.1522376097703,334.66308230198));
#25550=CARTESIAN_POINT('Ctrl Pts',(207.277649252723,98.0897376097703,336.417855231311));
#25551=CARTESIAN_POINT('Ctrl Pts',(208.377691910001,98.0272376097703,338.172628160643));
#25552=CARTESIAN_POINT('Ctrl Pts',(207.914727694784,97.9647376097703,340.191287620971));
#25553=CARTESIAN_POINT('Ctrl Pts',(207.451763479567,97.9022376097703,342.2099470813));
#25554=CARTESIAN_POINT('Ctrl Pts',(205.696990550236,97.8397376097703,343.309989738578));
#25555=CARTESIAN_POINT('Ctrl Pts',(203.942217620905,97.7772376097703,344.410032395856));
#25556=CARTESIAN_POINT('Ctrl Pts',(201.923558160576,97.7147376097703,343.947068180639));
#25557=CARTESIAN_POINT('Ctrl Pts',(199.904898700248,97.6522376097703,343.484103965422));
#25558=CARTESIAN_POINT('Ctrl Pts',(198.80485604297,97.5897376097703,341.72933103609));
#25559=CARTESIAN_POINT('Ctrl Pts',(197.704813385692,97.5272376097703,339.974558106759));
#25560=CARTESIAN_POINT('Ctrl Pts',(198.167777600909,97.4647376097703,337.955898646431));
#25561=CARTESIAN_POINT('Ctrl Pts',(198.630741816126,97.4022376097703,335.937239186102));
#25562=CARTESIAN_POINT('Ctrl Pts',(200.385514745457,97.3397376097703,334.837196528824));
#25563=CARTESIAN_POINT('Ctrl Pts',(202.140287674788,97.2772376097703,333.737153871546));
#25564=CARTESIAN_POINT('Ctrl Pts',(204.158947135117,97.2147376097703,334.200118086763));
#25565=CARTESIAN_POINT('Ctrl Pts',(206.177606595445,97.1522376097703,334.66308230198));
#25566=CARTESIAN_POINT('Ctrl Pts',(207.277649252723,97.0897376097703,336.417855231311));
#25567=CARTESIAN_POINT('Ctrl Pts',(208.377691910001,97.0272376097703,338.172628160643));
#25568=CARTESIAN_POINT('Ctrl Pts',(207.914727694784,96.9647376097703,340.191287620971));
#25569=CARTESIAN_POINT('Ctrl Pts',(207.451763479567,96.9022376097703,342.2099470813));
#25570=CARTESIAN_POINT('Ctrl Pts',(205.696990550236,96.8397376097703,343.309989738578));
#25571=CARTESIAN_POINT('Ctrl Pts',(203.942217620905,96.7772376097703,344.410032395856));
#25572=CARTESIAN_POINT('Ctrl Pts',(201.923558160576,96.7147376097703,343.947068180639));
#25573=CARTESIAN_POINT('Ctrl Pts',(199.904898700248,96.6522376097703,343.484103965422));
#25574=CARTESIAN_POINT('Ctrl Pts',(198.80485604297,96.5897376097703,341.72933103609));
#25575=CARTESIAN_POINT('Ctrl Pts',(197.704813385692,96.5272376097703,339.974558106759));
#25576=CARTESIAN_POINT('Ctrl Pts',(198.167777600909,96.4647376097703,337.955898646431));
#25577=CARTESIAN_POINT('Ctrl Pts',(198.630741816126,96.4022376097703,335.937239186102));
#25578=CARTESIAN_POINT('Ctrl Pts',(200.385514745457,96.3397376097703,334.837196528824));
#25579=CARTESIAN_POINT('Ctrl Pts',(202.140287674788,96.2772376097703,333.737153871546));
#25580=CARTESIAN_POINT('Ctrl Pts',(204.158947135117,96.2147376097703,334.200118086763));
#25581=CARTESIAN_POINT('Ctrl Pts',(206.177606595445,96.1522376097703,334.66308230198));
#25582=CARTESIAN_POINT('Ctrl Pts',(207.277649252723,96.0897376097703,336.417855231311));
#25583=CARTESIAN_POINT('Ctrl Pts',(208.377691910001,96.0272376097703,338.172628160643));
#25584=CARTESIAN_POINT('Ctrl Pts',(207.914727694784,95.9647376097703,340.191287620971));
#25585=CARTESIAN_POINT('Ctrl Pts',(207.451763479567,95.9022376097703,342.2099470813));
#25586=CARTESIAN_POINT('Ctrl Pts',(205.696990550236,95.8397376097703,343.309989738578));
#25587=CARTESIAN_POINT('Ctrl Pts',(203.942217620905,95.7772376097703,344.410032395856));
#25588=CARTESIAN_POINT('Ctrl Pts',(201.923558160576,95.7147376097703,343.947068180639));
#25589=CARTESIAN_POINT('Ctrl Pts',(199.904898700248,95.6522376097703,343.484103965422));
#25590=CARTESIAN_POINT('Ctrl Pts',(198.80485604297,95.5897376097703,341.72933103609));
#25591=CARTESIAN_POINT('Ctrl Pts',(197.704813385692,95.5272376097703,339.974558106759));
#25592=CARTESIAN_POINT('Ctrl Pts',(198.167777600909,95.4647376097703,337.955898646431));
#25593=CARTESIAN_POINT('Ctrl Pts',(198.630741816126,95.4022376097703,335.937239186102));
#25594=CARTESIAN_POINT('Ctrl Pts',(200.385514745457,95.3397376097703,334.837196528824));
#25595=CARTESIAN_POINT('Ctrl Pts',(202.140287674788,95.2772376097703,333.737153871546));
#25596=CARTESIAN_POINT('Ctrl Pts',(204.158947135117,95.2147376097703,334.200118086763));
#25597=CARTESIAN_POINT('Ctrl Pts',(206.177606595445,95.1522376097703,334.66308230198));
#25598=CARTESIAN_POINT('Ctrl Pts',(207.277649252723,95.0897376097703,336.417855231311));
#25599=CARTESIAN_POINT('Ctrl Pts',(208.377691910001,95.0272376097703,338.172628160643));
#25600=CARTESIAN_POINT('Ctrl Pts',(207.914727694784,94.9647376097703,340.191287620971));
#25601=CARTESIAN_POINT('Ctrl Pts',(207.451763479567,94.9022376097703,342.2099470813));
#25602=CARTESIAN_POINT('Ctrl Pts',(205.696990550236,94.8397376097703,343.309989738578));
#25603=CARTESIAN_POINT('Ctrl Pts',(203.942217620905,94.7772376097703,344.410032395856));
#25604=CARTESIAN_POINT('Ctrl Pts',(201.923558160576,94.7147376097703,343.947068180639));
#25605=CARTESIAN_POINT('Ctrl Pts',(199.904898700248,94.6522376097703,343.484103965422));
#25606=CARTESIAN_POINT('Ctrl Pts',(198.80485604297,94.5897376097703,341.72933103609));
#25607=CARTESIAN_POINT('Ctrl Pts',(197.704813385692,94.5272376097703,339.974558106759));
#25608=CARTESIAN_POINT('Ctrl Pts',(198.167777600909,94.4647376097703,337.955898646431));
#25609=CARTESIAN_POINT('Ctrl Pts',(198.630741816126,94.4022376097703,335.937239186102));
#25610=CARTESIAN_POINT('Ctrl Pts',(200.385514745457,94.3397376097703,334.837196528824));
#25611=CARTESIAN_POINT('Ctrl Pts',(202.140287674788,94.2772376097703,333.737153871546));
#25612=CARTESIAN_POINT('Ctrl Pts',(204.158947135117,94.2147376097703,334.200118086763));
#25613=CARTESIAN_POINT('Ctrl Pts',(206.177606595445,94.1522376097703,334.66308230198));
#25614=CARTESIAN_POINT('Ctrl Pts',(207.277649252723,94.0897376097703,336.417855231311));
#25615=CARTESIAN_POINT('Ctrl Pts',(208.377691910001,94.0272376097703,338.172628160643));
#25616=CARTESIAN_POINT('Ctrl Pts',(207.914727694784,93.9647376097703,340.191287620971));
#25617=CARTESIAN_POINT('Ctrl Pts',(207.451763479567,93.9022376097703,342.2099470813));
#25618=CARTESIAN_POINT('Ctrl Pts',(205.696990550236,93.8397376097703,343.309989738578));
#25619=CARTESIAN_POINT('Ctrl Pts',(203.942217620905,93.7772376097703,344.410032395856));
#25620=CARTESIAN_POINT('Ctrl Pts',(201.923558160576,93.7147376097703,343.947068180639));
#25621=CARTESIAN_POINT('Ctrl Pts',(199.904898700248,93.6522376097703,343.484103965422));
#25622=CARTESIAN_POINT('Ctrl Pts',(198.80485604297,93.5897376097703,341.72933103609));
#25623=CARTESIAN_POINT('Ctrl Pts',(197.704813385692,93.5272376097703,339.974558106759));
#25624=CARTESIAN_POINT('Ctrl Pts',(198.167777600909,93.4647376097703,337.955898646431));
#25625=CARTESIAN_POINT('Ctrl Pts',(198.630741816126,93.4022376097703,335.937239186102));
#25626=CARTESIAN_POINT('Ctrl Pts',(200.385514745457,93.3397376097703,334.837196528824));
#25627=CARTESIAN_POINT('Ctrl Pts',(202.140287674788,93.2772376097703,333.737153871546));
#25628=CARTESIAN_POINT('Ctrl Pts',(204.158947135117,93.2147376097703,334.200118086763));
#25629=CARTESIAN_POINT('Ctrl Pts',(206.177606595445,93.1522376097703,334.66308230198));
#25630=CARTESIAN_POINT('Ctrl Pts',(207.277649252723,93.0897376097703,336.417855231311));
#25631=CARTESIAN_POINT('Ctrl Pts',(208.377691910001,93.0272376097703,338.172628160643));
#25632=CARTESIAN_POINT('Ctrl Pts',(207.914727694784,92.9647376097703,340.191287620971));
#25633=CARTESIAN_POINT('Ctrl Pts',(207.451763479567,92.9022376097703,342.2099470813));
#25634=CARTESIAN_POINT('Ctrl Pts',(205.696990550236,92.8397376097703,343.309989738578));
#25635=CARTESIAN_POINT('Ctrl Pts',(203.942217620905,92.7772376097703,344.410032395856));
#25636=CARTESIAN_POINT('Ctrl Pts',(201.923558160576,92.7147376097703,343.947068180639));
#25637=CARTESIAN_POINT('Ctrl Pts',(199.904898700248,92.6522376097703,343.484103965422));
#25638=CARTESIAN_POINT('Ctrl Pts',(198.80485604297,92.5897376097703,341.72933103609));
#25639=CARTESIAN_POINT('Ctrl Pts',(197.704813385692,92.5272376097703,339.974558106759));
#25640=CARTESIAN_POINT('Ctrl Pts',(198.167777600909,92.4647376097703,337.955898646431));
#25641=CARTESIAN_POINT('Ctrl Pts',(198.630741816126,92.4022376097703,335.937239186102));
#25642=CARTESIAN_POINT('Ctrl Pts',(200.385514745457,92.3397376097703,334.837196528824));
#25643=CARTESIAN_POINT('Ctrl Pts',(202.140287674788,92.2772376097703,333.737153871546));
#25644=CARTESIAN_POINT('Ctrl Pts',(204.158947135117,92.2147376097703,334.200118086763));
#25645=CARTESIAN_POINT('Ctrl Pts',(206.177606595445,92.1522376097703,334.66308230198));
#25646=CARTESIAN_POINT('Ctrl Pts',(207.277649252723,92.0897376097703,336.417855231311));
#25647=CARTESIAN_POINT('Ctrl Pts',(208.377691910001,92.0272376097703,338.172628160643));
#25648=CARTESIAN_POINT('Ctrl Pts',(207.914727694784,91.9647376097703,340.191287620971));
#25649=CARTESIAN_POINT('Ctrl Pts',(207.451763479567,91.9022376097703,342.2099470813));
#25650=CARTESIAN_POINT('Ctrl Pts',(205.696990550236,91.8397376097703,343.309989738578));
#25651=CARTESIAN_POINT('Ctrl Pts',(203.942217620905,91.7772376097703,344.410032395856));
#25652=CARTESIAN_POINT('Ctrl Pts',(201.923558160576,91.7147376097703,343.947068180639));
#25653=CARTESIAN_POINT('Ctrl Pts',(199.904898700248,91.6522376097703,343.484103965422));
#25654=CARTESIAN_POINT('Ctrl Pts',(198.80485604297,91.5897376097703,341.72933103609));
#25655=CARTESIAN_POINT('Ctrl Pts',(197.704813385692,91.5272376097703,339.974558106759));
#25656=CARTESIAN_POINT('Ctrl Pts',(198.167777600909,91.4647376097703,337.955898646431));
#25657=CARTESIAN_POINT('Ctrl Pts',(198.630741816126,91.4022376097703,335.937239186102));
#25658=CARTESIAN_POINT('Ctrl Pts',(200.385514745457,91.3397376097703,334.837196528824));
#25659=CARTESIAN_POINT('Ctrl Pts',(202.140287674788,91.2772376097703,333.737153871546));
#25660=CARTESIAN_POINT('Ctrl Pts',(204.158947135117,91.2147376097703,334.200118086763));
#25661=CARTESIAN_POINT('Ctrl Pts',(206.177606595445,91.1522376097703,334.66308230198));
#25662=CARTESIAN_POINT('Ctrl Pts',(207.277649252723,91.0897376097703,336.417855231311));
#25663=CARTESIAN_POINT('Ctrl Pts',(208.377691910001,91.0272376097703,338.172628160643));
#25664=CARTESIAN_POINT('Ctrl Pts',(207.914727694784,90.9647376097703,340.191287620971));
#25665=CARTESIAN_POINT('Ctrl Pts',(207.451763479567,90.9022376097703,342.2099470813));
#25666=CARTESIAN_POINT('Ctrl Pts',(205.696990550236,90.8397376097703,343.309989738578));
#25667=CARTESIAN_POINT('Ctrl Pts',(203.942217620905,90.7772376097703,344.410032395856));
#25668=CARTESIAN_POINT('Ctrl Pts',(201.923558160576,90.7147376097703,343.947068180639));
#25669=CARTESIAN_POINT('Ctrl Pts',(199.904898700248,90.6522376097703,343.484103965422));
#25670=CARTESIAN_POINT('Ctrl Pts',(198.80485604297,90.5897376097703,341.72933103609));
#25671=CARTESIAN_POINT('Ctrl Pts',(197.704813385692,90.5272376097703,339.974558106759));
#25672=CARTESIAN_POINT('Ctrl Pts',(198.167777600909,90.4647376097703,337.955898646431));
#25673=CARTESIAN_POINT('Ctrl Pts',(198.630741816126,90.4022376097703,335.937239186102));
#25674=CARTESIAN_POINT('Ctrl Pts',(200.385514745457,90.3397376097703,334.837196528824));
#25675=CARTESIAN_POINT('Ctrl Pts',(202.140287674788,90.2772376097703,333.737153871546));
#25676=CARTESIAN_POINT('Ctrl Pts',(204.158947135117,90.2147376097703,334.200118086763));
#25677=CARTESIAN_POINT('Ctrl Pts',(206.177606595445,90.1522376097703,334.66308230198));
#25678=CARTESIAN_POINT('Ctrl Pts',(207.277649252723,90.0897376097703,336.417855231311));
#25679=CARTESIAN_POINT('Ctrl Pts',(208.377691910001,90.0272376097703,338.172628160643));
#25680=CARTESIAN_POINT('Ctrl Pts',(207.914727694784,89.9647376097703,340.191287620971));
#25681=CARTESIAN_POINT('Ctrl Pts',(207.451763479567,89.9022376097703,342.2099470813));
#25682=CARTESIAN_POINT('Ctrl Pts',(205.696990550236,89.8397376097703,343.309989738578));
#25683=CARTESIAN_POINT('Ctrl Pts',(203.942217620905,89.7772376097703,344.410032395856));
#25684=CARTESIAN_POINT('Ctrl Pts',(201.923558160576,89.7147376097703,343.947068180639));
#25685=CARTESIAN_POINT('Ctrl Pts',(199.904898700248,89.6522376097703,343.484103965422));
#25686=CARTESIAN_POINT('Ctrl Pts',(198.80485604297,89.5897376097703,341.72933103609));
#25687=CARTESIAN_POINT('Ctrl Pts',(197.704813385692,89.5272376097703,339.974558106759));
#25688=CARTESIAN_POINT('Ctrl Pts',(198.167777600909,89.4647376097703,337.955898646431));
#25689=CARTESIAN_POINT('Ctrl Pts',(198.630741816126,89.4022376097703,335.937239186102));
#25690=CARTESIAN_POINT('Ctrl Pts',(200.385514745457,89.3397376097703,334.837196528824));
#25691=CARTESIAN_POINT('Ctrl Pts',(202.140287674788,89.2772376097703,333.737153871546));
#25692=CARTESIAN_POINT('Ctrl Pts',(204.158947135117,89.2147376097703,334.200118086763));
#25693=CARTESIAN_POINT('Ctrl Pts',(206.177606595445,89.1522376097703,334.66308230198));
#25694=CARTESIAN_POINT('Ctrl Pts',(207.277649252723,89.0897376097703,336.417855231311));
#25695=CARTESIAN_POINT('Ctrl Pts',(208.377691910001,89.0272376097703,338.172628160643));
#25696=CARTESIAN_POINT('Ctrl Pts',(207.914727694784,88.9647376097703,340.191287620971));
#25697=CARTESIAN_POINT('Ctrl Pts',(207.451763479567,88.9022376097703,342.2099470813));
#25698=CARTESIAN_POINT('Ctrl Pts',(205.696990550236,88.8397376097703,343.309989738578));
#25699=CARTESIAN_POINT('Ctrl Pts',(203.942217620905,88.7772376097703,344.410032395856));
#25700=CARTESIAN_POINT('Ctrl Pts',(201.923558160576,88.7147376097703,343.947068180639));
#25701=CARTESIAN_POINT('Ctrl Pts',(199.904898700248,88.6522376097703,343.484103965422));
#25702=CARTESIAN_POINT('Ctrl Pts',(198.80485604297,88.5897376097703,341.72933103609));
#25703=CARTESIAN_POINT('Ctrl Pts',(197.704813385692,88.5272376097703,339.974558106759));
#25704=CARTESIAN_POINT('Ctrl Pts',(198.167777600909,88.4647376097703,337.955898646431));
#25705=CARTESIAN_POINT('Ctrl Pts',(198.630741816126,88.4022376097703,335.937239186102));
#25706=CARTESIAN_POINT('Ctrl Pts',(200.385514745457,88.3397376097703,334.837196528824));
#25707=CARTESIAN_POINT('Ctrl Pts',(202.140287674788,88.2772376097703,333.737153871546));
#25708=CARTESIAN_POINT('Ctrl Pts',(204.158947135117,88.2147376097703,334.200118086763));
#25709=CARTESIAN_POINT('Ctrl Pts',(206.177606595445,88.1522376097703,334.66308230198));
#25710=CARTESIAN_POINT('Ctrl Pts',(207.277649252723,88.0897376097703,336.417855231311));
#25711=CARTESIAN_POINT('Ctrl Pts',(208.377691910001,88.0272376097703,338.172628160643));
#25712=CARTESIAN_POINT('Ctrl Pts',(207.914727694784,87.9647376097703,340.191287620971));
#25713=CARTESIAN_POINT('Ctrl Pts',(207.451763479567,87.9022376097703,342.2099470813));
#25714=CARTESIAN_POINT('Ctrl Pts',(205.696990550236,87.8397376097703,343.309989738578));
#25715=CARTESIAN_POINT('Ctrl Pts',(203.942217620905,87.7772376097703,344.410032395856));
#25716=CARTESIAN_POINT('Ctrl Pts',(201.923558160576,87.7147376097703,343.947068180639));
#25717=CARTESIAN_POINT('Ctrl Pts',(199.904898700248,87.6522376097703,343.484103965422));
#25718=CARTESIAN_POINT('Ctrl Pts',(198.80485604297,87.5897376097703,341.72933103609));
#25719=CARTESIAN_POINT('Ctrl Pts',(197.704813385692,87.5272376097703,339.974558106759));
#25720=CARTESIAN_POINT('Ctrl Pts',(198.167777600909,87.4647376097703,337.955898646431));
#25721=CARTESIAN_POINT('Ctrl Pts',(198.630741816126,87.4022376097703,335.937239186102));
#25722=CARTESIAN_POINT('Ctrl Pts',(200.385514745457,87.3397376097703,334.837196528824));
#25723=CARTESIAN_POINT('Ctrl Pts',(202.140287674788,87.2772376097703,333.737153871546));
#25724=CARTESIAN_POINT('Ctrl Pts',(204.158947135117,87.2147376097703,334.200118086763));
#25725=CARTESIAN_POINT('Ctrl Pts',(204.03795315819,101.527237608405,334.727687233877));
#25726=CARTESIAN_POINT('Ctrl Pts',(205.838086322694,101.464737608405,335.140534102886));
#25727=CARTESIAN_POINT('Ctrl Pts',(206.819045869686,101.402237608405,336.705347291213));
#25728=CARTESIAN_POINT('Ctrl Pts',(207.800005416678,101.339737608405,338.27016047954));
#25729=CARTESIAN_POINT('Ctrl Pts',(207.38715854767,101.277237608405,340.070293644044));
#25730=CARTESIAN_POINT('Ctrl Pts',(206.974311678662,101.214737608405,341.870426808548));
#25731=CARTESIAN_POINT('Ctrl Pts',(205.409498490334,101.152237608405,342.851386355541));
#25732=CARTESIAN_POINT('Ctrl Pts',(203.844685302007,101.089737608405,343.832345902533));
#25733=CARTESIAN_POINT('Ctrl Pts',(202.044552137503,101.027237608405,343.419499033524));
#25734=CARTESIAN_POINT('Ctrl Pts',(200.244418972999,100.964737608405,343.006652164516));
#25735=CARTESIAN_POINT('Ctrl Pts',(199.263459426007,100.902237608405,341.441838976189));
#25736=CARTESIAN_POINT('Ctrl Pts',(198.282499879015,100.839737608405,339.877025787862));
#25737=CARTESIAN_POINT('Ctrl Pts',(198.695346748023,100.777237608405,338.076892623358));
#25738=CARTESIAN_POINT('Ctrl Pts',(199.108193617031,100.714737608405,336.276759458854));
#25739=CARTESIAN_POINT('Ctrl Pts',(200.673006805358,100.652237608405,335.295799911861));
#25740=CARTESIAN_POINT('Ctrl Pts',(202.237819993686,100.589737608405,334.314840364869));
#25741=CARTESIAN_POINT('Ctrl Pts',(204.03795315819,100.527237608405,334.727687233877));
#25742=CARTESIAN_POINT('Ctrl Pts',(205.838086322694,100.464737608405,335.140534102886));
#25743=CARTESIAN_POINT('Ctrl Pts',(206.819045869686,100.402237608405,336.705347291213));
#25744=CARTESIAN_POINT('Ctrl Pts',(207.800005416678,100.339737608405,338.27016047954));
#25745=CARTESIAN_POINT('Ctrl Pts',(207.38715854767,100.277237608405,340.070293644044));
#25746=CARTESIAN_POINT('Ctrl Pts',(206.974311678662,100.214737608405,341.870426808548));
#25747=CARTESIAN_POINT('Ctrl Pts',(205.409498490334,100.152237608405,342.851386355541));
#25748=CARTESIAN_POINT('Ctrl Pts',(203.844685302007,100.089737608405,343.832345902533));
#25749=CARTESIAN_POINT('Ctrl Pts',(202.044552137503,100.027237608405,343.419499033524));
#25750=CARTESIAN_POINT('Ctrl Pts',(200.244418972999,99.9647376084047,343.006652164516));
#25751=CARTESIAN_POINT('Ctrl Pts',(199.263459426007,99.9022376084047,341.441838976189));
#25752=CARTESIAN_POINT('Ctrl Pts',(198.282499879015,99.8397376084047,339.877025787862));
#25753=CARTESIAN_POINT('Ctrl Pts',(198.695346748023,99.7772376084047,338.076892623358));
#25754=CARTESIAN_POINT('Ctrl Pts',(199.108193617031,99.7147376084047,336.276759458854));
#25755=CARTESIAN_POINT('Ctrl Pts',(200.673006805358,99.6522376084047,335.295799911861));
#25756=CARTESIAN_POINT('Ctrl Pts',(202.237819993686,99.5897376084047,334.314840364869));
#25757=CARTESIAN_POINT('Ctrl Pts',(204.03795315819,99.5272376084047,334.727687233877));
#25758=CARTESIAN_POINT('Ctrl Pts',(205.838086322694,99.4647376084047,335.140534102886));
#25759=CARTESIAN_POINT('Ctrl Pts',(206.819045869686,99.4022376084047,336.705347291213));
#25760=CARTESIAN_POINT('Ctrl Pts',(207.800005416678,99.3397376084047,338.27016047954));
#25761=CARTESIAN_POINT('Ctrl Pts',(207.38715854767,99.2772376084047,340.070293644044));
#25762=CARTESIAN_POINT('Ctrl Pts',(206.974311678662,99.2147376084047,341.870426808548));
#25763=CARTESIAN_POINT('Ctrl Pts',(205.409498490334,99.1522376084047,342.851386355541));
#25764=CARTESIAN_POINT('Ctrl Pts',(203.844685302007,99.0897376084047,343.832345902533));
#25765=CARTESIAN_POINT('Ctrl Pts',(202.044552137503,99.0272376084047,343.419499033524));
#25766=CARTESIAN_POINT('Ctrl Pts',(200.244418972999,98.9647376084047,343.006652164516));
#25767=CARTESIAN_POINT('Ctrl Pts',(199.263459426007,98.9022376084047,341.441838976189));
#25768=CARTESIAN_POINT('Ctrl Pts',(198.282499879015,98.8397376084047,339.877025787862));
#25769=CARTESIAN_POINT('Ctrl Pts',(198.695346748023,98.7772376084047,338.076892623358));
#25770=CARTESIAN_POINT('Ctrl Pts',(199.108193617031,98.7147376084047,336.276759458854));
#25771=CARTESIAN_POINT('Ctrl Pts',(200.673006805358,98.6522376084047,335.295799911861));
#25772=CARTESIAN_POINT('Ctrl Pts',(202.237819993686,98.5897376084047,334.314840364869));
#25773=CARTESIAN_POINT('Ctrl Pts',(204.03795315819,98.5272376084047,334.727687233877));
#25774=CARTESIAN_POINT('Ctrl Pts',(205.838086322694,98.4647376084047,335.140534102886));
#25775=CARTESIAN_POINT('Ctrl Pts',(206.819045869686,98.4022376084047,336.705347291213));
#25776=CARTESIAN_POINT('Ctrl Pts',(207.800005416678,98.3397376084047,338.27016047954));
#25777=CARTESIAN_POINT('Ctrl Pts',(207.38715854767,98.2772376084047,340.070293644044));
#25778=CARTESIAN_POINT('Ctrl Pts',(206.974311678662,98.2147376084047,341.870426808548));
#25779=CARTESIAN_POINT('Ctrl Pts',(205.409498490334,98.1522376084047,342.851386355541));
#25780=CARTESIAN_POINT('Ctrl Pts',(203.844685302007,98.0897376084047,343.832345902533));
#25781=CARTESIAN_POINT('Ctrl Pts',(202.044552137503,98.0272376084047,343.419499033524));
#25782=CARTESIAN_POINT('Ctrl Pts',(200.244418972999,97.9647376084047,343.006652164516));
#25783=CARTESIAN_POINT('Ctrl Pts',(199.263459426007,97.9022376084047,341.441838976189));
#25784=CARTESIAN_POINT('Ctrl Pts',(198.282499879015,97.8397376084047,339.877025787862));
#25785=CARTESIAN_POINT('Ctrl Pts',(198.695346748023,97.7772376084047,338.076892623358));
#25786=CARTESIAN_POINT('Ctrl Pts',(199.108193617031,97.7147376084047,336.276759458854));
#25787=CARTESIAN_POINT('Ctrl Pts',(200.673006805358,97.6522376084047,335.295799911861));
#25788=CARTESIAN_POINT('Ctrl Pts',(202.237819993686,97.5897376084047,334.314840364869));
#25789=CARTESIAN_POINT('Ctrl Pts',(204.03795315819,97.5272376084047,334.727687233877));
#25790=CARTESIAN_POINT('Ctrl Pts',(205.838086322694,97.4647376084047,335.140534102886));
#25791=CARTESIAN_POINT('Ctrl Pts',(206.819045869686,97.4022376084047,336.705347291213));
#25792=CARTESIAN_POINT('Ctrl Pts',(207.800005416678,97.3397376084047,338.27016047954));
#25793=CARTESIAN_POINT('Ctrl Pts',(207.38715854767,97.2772376084047,340.070293644044));
#25794=CARTESIAN_POINT('Ctrl Pts',(206.974311678662,97.2147376084047,341.870426808548));
#25795=CARTESIAN_POINT('Ctrl Pts',(205.409498490334,97.1522376084047,342.851386355541));
#25796=CARTESIAN_POINT('Ctrl Pts',(203.844685302007,97.0897376084047,343.832345902533));
#25797=CARTESIAN_POINT('Ctrl Pts',(202.044552137503,97.0272376084047,343.419499033524));
#25798=CARTESIAN_POINT('Ctrl Pts',(200.244418972999,96.9647376084047,343.006652164516));
#25799=CARTESIAN_POINT('Ctrl Pts',(199.263459426007,96.9022376084047,341.441838976189));
#25800=CARTESIAN_POINT('Ctrl Pts',(198.282499879015,96.8397376084047,339.877025787862));
#25801=CARTESIAN_POINT('Ctrl Pts',(198.695346748023,96.7772376084047,338.076892623358));
#25802=CARTESIAN_POINT('Ctrl Pts',(199.108193617031,96.7147376084047,336.276759458854));
#25803=CARTESIAN_POINT('Ctrl Pts',(200.673006805358,96.6522376084047,335.295799911861));
#25804=CARTESIAN_POINT('Ctrl Pts',(202.237819993686,96.5897376084047,334.314840364869));
#25805=CARTESIAN_POINT('Ctrl Pts',(204.03795315819,96.5272376084047,334.727687233877));
#25806=CARTESIAN_POINT('Ctrl Pts',(205.838086322694,96.4647376084047,335.140534102886));
#25807=CARTESIAN_POINT('Ctrl Pts',(206.819045869686,96.4022376084047,336.705347291213));
#25808=CARTESIAN_POINT('Ctrl Pts',(207.800005416678,96.3397376084047,338.27016047954));
#25809=CARTESIAN_POINT('Ctrl Pts',(207.38715854767,96.2772376084047,340.070293644044));
#25810=CARTESIAN_POINT('Ctrl Pts',(206.974311678662,96.2147376084047,341.870426808548));
#25811=CARTESIAN_POINT('Ctrl Pts',(205.409498490334,96.1522376084047,342.851386355541));
#25812=CARTESIAN_POINT('Ctrl Pts',(203.844685302007,96.0897376084047,343.832345902533));
#25813=CARTESIAN_POINT('Ctrl Pts',(202.044552137503,96.0272376084047,343.419499033524));
#25814=CARTESIAN_POINT('Ctrl Pts',(200.244418972999,95.9647376084047,343.006652164516));
#25815=CARTESIAN_POINT('Ctrl Pts',(199.263459426007,95.9022376084047,341.441838976189));
#25816=CARTESIAN_POINT('Ctrl Pts',(198.282499879015,95.8397376084047,339.877025787862));
#25817=CARTESIAN_POINT('Ctrl Pts',(198.695346748023,95.7772376084047,338.076892623358));
#25818=CARTESIAN_POINT('Ctrl Pts',(199.108193617031,95.7147376084047,336.276759458854));
#25819=CARTESIAN_POINT('Ctrl Pts',(200.673006805358,95.6522376084047,335.295799911861));
#25820=CARTESIAN_POINT('Ctrl Pts',(202.237819993686,95.5897376084047,334.314840364869));
#25821=CARTESIAN_POINT('Ctrl Pts',(204.03795315819,95.5272376084047,334.727687233877));
#25822=CARTESIAN_POINT('Ctrl Pts',(205.838086322694,95.4647376084047,335.140534102886));
#25823=CARTESIAN_POINT('Ctrl Pts',(206.819045869686,95.4022376084047,336.705347291213));
#25824=CARTESIAN_POINT('Ctrl Pts',(207.800005416678,95.3397376084047,338.27016047954));
#25825=CARTESIAN_POINT('Ctrl Pts',(207.38715854767,95.2772376084047,340.070293644044));
#25826=CARTESIAN_POINT('Ctrl Pts',(206.974311678662,95.2147376084047,341.870426808548));
#25827=CARTESIAN_POINT('Ctrl Pts',(205.409498490334,95.1522376084047,342.851386355541));
#25828=CARTESIAN_POINT('Ctrl Pts',(203.844685302007,95.0897376084047,343.832345902533));
#25829=CARTESIAN_POINT('Ctrl Pts',(202.044552137503,95.0272376084047,343.419499033524));
#25830=CARTESIAN_POINT('Ctrl Pts',(200.244418972999,94.9647376084047,343.006652164516));
#25831=CARTESIAN_POINT('Ctrl Pts',(199.263459426007,94.9022376084047,341.441838976189));
#25832=CARTESIAN_POINT('Ctrl Pts',(198.282499879015,94.8397376084047,339.877025787862));
#25833=CARTESIAN_POINT('Ctrl Pts',(198.695346748023,94.7772376084047,338.076892623358));
#25834=CARTESIAN_POINT('Ctrl Pts',(199.108193617031,94.7147376084047,336.276759458854));
#25835=CARTESIAN_POINT('Ctrl Pts',(200.673006805358,94.6522376084047,335.295799911861));
#25836=CARTESIAN_POINT('Ctrl Pts',(202.237819993686,94.5897376084047,334.314840364869));
#25837=CARTESIAN_POINT('Ctrl Pts',(204.03795315819,94.5272376084047,334.727687233877));
#25838=CARTESIAN_POINT('Ctrl Pts',(205.838086322694,94.4647376084047,335.140534102886));
#25839=CARTESIAN_POINT('Ctrl Pts',(206.819045869686,94.4022376084047,336.705347291213));
#25840=CARTESIAN_POINT('Ctrl Pts',(207.800005416678,94.3397376084047,338.27016047954));
#25841=CARTESIAN_POINT('Ctrl Pts',(207.38715854767,94.2772376084047,340.070293644044));
#25842=CARTESIAN_POINT('Ctrl Pts',(206.974311678662,94.2147376084047,341.870426808548));
#25843=CARTESIAN_POINT('Ctrl Pts',(205.409498490334,94.1522376084047,342.851386355541));
#25844=CARTESIAN_POINT('Ctrl Pts',(203.844685302007,94.0897376084047,343.832345902533));
#25845=CARTESIAN_POINT('Ctrl Pts',(202.044552137503,94.0272376084047,343.419499033524));
#25846=CARTESIAN_POINT('Ctrl Pts',(200.244418972999,93.9647376084047,343.006652164516));
#25847=CARTESIAN_POINT('Ctrl Pts',(199.263459426007,93.9022376084047,341.441838976189));
#25848=CARTESIAN_POINT('Ctrl Pts',(198.282499879015,93.8397376084047,339.877025787862));
#25849=CARTESIAN_POINT('Ctrl Pts',(198.695346748023,93.7772376084047,338.076892623358));
#25850=CARTESIAN_POINT('Ctrl Pts',(199.108193617031,93.7147376084047,336.276759458854));
#25851=CARTESIAN_POINT('Ctrl Pts',(200.673006805358,93.6522376084047,335.295799911861));
#25852=CARTESIAN_POINT('Ctrl Pts',(202.237819993686,93.5897376084047,334.314840364869));
#25853=CARTESIAN_POINT('Ctrl Pts',(204.03795315819,93.5272376084047,334.727687233877));
#25854=CARTESIAN_POINT('Ctrl Pts',(205.838086322694,93.4647376084047,335.140534102886));
#25855=CARTESIAN_POINT('Ctrl Pts',(206.819045869686,93.4022376084047,336.705347291213));
#25856=CARTESIAN_POINT('Ctrl Pts',(207.800005416678,93.3397376084047,338.27016047954));
#25857=CARTESIAN_POINT('Ctrl Pts',(207.38715854767,93.2772376084047,340.070293644044));
#25858=CARTESIAN_POINT('Ctrl Pts',(206.974311678662,93.2147376084047,341.870426808548));
#25859=CARTESIAN_POINT('Ctrl Pts',(205.409498490334,93.1522376084047,342.851386355541));
#25860=CARTESIAN_POINT('Ctrl Pts',(203.844685302007,93.0897376084047,343.832345902533));
#25861=CARTESIAN_POINT('Ctrl Pts',(202.044552137503,93.0272376084047,343.419499033524));
#25862=CARTESIAN_POINT('Ctrl Pts',(200.244418972999,92.9647376084047,343.006652164516));
#25863=CARTESIAN_POINT('Ctrl Pts',(199.263459426007,92.9022376084047,341.441838976189));
#25864=CARTESIAN_POINT('Ctrl Pts',(198.282499879015,92.8397376084047,339.877025787862));
#25865=CARTESIAN_POINT('Ctrl Pts',(198.695346748023,92.7772376084047,338.076892623358));
#25866=CARTESIAN_POINT('Ctrl Pts',(199.108193617031,92.7147376084047,336.276759458854));
#25867=CARTESIAN_POINT('Ctrl Pts',(200.673006805358,92.6522376084047,335.295799911861));
#25868=CARTESIAN_POINT('Ctrl Pts',(202.237819993686,92.5897376084047,334.314840364869));
#25869=CARTESIAN_POINT('Ctrl Pts',(204.03795315819,92.5272376084047,334.727687233877));
#25870=CARTESIAN_POINT('Ctrl Pts',(205.838086322694,92.4647376084047,335.140534102886));
#25871=CARTESIAN_POINT('Ctrl Pts',(206.819045869686,92.4022376084047,336.705347291213));
#25872=CARTESIAN_POINT('Ctrl Pts',(207.800005416678,92.3397376084047,338.27016047954));
#25873=CARTESIAN_POINT('Ctrl Pts',(207.38715854767,92.2772376084047,340.070293644044));
#25874=CARTESIAN_POINT('Ctrl Pts',(206.974311678662,92.2147376084047,341.870426808548));
#25875=CARTESIAN_POINT('Ctrl Pts',(205.409498490334,92.1522376084047,342.851386355541));
#25876=CARTESIAN_POINT('Ctrl Pts',(203.844685302007,92.0897376084047,343.832345902533));
#25877=CARTESIAN_POINT('Ctrl Pts',(202.044552137503,92.0272376084047,343.419499033524));
#25878=CARTESIAN_POINT('Ctrl Pts',(200.244418972999,91.9647376084047,343.006652164516));
#25879=CARTESIAN_POINT('Ctrl Pts',(199.263459426007,91.9022376084047,341.441838976189));
#25880=CARTESIAN_POINT('Ctrl Pts',(198.282499879015,91.8397376084047,339.877025787862));
#25881=CARTESIAN_POINT('Ctrl Pts',(198.695346748023,91.7772376084047,338.076892623358));
#25882=CARTESIAN_POINT('Ctrl Pts',(199.108193617031,91.7147376084047,336.276759458854));
#25883=CARTESIAN_POINT('Ctrl Pts',(200.673006805358,91.6522376084047,335.295799911861));
#25884=CARTESIAN_POINT('Ctrl Pts',(202.237819993686,91.5897376084047,334.314840364869));
#25885=CARTESIAN_POINT('Ctrl Pts',(204.03795315819,91.5272376084047,334.727687233877));
#25886=CARTESIAN_POINT('Ctrl Pts',(205.838086322694,91.4647376084047,335.140534102886));
#25887=CARTESIAN_POINT('Ctrl Pts',(206.819045869686,91.4022376084047,336.705347291213));
#25888=CARTESIAN_POINT('Ctrl Pts',(207.800005416678,91.3397376084047,338.27016047954));
#25889=CARTESIAN_POINT('Ctrl Pts',(207.38715854767,91.2772376084047,340.070293644044));
#25890=CARTESIAN_POINT('Ctrl Pts',(206.974311678662,91.2147376084047,341.870426808548));
#25891=CARTESIAN_POINT('Ctrl Pts',(205.409498490334,91.1522376084047,342.851386355541));
#25892=CARTESIAN_POINT('Ctrl Pts',(203.844685302007,91.0897376084047,343.832345902533));
#25893=CARTESIAN_POINT('Ctrl Pts',(202.044552137503,91.0272376084047,343.419499033524));
#25894=CARTESIAN_POINT('Ctrl Pts',(200.244418972999,90.9647376084047,343.006652164516));
#25895=CARTESIAN_POINT('Ctrl Pts',(199.263459426007,90.9022376084047,341.441838976189));
#25896=CARTESIAN_POINT('Ctrl Pts',(198.282499879015,90.8397376084047,339.877025787862));
#25897=CARTESIAN_POINT('Ctrl Pts',(198.695346748023,90.7772376084047,338.076892623358));
#25898=CARTESIAN_POINT('Ctrl Pts',(199.108193617031,90.7147376084047,336.276759458854));
#25899=CARTESIAN_POINT('Ctrl Pts',(200.673006805358,90.6522376084047,335.295799911861));
#25900=CARTESIAN_POINT('Ctrl Pts',(202.237819993686,90.5897376084047,334.314840364869));
#25901=CARTESIAN_POINT('Ctrl Pts',(204.03795315819,90.5272376084047,334.727687233877));
#25902=CARTESIAN_POINT('Ctrl Pts',(205.838086322694,90.4647376084047,335.140534102886));
#25903=CARTESIAN_POINT('Ctrl Pts',(206.819045869686,90.4022376084047,336.705347291213));
#25904=CARTESIAN_POINT('Ctrl Pts',(207.800005416678,90.3397376084047,338.27016047954));
#25905=CARTESIAN_POINT('Ctrl Pts',(207.38715854767,90.2772376084047,340.070293644044));
#25906=CARTESIAN_POINT('Ctrl Pts',(206.974311678662,90.2147376084047,341.870426808548));
#25907=CARTESIAN_POINT('Ctrl Pts',(205.409498490334,90.1522376084047,342.851386355541));
#25908=CARTESIAN_POINT('Ctrl Pts',(203.844685302007,90.0897376084047,343.832345902533));
#25909=CARTESIAN_POINT('Ctrl Pts',(202.044552137503,90.0272376084047,343.419499033524));
#25910=CARTESIAN_POINT('Ctrl Pts',(200.244418972999,89.9647376084047,343.006652164516));
#25911=CARTESIAN_POINT('Ctrl Pts',(199.263459426007,89.9022376084047,341.441838976189));
#25912=CARTESIAN_POINT('Ctrl Pts',(198.282499879015,89.8397376084047,339.877025787862));
#25913=CARTESIAN_POINT('Ctrl Pts',(198.695346748023,89.7772376084047,338.076892623358));
#25914=CARTESIAN_POINT('Ctrl Pts',(199.108193617031,89.7147376084047,336.276759458854));
#25915=CARTESIAN_POINT('Ctrl Pts',(200.673006805358,89.6522376084047,335.295799911861));
#25916=CARTESIAN_POINT('Ctrl Pts',(202.237819993686,89.5897376084047,334.314840364869));
#25917=CARTESIAN_POINT('Ctrl Pts',(204.03795315819,89.5272376084047,334.727687233877));
#25918=CARTESIAN_POINT('Ctrl Pts',(205.838086322694,89.4647376084047,335.140534102886));
#25919=CARTESIAN_POINT('Ctrl Pts',(206.819045869686,89.4022376084047,336.705347291213));
#25920=CARTESIAN_POINT('Ctrl Pts',(207.800005416678,89.3397376084047,338.27016047954));
#25921=CARTESIAN_POINT('Ctrl Pts',(207.38715854767,89.2772376084047,340.070293644044));
#25922=CARTESIAN_POINT('Ctrl Pts',(206.974311678662,89.2147376084047,341.870426808548));
#25923=CARTESIAN_POINT('Ctrl Pts',(205.409498490334,89.1522376084047,342.851386355541));
#25924=CARTESIAN_POINT('Ctrl Pts',(203.844685302007,89.0897376084047,343.832345902533));
#25925=CARTESIAN_POINT('Ctrl Pts',(202.044552137503,89.0272376084047,343.419499033524));
#25926=CARTESIAN_POINT('Ctrl Pts',(200.244418972999,88.9647376084047,343.006652164516));
#25927=CARTESIAN_POINT('Ctrl Pts',(199.263459426007,88.9022376084047,341.441838976189));
#25928=CARTESIAN_POINT('Ctrl Pts',(198.282499879015,88.8397376084047,339.877025787862));
#25929=CARTESIAN_POINT('Ctrl Pts',(198.695346748023,88.7772376084047,338.076892623358));
#25930=CARTESIAN_POINT('Ctrl Pts',(199.108193617031,88.7147376084047,336.276759458854));
#25931=CARTESIAN_POINT('Ctrl Pts',(200.673006805358,88.6522376084047,335.295799911861));
#25932=CARTESIAN_POINT('Ctrl Pts',(202.237819993686,88.5897376084047,334.314840364869));
#25933=CARTESIAN_POINT('Ctrl Pts',(204.03795315819,88.5272376084047,334.727687233877));
#25934=CARTESIAN_POINT('Ctrl Pts',(205.838086322694,88.4647376084047,335.140534102886));
#25935=CARTESIAN_POINT('Ctrl Pts',(206.819045869686,88.4022376084047,336.705347291213));
#25936=CARTESIAN_POINT('Ctrl Pts',(207.800005416678,88.3397376084047,338.27016047954));
#25937=CARTESIAN_POINT('Ctrl Pts',(207.38715854767,88.2772376084047,340.070293644044));
#25938=CARTESIAN_POINT('Ctrl Pts',(206.974311678662,88.2147376084047,341.870426808548));
#25939=CARTESIAN_POINT('Ctrl Pts',(205.409498490334,88.1522376084047,342.851386355541));
#25940=CARTESIAN_POINT('Ctrl Pts',(203.844685302007,88.0897376084047,343.832345902533));
#25941=CARTESIAN_POINT('Ctrl Pts',(202.044552137503,88.0272376084047,343.419499033524));
#25942=CARTESIAN_POINT('Ctrl Pts',(200.244418972999,87.9647376084047,343.006652164516));
#25943=CARTESIAN_POINT('Ctrl Pts',(199.263459426007,87.9022376084047,341.441838976189));
#25944=CARTESIAN_POINT('Ctrl Pts',(198.282499879015,87.8397376084047,339.877025787862));
#25945=CARTESIAN_POINT('Ctrl Pts',(198.695346748023,87.7772376084047,338.076892623358));
#25946=CARTESIAN_POINT('Ctrl Pts',(199.108193617031,87.7147376084047,336.276759458854));
#25947=CARTESIAN_POINT('Ctrl Pts',(200.673006805358,87.6522376084047,335.295799911861));
#25948=CARTESIAN_POINT('Ctrl Pts',(202.237819993686,87.5897376084047,334.314840364869));
#25949=CARTESIAN_POINT('Ctrl Pts',(204.03795315819,87.5272376084047,334.727687233877));
#25950=CARTESIAN_POINT('Origin',(224.770541810138,65.2397376070391,333.797420988906));
#25951=CARTESIAN_POINT('Origin',(220.299763861057,65.2397376070391,353.291321176658));
#25952=CARTESIAN_POINT('Origin',(220.299763861057,65.2397376070391,353.291321176658));
#25953=CARTESIAN_POINT('Origin',(224.770541810138,65.2397376070391,333.797420988906));
#25954=CARTESIAN_POINT('Origin',(203.041252647848,99.3647376084047,339.073593133703));
#25955=CARTESIAN_POINT('',(208.562910255543,96.8022376084046,339.539344956919));
#25956=CARTESIAN_POINT('',(208.562910255543,96.9272376084047,339.539344956919));
#25957=CARTESIAN_POINT('',(208.562910255543,99.3647376084047,339.539344956919));
#25958=CARTESIAN_POINT('',(204.724000912662,97.739737607039,344.353175103396));
#25959=CARTESIAN_POINT('Ctrl Pts',(204.724000912662,97.739737607039,344.353175103396));
#25960=CARTESIAN_POINT('Ctrl Pts',(203.673826787241,97.7072511661896,344.687894537141));
#25961=CARTESIAN_POINT('Ctrl Pts',(202.575500824633,97.6772376084047,344.595250741398));
#25962=CARTESIAN_POINT('Ctrl Pts',(200.288355356745,97.6147376084047,344.402330019522));
#25963=CARTESIAN_POINT('Ctrl Pts',(198.807514837511,97.5522376084047,342.648658398949));
#25964=CARTESIAN_POINT('Ctrl Pts',(197.326674318278,97.4897376084047,340.894986778376));
#25965=CARTESIAN_POINT('Ctrl Pts',(197.519595040153,97.4272376084047,338.607841310488));
#25966=CARTESIAN_POINT('Ctrl Pts',(197.712515762029,97.3647376084047,336.320695842601));
#25967=CARTESIAN_POINT('Ctrl Pts',(199.466187382602,97.3022376084047,334.839855323367));
#25968=CARTESIAN_POINT('Ctrl Pts',(201.219859003176,97.2397376084047,333.359014804133));
#25969=CARTESIAN_POINT('Ctrl Pts',(203.507004471063,97.1772376084047,333.551935526009));
#25970=CARTESIAN_POINT('Ctrl Pts',(205.794149938951,97.1147376084047,333.744856247885));
#25971=CARTESIAN_POINT('Ctrl Pts',(207.274990458185,97.0522376084047,335.498527868458));
#25972=CARTESIAN_POINT('Ctrl Pts',(208.755830977418,96.9897376084047,337.252199489031));
#25973=CARTESIAN_POINT('Ctrl Pts',(208.562910255543,96.9272376084047,339.539344956919));
#25974=CARTESIAN_POINT('',(207.964363569528,97.739737607039,341.616938637223));
#25975=CARTESIAN_POINT('Origin',(203.041252647847,97.7397376070395,339.073593133703));
#25976=CARTESIAN_POINT('Ctrl Pts',(207.964363569528,97.7397376070391,341.616938637223));
#25977=CARTESIAN_POINT('Ctrl Pts',(207.458460705412,97.7072511661896,342.596206264131));
#25978=CARTESIAN_POINT('Ctrl Pts',(206.616317913094,97.6772376084047,343.30733094404));
#25979=CARTESIAN_POINT('Ctrl Pts',(204.86264629252,97.6147376084047,344.788171463274));
#25980=CARTESIAN_POINT('Ctrl Pts',(202.575500824633,97.5522376084047,344.595250741398));
#25981=CARTESIAN_POINT('Ctrl Pts',(200.288355356745,97.4897376084047,344.402330019522));
#25982=CARTESIAN_POINT('Ctrl Pts',(198.807514837511,97.4272376084047,342.648658398949));
#25983=CARTESIAN_POINT('Ctrl Pts',(197.326674318278,97.3647376084047,340.894986778376));
#25984=CARTESIAN_POINT('Ctrl Pts',(197.519595040153,97.3022376084047,338.607841310488));
#25985=CARTESIAN_POINT('Ctrl Pts',(197.712515762029,97.2397376084047,336.320695842601));
#25986=CARTESIAN_POINT('Ctrl Pts',(199.466187382602,97.1772376084047,334.839855323367));
#25987=CARTESIAN_POINT('Ctrl Pts',(201.219859003176,97.1147376084047,333.359014804133));
#25988=CARTESIAN_POINT('Ctrl Pts',(203.507004471063,97.0522376084047,333.551935526009));
#25989=CARTESIAN_POINT('Ctrl Pts',(205.794149938951,96.9897376084047,333.744856247885));
#25990=CARTESIAN_POINT('Ctrl Pts',(207.274990458185,96.9272376084047,335.498527868458));
#25991=CARTESIAN_POINT('Ctrl Pts',(208.755830977418,96.8647376084047,337.252199489031));
#25992=CARTESIAN_POINT('Ctrl Pts',(208.562910255543,96.8022376084046,339.539344956919));
#25993=CARTESIAN_POINT('Origin',(203.041252647848,99.3647376084047,339.073593133703));
#25994=CARTESIAN_POINT('',(208.562910255543,95.8022376084047,339.539344956919));
#25995=CARTESIAN_POINT('',(208.562910255543,95.9272376084047,339.539344956919));
#25996=CARTESIAN_POINT('',(208.562910255543,99.3647376084047,339.539344956919));
#25997=CARTESIAN_POINT('Ctrl Pts',(208.562910255543,96.9272376084047,339.539344956919));
#25998=CARTESIAN_POINT('Ctrl Pts',(208.369989533667,96.8647376084047,341.826490424806));
#25999=CARTESIAN_POINT('Ctrl Pts',(206.616317913094,96.8022376084046,343.30733094404));
#26000=CARTESIAN_POINT('Ctrl Pts',(204.86264629252,96.7397376084047,344.788171463274));
#26001=CARTESIAN_POINT('Ctrl Pts',(202.575500824633,96.6772376084047,344.595250741398));
#26002=CARTESIAN_POINT('Ctrl Pts',(200.288355356745,96.6147376084047,344.402330019522));
#26003=CARTESIAN_POINT('Ctrl Pts',(198.807514837511,96.5522376084046,342.648658398949));
#26004=CARTESIAN_POINT('Ctrl Pts',(197.326674318278,96.4897376084047,340.894986778376));
#26005=CARTESIAN_POINT('Ctrl Pts',(197.519595040153,96.4272376084047,338.607841310488));
#26006=CARTESIAN_POINT('Ctrl Pts',(197.712515762029,96.3647376084047,336.320695842601));
#26007=CARTESIAN_POINT('Ctrl Pts',(199.466187382602,96.3022376084047,334.839855323367));
#26008=CARTESIAN_POINT('Ctrl Pts',(201.219859003176,96.2397376084047,333.359014804133));
#26009=CARTESIAN_POINT('Ctrl Pts',(203.507004471063,96.1772376084047,333.551935526009));
#26010=CARTESIAN_POINT('Ctrl Pts',(205.794149938951,96.1147376084047,333.744856247885));
#26011=CARTESIAN_POINT('Ctrl Pts',(207.274990458185,96.0522376084047,335.498527868458));
#26012=CARTESIAN_POINT('Ctrl Pts',(208.755830977418,95.9897376084047,337.252199489031));
#26013=CARTESIAN_POINT('Ctrl Pts',(208.562910255543,95.9272376084047,339.539344956919));
#26014=CARTESIAN_POINT('Ctrl Pts',(208.562910255543,96.8022376084046,339.539344956919));
#26015=CARTESIAN_POINT('Ctrl Pts',(208.369989533667,96.7397376084047,341.826490424806));
#26016=CARTESIAN_POINT('Ctrl Pts',(206.616317913094,96.6772376084047,343.30733094404));
#26017=CARTESIAN_POINT('Ctrl Pts',(204.86264629252,96.6147376084047,344.788171463274));
#26018=CARTESIAN_POINT('Ctrl Pts',(202.575500824633,96.5522376084046,344.595250741398));
#26019=CARTESIAN_POINT('Ctrl Pts',(200.288355356745,96.4897376084047,344.402330019522));
#26020=CARTESIAN_POINT('Ctrl Pts',(198.807514837511,96.4272376084047,342.648658398949));
#26021=CARTESIAN_POINT('Ctrl Pts',(197.326674318278,96.3647376084047,340.894986778376));
#26022=CARTESIAN_POINT('Ctrl Pts',(197.519595040153,96.3022376084047,338.607841310488));
#26023=CARTESIAN_POINT('Ctrl Pts',(197.712515762029,96.2397376084047,336.320695842601));
#26024=CARTESIAN_POINT('Ctrl Pts',(199.466187382602,96.1772376084047,334.839855323367));
#26025=CARTESIAN_POINT('Ctrl Pts',(201.219859003176,96.1147376084047,333.359014804133));
#26026=CARTESIAN_POINT('Ctrl Pts',(203.507004471063,96.0522376084047,333.551935526009));
#26027=CARTESIAN_POINT('Ctrl Pts',(205.794149938951,95.9897376084047,333.744856247885));
#26028=CARTESIAN_POINT('Ctrl Pts',(207.274990458185,95.9272376084047,335.498527868458));
#26029=CARTESIAN_POINT('Ctrl Pts',(208.755830977418,95.8647376084047,337.252199489031));
#26030=CARTESIAN_POINT('Ctrl Pts',(208.562910255543,95.8022376084047,339.539344956919));
#26031=CARTESIAN_POINT('Origin',(203.041252647848,99.3647376084047,339.073593133703));
#26032=CARTESIAN_POINT('',(208.562910255543,94.8022376084047,339.539344956919));
#26033=CARTESIAN_POINT('',(208.562910255543,94.9272376084047,339.539344956919));
#26034=CARTESIAN_POINT('',(208.562910255543,99.3647376084047,339.539344956919));
#26035=CARTESIAN_POINT('Ctrl Pts',(208.562910255543,95.9272376084047,339.539344956919));
#26036=CARTESIAN_POINT('Ctrl Pts',(208.369989533667,95.8647376084047,341.826490424806));
#26037=CARTESIAN_POINT('Ctrl Pts',(206.616317913094,95.8022376084047,343.30733094404));
#26038=CARTESIAN_POINT('Ctrl Pts',(204.86264629252,95.7397376084047,344.788171463274));
#26039=CARTESIAN_POINT('Ctrl Pts',(202.575500824633,95.6772376084046,344.595250741398));
#26040=CARTESIAN_POINT('Ctrl Pts',(200.288355356745,95.6147376084047,344.402330019522));
#26041=CARTESIAN_POINT('Ctrl Pts',(198.807514837511,95.5522376084046,342.648658398949));
#26042=CARTESIAN_POINT('Ctrl Pts',(197.326674318278,95.4897376084047,340.894986778376));
#26043=CARTESIAN_POINT('Ctrl Pts',(197.519595040153,95.4272376084047,338.607841310488));
#26044=CARTESIAN_POINT('Ctrl Pts',(197.712515762029,95.3647376084047,336.320695842601));
#26045=CARTESIAN_POINT('Ctrl Pts',(199.466187382602,95.3022376084047,334.839855323367));
#26046=CARTESIAN_POINT('Ctrl Pts',(201.219859003176,95.2397376084047,333.359014804133));
#26047=CARTESIAN_POINT('Ctrl Pts',(203.507004471063,95.1772376084047,333.551935526009));
#26048=CARTESIAN_POINT('Ctrl Pts',(205.794149938951,95.1147376084047,333.744856247885));
#26049=CARTESIAN_POINT('Ctrl Pts',(207.274990458185,95.0522376084046,335.498527868458));
#26050=CARTESIAN_POINT('Ctrl Pts',(208.755830977418,94.9897376084047,337.252199489031));
#26051=CARTESIAN_POINT('Ctrl Pts',(208.562910255543,94.9272376084047,339.539344956919));
#26052=CARTESIAN_POINT('Ctrl Pts',(208.562910255543,95.8022376084047,339.539344956919));
#26053=CARTESIAN_POINT('Ctrl Pts',(208.369989533667,95.7397376084047,341.826490424806));
#26054=CARTESIAN_POINT('Ctrl Pts',(206.616317913094,95.6772376084046,343.30733094404));
#26055=CARTESIAN_POINT('Ctrl Pts',(204.86264629252,95.6147376084047,344.788171463274));
#26056=CARTESIAN_POINT('Ctrl Pts',(202.575500824633,95.5522376084046,344.595250741398));
#26057=CARTESIAN_POINT('Ctrl Pts',(200.288355356745,95.4897376084047,344.402330019522));
#26058=CARTESIAN_POINT('Ctrl Pts',(198.807514837511,95.4272376084047,342.648658398949));
#26059=CARTESIAN_POINT('Ctrl Pts',(197.326674318278,95.3647376084047,340.894986778376));
#26060=CARTESIAN_POINT('Ctrl Pts',(197.519595040153,95.3022376084046,338.607841310488));
#26061=CARTESIAN_POINT('Ctrl Pts',(197.712515762029,95.2397376084047,336.320695842601));
#26062=CARTESIAN_POINT('Ctrl Pts',(199.466187382602,95.1772376084047,334.839855323367));
#26063=CARTESIAN_POINT('Ctrl Pts',(201.219859003176,95.1147376084047,333.359014804133));
#26064=CARTESIAN_POINT('Ctrl Pts',(203.507004471063,95.0522376084047,333.551935526009));
#26065=CARTESIAN_POINT('Ctrl Pts',(205.794149938951,94.9897376084047,333.744856247885));
#26066=CARTESIAN_POINT('Ctrl Pts',(207.274990458185,94.9272376084047,335.498527868458));
#26067=CARTESIAN_POINT('Ctrl Pts',(208.755830977418,94.8647376084047,337.252199489031));
#26068=CARTESIAN_POINT('Ctrl Pts',(208.562910255543,94.8022376084047,339.539344956919));
#26069=CARTESIAN_POINT('Origin',(203.041252647848,99.3647376084047,339.073593133703));
#26070=CARTESIAN_POINT('',(208.562910255543,93.8022376084047,339.539344956919));
#26071=CARTESIAN_POINT('',(208.562910255543,93.9272376084047,339.539344956919));
#26072=CARTESIAN_POINT('',(208.562910255543,99.3647376084047,339.539344956919));
#26073=CARTESIAN_POINT('Ctrl Pts',(208.562910255543,94.9272376084047,339.539344956919));
#26074=CARTESIAN_POINT('Ctrl Pts',(208.369989533667,94.8647376084047,341.826490424806));
#26075=CARTESIAN_POINT('Ctrl Pts',(206.616317913094,94.8022376084047,343.30733094404));
#26076=CARTESIAN_POINT('Ctrl Pts',(204.86264629252,94.7397376084047,344.788171463274));
#26077=CARTESIAN_POINT('Ctrl Pts',(202.575500824633,94.6772376084047,344.595250741398));
#26078=CARTESIAN_POINT('Ctrl Pts',(200.288355356745,94.6147376084047,344.402330019522));
#26079=CARTESIAN_POINT('Ctrl Pts',(198.807514837511,94.5522376084047,342.648658398949));
#26080=CARTESIAN_POINT('Ctrl Pts',(197.326674318278,94.4897376084047,340.894986778376));
#26081=CARTESIAN_POINT('Ctrl Pts',(197.519595040153,94.4272376084047,338.607841310488));
#26082=CARTESIAN_POINT('Ctrl Pts',(197.712515762029,94.3647376084047,336.320695842601));
#26083=CARTESIAN_POINT('Ctrl Pts',(199.466187382602,94.3022376084047,334.839855323367));
#26084=CARTESIAN_POINT('Ctrl Pts',(201.219859003176,94.2397376084047,333.359014804133));
#26085=CARTESIAN_POINT('Ctrl Pts',(203.507004471063,94.1772376084047,333.551935526009));
#26086=CARTESIAN_POINT('Ctrl Pts',(205.794149938951,94.1147376084047,333.744856247885));
#26087=CARTESIAN_POINT('Ctrl Pts',(207.274990458185,94.0522376084047,335.498527868458));
#26088=CARTESIAN_POINT('Ctrl Pts',(208.755830977418,93.9897376084047,337.252199489031));
#26089=CARTESIAN_POINT('Ctrl Pts',(208.562910255543,93.9272376084047,339.539344956919));
#26090=CARTESIAN_POINT('Ctrl Pts',(208.562910255543,94.8022376084047,339.539344956919));
#26091=CARTESIAN_POINT('Ctrl Pts',(208.369989533667,94.7397376084047,341.826490424806));
#26092=CARTESIAN_POINT('Ctrl Pts',(206.616317913094,94.6772376084047,343.30733094404));
#26093=CARTESIAN_POINT('Ctrl Pts',(204.86264629252,94.6147376084047,344.788171463274));
#26094=CARTESIAN_POINT('Ctrl Pts',(202.575500824633,94.5522376084047,344.595250741398));
#26095=CARTESIAN_POINT('Ctrl Pts',(200.288355356745,94.4897376084047,344.402330019522));
#26096=CARTESIAN_POINT('Ctrl Pts',(198.807514837511,94.4272376084047,342.648658398949));
#26097=CARTESIAN_POINT('Ctrl Pts',(197.326674318278,94.3647376084047,340.894986778376));
#26098=CARTESIAN_POINT('Ctrl Pts',(197.519595040153,94.3022376084047,338.607841310488));
#26099=CARTESIAN_POINT('Ctrl Pts',(197.712515762029,94.2397376084047,336.320695842601));
#26100=CARTESIAN_POINT('Ctrl Pts',(199.466187382602,94.1772376084047,334.839855323367));
#26101=CARTESIAN_POINT('Ctrl Pts',(201.219859003176,94.1147376084047,333.359014804133));
#26102=CARTESIAN_POINT('Ctrl Pts',(203.507004471063,94.0522376084047,333.551935526009));
#26103=CARTESIAN_POINT('Ctrl Pts',(205.794149938951,93.9897376084047,333.744856247885));
#26104=CARTESIAN_POINT('Ctrl Pts',(207.274990458185,93.9272376084047,335.498527868458));
#26105=CARTESIAN_POINT('Ctrl Pts',(208.755830977418,93.8647376084047,337.252199489031));
#26106=CARTESIAN_POINT('Ctrl Pts',(208.562910255543,93.8022376084047,339.539344956919));
#26107=CARTESIAN_POINT('Origin',(203.041252647848,99.3647376084047,339.073593133703));
#26108=CARTESIAN_POINT('',(208.562910255543,92.8022376084047,339.539344956919));
#26109=CARTESIAN_POINT('',(208.562910255543,92.9272376084047,339.539344956919));
#26110=CARTESIAN_POINT('',(208.562910255543,99.3647376084047,339.539344956919));
#26111=CARTESIAN_POINT('Ctrl Pts',(208.562910255543,93.9272376084047,339.539344956919));
#26112=CARTESIAN_POINT('Ctrl Pts',(208.369989533667,93.8647376084047,341.826490424806));
#26113=CARTESIAN_POINT('Ctrl Pts',(206.616317913094,93.8022376084047,343.30733094404));
#26114=CARTESIAN_POINT('Ctrl Pts',(204.86264629252,93.7397376084047,344.788171463274));
#26115=CARTESIAN_POINT('Ctrl Pts',(202.575500824633,93.6772376084047,344.595250741398));
#26116=CARTESIAN_POINT('Ctrl Pts',(200.288355356745,93.6147376084047,344.402330019522));
#26117=CARTESIAN_POINT('Ctrl Pts',(198.807514837511,93.5522376084047,342.648658398949));
#26118=CARTESIAN_POINT('Ctrl Pts',(197.326674318278,93.4897376084047,340.894986778376));
#26119=CARTESIAN_POINT('Ctrl Pts',(197.519595040153,93.4272376084047,338.607841310488));
#26120=CARTESIAN_POINT('Ctrl Pts',(197.712515762029,93.3647376084047,336.320695842601));
#26121=CARTESIAN_POINT('Ctrl Pts',(199.466187382602,93.3022376084047,334.839855323367));
#26122=CARTESIAN_POINT('Ctrl Pts',(201.219859003176,93.2397376084047,333.359014804133));
#26123=CARTESIAN_POINT('Ctrl Pts',(203.507004471063,93.1772376084047,333.551935526009));
#26124=CARTESIAN_POINT('Ctrl Pts',(205.794149938951,93.1147376084047,333.744856247885));
#26125=CARTESIAN_POINT('Ctrl Pts',(207.274990458185,93.0522376084047,335.498527868458));
#26126=CARTESIAN_POINT('Ctrl Pts',(208.755830977418,92.9897376084047,337.252199489031));
#26127=CARTESIAN_POINT('Ctrl Pts',(208.562910255543,92.9272376084047,339.539344956919));
#26128=CARTESIAN_POINT('Ctrl Pts',(208.562910255543,93.8022376084047,339.539344956919));
#26129=CARTESIAN_POINT('Ctrl Pts',(208.369989533667,93.7397376084047,341.826490424806));
#26130=CARTESIAN_POINT('Ctrl Pts',(206.616317913094,93.6772376084047,343.30733094404));
#26131=CARTESIAN_POINT('Ctrl Pts',(204.86264629252,93.6147376084047,344.788171463274));
#26132=CARTESIAN_POINT('Ctrl Pts',(202.575500824633,93.5522376084047,344.595250741398));
#26133=CARTESIAN_POINT('Ctrl Pts',(200.288355356745,93.4897376084047,344.402330019522));
#26134=CARTESIAN_POINT('Ctrl Pts',(198.807514837511,93.4272376084047,342.648658398949));
#26135=CARTESIAN_POINT('Ctrl Pts',(197.326674318278,93.3647376084047,340.894986778376));
#26136=CARTESIAN_POINT('Ctrl Pts',(197.519595040153,93.3022376084047,338.607841310488));
#26137=CARTESIAN_POINT('Ctrl Pts',(197.712515762029,93.2397376084047,336.320695842601));
#26138=CARTESIAN_POINT('Ctrl Pts',(199.466187382602,93.1772376084047,334.839855323367));
#26139=CARTESIAN_POINT('Ctrl Pts',(201.219859003176,93.1147376084047,333.359014804133));
#26140=CARTESIAN_POINT('Ctrl Pts',(203.507004471063,93.0522376084047,333.551935526009));
#26141=CARTESIAN_POINT('Ctrl Pts',(205.794149938951,92.9897376084047,333.744856247885));
#26142=CARTESIAN_POINT('Ctrl Pts',(207.274990458185,92.9272376084047,335.498527868458));
#26143=CARTESIAN_POINT('Ctrl Pts',(208.755830977418,92.8647376084047,337.252199489031));
#26144=CARTESIAN_POINT('Ctrl Pts',(208.562910255543,92.8022376084047,339.539344956919));
#26145=CARTESIAN_POINT('Origin',(203.041252647848,99.3647376084047,339.073593133703));
#26146=CARTESIAN_POINT('',(208.562910255543,91.8022376084047,339.539344956919));
#26147=CARTESIAN_POINT('',(208.562910255543,91.9272376084047,339.539344956919));
#26148=CARTESIAN_POINT('',(208.562910255543,99.3647376084047,339.539344956919));
#26149=CARTESIAN_POINT('Ctrl Pts',(208.562910255543,92.9272376084047,339.539344956919));
#26150=CARTESIAN_POINT('Ctrl Pts',(208.369989533667,92.8647376084047,341.826490424806));
#26151=CARTESIAN_POINT('Ctrl Pts',(206.616317913094,92.8022376084047,343.30733094404));
#26152=CARTESIAN_POINT('Ctrl Pts',(204.86264629252,92.7397376084047,344.788171463274));
#26153=CARTESIAN_POINT('Ctrl Pts',(202.575500824633,92.6772376084047,344.595250741398));
#26154=CARTESIAN_POINT('Ctrl Pts',(200.288355356745,92.6147376084047,344.402330019522));
#26155=CARTESIAN_POINT('Ctrl Pts',(198.807514837511,92.5522376084047,342.648658398949));
#26156=CARTESIAN_POINT('Ctrl Pts',(197.326674318278,92.4897376084047,340.894986778376));
#26157=CARTESIAN_POINT('Ctrl Pts',(197.519595040153,92.4272376084047,338.607841310488));
#26158=CARTESIAN_POINT('Ctrl Pts',(197.712515762029,92.3647376084047,336.320695842601));
#26159=CARTESIAN_POINT('Ctrl Pts',(199.466187382602,92.3022376084047,334.839855323367));
#26160=CARTESIAN_POINT('Ctrl Pts',(201.219859003176,92.2397376084047,333.359014804133));
#26161=CARTESIAN_POINT('Ctrl Pts',(203.507004471063,92.1772376084047,333.551935526009));
#26162=CARTESIAN_POINT('Ctrl Pts',(205.794149938951,92.1147376084047,333.744856247885));
#26163=CARTESIAN_POINT('Ctrl Pts',(207.274990458185,92.0522376084047,335.498527868458));
#26164=CARTESIAN_POINT('Ctrl Pts',(208.755830977418,91.9897376084047,337.252199489031));
#26165=CARTESIAN_POINT('Ctrl Pts',(208.562910255543,91.9272376084047,339.539344956919));
#26166=CARTESIAN_POINT('Ctrl Pts',(208.562910255543,92.8022376084047,339.539344956919));
#26167=CARTESIAN_POINT('Ctrl Pts',(208.369989533667,92.7397376084047,341.826490424806));
#26168=CARTESIAN_POINT('Ctrl Pts',(206.616317913094,92.6772376084047,343.30733094404));
#26169=CARTESIAN_POINT('Ctrl Pts',(204.86264629252,92.6147376084047,344.788171463274));
#26170=CARTESIAN_POINT('Ctrl Pts',(202.575500824633,92.5522376084047,344.595250741398));
#26171=CARTESIAN_POINT('Ctrl Pts',(200.288355356745,92.4897376084047,344.402330019522));
#26172=CARTESIAN_POINT('Ctrl Pts',(198.807514837511,92.4272376084047,342.648658398949));
#26173=CARTESIAN_POINT('Ctrl Pts',(197.326674318278,92.3647376084047,340.894986778376));
#26174=CARTESIAN_POINT('Ctrl Pts',(197.519595040153,92.3022376084047,338.607841310488));
#26175=CARTESIAN_POINT('Ctrl Pts',(197.712515762029,92.2397376084047,336.320695842601));
#26176=CARTESIAN_POINT('Ctrl Pts',(199.466187382602,92.1772376084047,334.839855323367));
#26177=CARTESIAN_POINT('Ctrl Pts',(201.219859003176,92.1147376084047,333.359014804133));
#26178=CARTESIAN_POINT('Ctrl Pts',(203.507004471063,92.0522376084047,333.551935526009));
#26179=CARTESIAN_POINT('Ctrl Pts',(205.794149938951,91.9897376084047,333.744856247885));
#26180=CARTESIAN_POINT('Ctrl Pts',(207.274990458185,91.9272376084047,335.498527868458));
#26181=CARTESIAN_POINT('Ctrl Pts',(208.755830977418,91.8647376084047,337.252199489031));
#26182=CARTESIAN_POINT('Ctrl Pts',(208.562910255543,91.8022376084047,339.539344956919));
#26183=CARTESIAN_POINT('Origin',(203.041252647848,99.3647376084047,339.073593133703));
#26184=CARTESIAN_POINT('',(208.562910255543,90.8022376084047,339.539344956919));
#26185=CARTESIAN_POINT('',(208.562910255543,90.9272376084047,339.539344956919));
#26186=CARTESIAN_POINT('',(208.562910255543,99.3647376084047,339.539344956919));
#26187=CARTESIAN_POINT('Ctrl Pts',(208.562910255543,91.9272376084047,339.539344956919));
#26188=CARTESIAN_POINT('Ctrl Pts',(208.369989533667,91.8647376084047,341.826490424806));
#26189=CARTESIAN_POINT('Ctrl Pts',(206.616317913094,91.8022376084047,343.30733094404));
#26190=CARTESIAN_POINT('Ctrl Pts',(204.86264629252,91.7397376084047,344.788171463274));
#26191=CARTESIAN_POINT('Ctrl Pts',(202.575500824633,91.6772376084047,344.595250741398));
#26192=CARTESIAN_POINT('Ctrl Pts',(200.288355356745,91.6147376084047,344.402330019522));
#26193=CARTESIAN_POINT('Ctrl Pts',(198.807514837511,91.5522376084047,342.648658398949));
#26194=CARTESIAN_POINT('Ctrl Pts',(197.326674318278,91.4897376084047,340.894986778376));
#26195=CARTESIAN_POINT('Ctrl Pts',(197.519595040153,91.4272376084047,338.607841310488));
#26196=CARTESIAN_POINT('Ctrl Pts',(197.712515762029,91.3647376084047,336.320695842601));
#26197=CARTESIAN_POINT('Ctrl Pts',(199.466187382602,91.3022376084047,334.839855323367));
#26198=CARTESIAN_POINT('Ctrl Pts',(201.219859003176,91.2397376084047,333.359014804133));
#26199=CARTESIAN_POINT('Ctrl Pts',(203.507004471063,91.1772376084047,333.551935526009));
#26200=CARTESIAN_POINT('Ctrl Pts',(205.794149938951,91.1147376084047,333.744856247885));
#26201=CARTESIAN_POINT('Ctrl Pts',(207.274990458185,91.0522376084047,335.498527868458));
#26202=CARTESIAN_POINT('Ctrl Pts',(208.755830977418,90.9897376084047,337.252199489031));
#26203=CARTESIAN_POINT('Ctrl Pts',(208.562910255543,90.9272376084047,339.539344956919));
#26204=CARTESIAN_POINT('Ctrl Pts',(208.562910255543,91.8022376084047,339.539344956919));
#26205=CARTESIAN_POINT('Ctrl Pts',(208.369989533667,91.7397376084047,341.826490424806));
#26206=CARTESIAN_POINT('Ctrl Pts',(206.616317913094,91.6772376084047,343.30733094404));
#26207=CARTESIAN_POINT('Ctrl Pts',(204.86264629252,91.6147376084047,344.788171463274));
#26208=CARTESIAN_POINT('Ctrl Pts',(202.575500824633,91.5522376084047,344.595250741398));
#26209=CARTESIAN_POINT('Ctrl Pts',(200.288355356745,91.4897376084047,344.402330019522));
#26210=CARTESIAN_POINT('Ctrl Pts',(198.807514837511,91.4272376084047,342.648658398949));
#26211=CARTESIAN_POINT('Ctrl Pts',(197.326674318278,91.3647376084047,340.894986778376));
#26212=CARTESIAN_POINT('Ctrl Pts',(197.519595040153,91.3022376084047,338.607841310488));
#26213=CARTESIAN_POINT('Ctrl Pts',(197.712515762029,91.2397376084047,336.320695842601));
#26214=CARTESIAN_POINT('Ctrl Pts',(199.466187382602,91.1772376084047,334.839855323367));
#26215=CARTESIAN_POINT('Ctrl Pts',(201.219859003176,91.1147376084047,333.359014804133));
#26216=CARTESIAN_POINT('Ctrl Pts',(203.507004471063,91.0522376084047,333.551935526009));
#26217=CARTESIAN_POINT('Ctrl Pts',(205.794149938951,90.9897376084047,333.744856247885));
#26218=CARTESIAN_POINT('Ctrl Pts',(207.274990458185,90.9272376084047,335.498527868458));
#26219=CARTESIAN_POINT('Ctrl Pts',(208.755830977418,90.8647376084047,337.252199489031));
#26220=CARTESIAN_POINT('Ctrl Pts',(208.562910255543,90.8022376084047,339.539344956919));
#26221=CARTESIAN_POINT('Origin',(203.041252647848,99.3647376084047,339.073593133703));
#26222=CARTESIAN_POINT('',(208.562910255543,89.8022376084047,339.539344956919));
#26223=CARTESIAN_POINT('',(208.562910255543,89.9272376084047,339.539344956919));
#26224=CARTESIAN_POINT('',(208.562910255543,99.3647376084047,339.539344956919));
#26225=CARTESIAN_POINT('',(197.519595040153,89.3022376084047,338.607841310488));
#26226=CARTESIAN_POINT('Ctrl Pts',(208.562910255543,89.8022376084047,339.539344956919));
#26227=CARTESIAN_POINT('Ctrl Pts',(208.369989533667,89.7397376084047,341.826490424806));
#26228=CARTESIAN_POINT('Ctrl Pts',(206.616317913094,89.6772376084047,343.30733094404));
#26229=CARTESIAN_POINT('Ctrl Pts',(204.86264629252,89.6147376084047,344.788171463274));
#26230=CARTESIAN_POINT('Ctrl Pts',(202.575500824633,89.5522376084047,344.595250741398));
#26231=CARTESIAN_POINT('Ctrl Pts',(200.288355356745,89.4897376084047,344.402330019522));
#26232=CARTESIAN_POINT('Ctrl Pts',(198.807514837511,89.4272376084047,342.648658398949));
#26233=CARTESIAN_POINT('Ctrl Pts',(197.326674318278,89.3647376084047,340.894986778376));
#26234=CARTESIAN_POINT('Ctrl Pts',(197.519595040153,89.3022376084047,338.607841310488));
#26235=CARTESIAN_POINT('',(197.519595040153,89.4272376084047,338.607841310488));
#26236=CARTESIAN_POINT('',(197.519595040153,89.3647376084047,338.607841310488));
#26237=CARTESIAN_POINT('Ctrl Pts',(208.562910255543,89.9272376084047,339.539344956919));
#26238=CARTESIAN_POINT('Ctrl Pts',(208.369989533667,89.8647376084047,341.826490424806));
#26239=CARTESIAN_POINT('Ctrl Pts',(206.616317913094,89.8022376084047,343.30733094404));
#26240=CARTESIAN_POINT('Ctrl Pts',(204.86264629252,89.7397376084047,344.788171463274));
#26241=CARTESIAN_POINT('Ctrl Pts',(202.575500824633,89.6772376084047,344.595250741398));
#26242=CARTESIAN_POINT('Ctrl Pts',(200.288355356745,89.6147376084047,344.402330019522));
#26243=CARTESIAN_POINT('Ctrl Pts',(198.807514837511,89.5522376084047,342.648658398949));
#26244=CARTESIAN_POINT('Ctrl Pts',(197.326674318278,89.4897376084046,340.894986778376));
#26245=CARTESIAN_POINT('Ctrl Pts',(197.519595040153,89.4272376084047,338.607841310488));
#26246=CARTESIAN_POINT('Origin',(203.041252647848,90.7397376070391,339.073593133703));
#26247=CARTESIAN_POINT('',(208.023559698486,90.4897376097703,339.49385073704));
#26248=CARTESIAN_POINT('',(208.023559697325,90.2397376062055,339.493850750802));
#26249=CARTESIAN_POINT('',(208.023559698486,90.7397376070391,339.49385073704));
#26250=CARTESIAN_POINT('',(198.05894559721,89.7397376070391,338.653335530367));
#26251=CARTESIAN_POINT('Ctrl Pts',(208.023559697324,90.2397376066219,339.493850750814));
#26252=CARTESIAN_POINT('Ctrl Pts',(207.967987441932,90.2197850692749,340.152680070072));
#26253=CARTESIAN_POINT('Ctrl Pts',(207.782272105817,90.1983863675473,340.794108678668));
#26254=CARTESIAN_POINT('Ctrl Pts',(207.180297127688,90.155775815837,341.951424930312));
#26255=CARTESIAN_POINT('Ctrl Pts',(206.776201966202,90.1349754025954,342.459419328652));
#26256=CARTESIAN_POINT('Ctrl Pts',(205.779186547245,90.0953363464056,343.310258462585));
#26257=CARTESIAN_POINT('Ctrl Pts',(205.189690768065,90.07382879957,343.637577962599));
#26258=CARTESIAN_POINT('Ctrl Pts',(203.940216513502,90.0310110797161,344.033994790525));
#26259=CARTESIAN_POINT('Ctrl Pts',(203.295286092653,90.0102018454483,344.108396766252));
#26260=CARTESIAN_POINT('Ctrl Pts',(201.988697801305,89.970545740923,344.006885610872));
#26261=CARTESIAN_POINT('Ctrl Pts',(201.340411387471,89.9490761928212,343.822541545439));
#26262=CARTESIAN_POINT('Ctrl Pts',(200.175806375358,89.9062643752447,343.221250634602));
#26263=CARTESIAN_POINT('Ctrl Pts',(199.666462394256,89.8854456907724,342.818549125729));
#26264=CARTESIAN_POINT('Ctrl Pts',(198.812968631957,89.8457712813281,341.824314123643));
#26265=CARTESIAN_POINT('Ctrl Pts',(198.484119335941,89.8243423309613,341.236348328231));
#26266=CARTESIAN_POINT('Ctrl Pts',(198.0787326342,89.7810008888298,339.972904723502));
#26267=CARTESIAN_POINT('Ctrl Pts',(198.003482338787,89.7596510109899,339.310872672583));
#26268=CARTESIAN_POINT('Ctrl Pts',(198.05894559721,89.7397376070391,338.653335530367));
#26269=CARTESIAN_POINT('',(198.05894559721,88.9897376097703,338.653335530367));
#26270=CARTESIAN_POINT('',(198.05894559721,89.3647376084047,338.653335530367));
#26271=CARTESIAN_POINT('',(208.023559701634,89.4897376120309,339.493850699717));
#26272=CARTESIAN_POINT('Ctrl Pts',(198.05894559721,88.9897376097702,338.653335530367));
#26273=CARTESIAN_POINT('Ctrl Pts',(198.005090318586,89.0090736882593,339.29180948604));
#26274=CARTESIAN_POINT('Ctrl Pts',(198.074464345089,89.0297695070508,339.934698175558));
#26275=CARTESIAN_POINT('Ctrl Pts',(198.460228811946,89.0725294411995,341.185710855226));
#26276=CARTESIAN_POINT('Ctrl Pts',(198.783316518751,89.0941847312611,341.778563826942));
#26277=CARTESIAN_POINT('Ctrl Pts',(199.626819057716,89.1337898500415,342.782311924146));
#26278=CARTESIAN_POINT('Ctrl Pts',(200.131272251541,89.154503989331,343.190034651175));
#26279=CARTESIAN_POINT('Ctrl Pts',(201.289603850442,89.1973264338864,343.804177733881));
#26280=CARTESIAN_POINT('Ctrl Pts',(201.936946584312,89.2189840397084,343.995714396649));
#26281=CARTESIAN_POINT('Ctrl Pts',(203.242840017277,89.2586049282707,344.110677077451));
#26282=CARTESIAN_POINT('Ctrl Pts',(203.88785366535,89.2792909113593,344.043124405737));
#26283=CARTESIAN_POINT('Ctrl Pts',(205.141524234994,89.3221070406722,343.66003376277));
#26284=CARTESIAN_POINT('Ctrl Pts',(205.735050890444,89.3437671108541,343.338577820788));
#26285=CARTESIAN_POINT('Ctrl Pts',(206.74077207075,89.3834050008466,342.497961995612));
#26286=CARTESIAN_POINT('Ctrl Pts',(207.14975080574,89.4040608004847,341.994741599264));
#26287=CARTESIAN_POINT('Ctrl Pts',(207.766908544629,89.4468700687691,340.838421449675));
#26288=CARTESIAN_POINT('Ctrl Pts',(207.960204977618,89.4685327560788,340.19181273531));
#26289=CARTESIAN_POINT('Ctrl Pts',(208.021696674723,89.4890809562878,339.515515705685));
#26290=CARTESIAN_POINT('Ctrl Pts',(208.022645922154,89.4894095295346,339.504683889451));
#26291=CARTESIAN_POINT('Ctrl Pts',(208.023559701637,89.4897376109016,339.493850699683));
#26292=CARTESIAN_POINT('',(208.023559698486,88.7397376070391,339.49385073704));
#26293=CARTESIAN_POINT('',(208.023559698486,90.7397376070391,339.49385073704));
#26294=CARTESIAN_POINT('Origin',(203.041252647848,88.7397376070391,339.073593133703));
#26295=CARTESIAN_POINT('Ctrl Pts',(208.023559701637,89.4897376109016,339.493850699683));
#26296=CARTESIAN_POINT('Ctrl Pts',(208.076621398869,89.5087887654594,338.864784884326));
#26297=CARTESIAN_POINT('Ctrl Pts',(208.01007822827,89.5291676759465,338.23117685209));
#26298=CARTESIAN_POINT('Ctrl Pts',(207.633971862084,89.5716142611113,336.987154430157));
#26299=CARTESIAN_POINT('Ctrl Pts',(207.31442046961,89.5932797215223,336.392847542905));
#26300=CARTESIAN_POINT('Ctrl Pts',(206.477172736627,89.6329556427219,335.384830836249));
#26301=CARTESIAN_POINT('Ctrl Pts',(205.975388234505,89.6535445750485,334.974388851488));
#26302=CARTESIAN_POINT('Ctrl Pts',(204.821415324561,89.6963382969244,334.353724563616));
#26303=CARTESIAN_POINT('Ctrl Pts',(204.175667351599,89.7180066883986,334.158381533697));
#26304=CARTESIAN_POINT('Ctrl Pts',(202.871295313364,89.7577038137528,334.03538883353));
#26305=CARTESIAN_POINT('Ctrl Pts',(202.226242850506,89.7782558592171,334.098831131073));
#26306=CARTESIAN_POINT('Ctrl Pts',(200.970929427903,89.8210407931791,334.473622444604));
#26307=CARTESIAN_POINT('Ctrl Pts',(200.375722267236,89.8427122741615,334.790956207083));
#26308=CARTESIAN_POINT('Ctrl Pts',(199.365042657244,89.8824321833746,335.624283739083));
#26309=CARTESIAN_POINT('Ctrl Pts',(198.952900510298,89.9029449122807,336.124400305907));
#26310=CARTESIAN_POINT('Ctrl Pts',(198.328169474475,89.9457203070914,337.275640752034));
#26311=CARTESIAN_POINT('Ctrl Pts',(198.130453351107,89.9673950346759,337.920381087117));
#26312=CARTESIAN_POINT('Ctrl Pts',(198.002447617131,90.0071394005659,339.223791172444));
#26313=CARTESIAN_POINT('Ctrl Pts',(198.063325820062,90.0276102965623,339.868868364745));
#26314=CARTESIAN_POINT('Ctrl Pts',(198.432941636231,90.0703753398379,341.125192231522));
#26315=CARTESIAN_POINT('Ctrl Pts',(198.747700402311,90.0920534675672,341.721433688454));
#26316=CARTESIAN_POINT('Ctrl Pts',(199.576477995088,90.1318240574313,342.735191965214));
#26317=CARTESIAN_POINT('Ctrl Pts',(200.074663144713,90.1522505277069,343.149303477133));
#26318=CARTESIAN_POINT('Ctrl Pts',(201.222731634814,90.1950043416697,343.778734947524));
#26319=CARTESIAN_POINT('Ctrl Pts',(201.866294730716,90.2166860169306,343.979193250902));
#26320=CARTESIAN_POINT('Ctrl Pts',(203.168580269176,90.2564846931557,344.112998312768));
#26321=CARTESIAN_POINT('Ctrl Pts',(203.813686573369,90.2768640815098,344.055084606509));
#26322=CARTESIAN_POINT('Ctrl Pts',(205.071164927256,90.319605718618,343.691450627512));
#26323=CARTESIAN_POINT('Ctrl Pts',(205.668588705134,90.3412910795915,343.379672154712));
#26324=CARTESIAN_POINT('Ctrl Pts',(206.685892465735,90.3811197993696,342.556158140771));
#26325=CARTESIAN_POINT('Ctrl Pts',(207.102277090973,90.4014494024921,342.060201444154));
#26326=CARTESIAN_POINT('Ctrl Pts',(207.73712014721,90.444177840985,340.91580305819));
#26327=CARTESIAN_POINT('Ctrl Pts',(207.940734477137,90.465867013117,340.273612075629));
#26328=CARTESIAN_POINT('Ctrl Pts',(208.016544922203,90.4873766903905,339.571581044975));
#26329=CARTESIAN_POINT('Ctrl Pts',(208.020280595153,90.4885602878616,339.532725702126));
#26330=CARTESIAN_POINT('Ctrl Pts',(208.023559698486,90.4897376097703,339.49385073704));
#26331=CARTESIAN_POINT('Origin',(203.041252647848,90.7397376070391,339.073593133703));
#26332=CARTESIAN_POINT('',(208.023559698486,91.4897376097703,339.49385073704));
#26333=CARTESIAN_POINT('',(208.023559700815,91.2397376087116,339.493850709426));
#26334=CARTESIAN_POINT('',(208.023559698486,90.7397376070391,339.49385073704));
#26335=CARTESIAN_POINT('Ctrl Pts',(208.023559700817,91.2397376078761,339.493850709401));
#26336=CARTESIAN_POINT('Ctrl Pts',(208.022777603548,91.2394568054081,339.503122758184));
#26337=CARTESIAN_POINT('Ctrl Pts',(208.021969523626,91.2391756424233,339.512393806923));
#26338=CARTESIAN_POINT('Ctrl Pts',(207.961248460585,91.2186807736327,340.187251224621));
#26339=CARTESIAN_POINT('Ctrl Pts',(207.768528810363,91.1970197338633,340.834101140624));
#26340=CARTESIAN_POINT('Ctrl Pts',(207.152359200336,91.1542061274548,341.991081257056));
#26341=CARTESIAN_POINT('Ctrl Pts',(206.743792353717,91.1335312920547,342.494705903154));
#26342=CARTESIAN_POINT('Ctrl Pts',(205.738717945261,91.0939041360525,343.336268826221));
#26343=CARTESIAN_POINT('Ctrl Pts',(205.145411812608,91.0722456178563,343.658260191733));
#26344=CARTESIAN_POINT('Ctrl Pts',(203.891956933637,91.0294254953918,344.042430123254));
#26345=CARTESIAN_POINT('Ctrl Pts',(203.246948260431,91.0087217510958,344.110517218662));
#26346=CARTESIAN_POINT('Ctrl Pts',(201.94085888431,90.9691108202269,343.996598011257));
#26347=CARTESIAN_POINT('Ctrl Pts',(201.293310661819,90.9474546733328,343.805556421513));
#26348=CARTESIAN_POINT('Ctrl Pts',(200.13441431828,90.9046285537418,343.192261376409));
#26349=CARTESIAN_POINT('Ctrl Pts',(199.629614609139,90.883897862016,342.784891644092));
#26350=CARTESIAN_POINT('Ctrl Pts',(198.785301502277,90.8443019743155,341.781698511198));
#26351=CARTESIAN_POINT('Ctrl Pts',(198.461755707079,90.8226480531073,341.189035529012));
#26352=CARTESIAN_POINT('Ctrl Pts',(198.074450686669,90.7798164147686,339.93620986008));
#26353=CARTESIAN_POINT('Ctrl Pts',(198.004811342931,90.7590606317338,339.291215546541));
#26354=CARTESIAN_POINT('Ctrl Pts',(198.115700527921,90.7194786821743,337.984559478539));
#26355=CARTESIAN_POINT('Ctrl Pts',(198.305303958764,90.6978268463121,337.336416836373));
#26356=CARTESIAN_POINT('Ctrl Pts',(198.9161012012,90.6549925470052,336.175948231855));
#26357=CARTESIAN_POINT('Ctrl Pts',(199.322422686908,90.6342218043809,335.670126393806));
#26358=CARTESIAN_POINT('Ctrl Pts',(200.323893310057,90.5946398319776,334.823555912036));
#26359=CARTESIAN_POINT('Ctrl Pts',(200.915848087721,90.573003751093,334.498699366079));
#26360=CARTESIAN_POINT('Ctrl Pts',(202.167969031834,90.5301668015468,334.108647846274));
#26361=CARTESIAN_POINT('Ctrl Pts',(202.812944576869,90.5093894178012,334.03759841499));
#26362=CARTESIAN_POINT('Ctrl Pts',(204.119678768791,90.4697947026187,334.145756215511));
#26363=CARTESIAN_POINT('Ctrl Pts',(204.767963222047,90.4481874864064,334.333847661661));
#26364=CARTESIAN_POINT('Ctrl Pts',(205.929741942553,90.4053547586586,334.942004109873));
#26365=CARTESIAN_POINT('Ctrl Pts',(206.436569810911,90.3845702374061,335.347297289931));
#26366=CARTESIAN_POINT('Ctrl Pts',(207.285116225065,90.3449618052323,336.346708031024));
#26367=CARTESIAN_POINT('Ctrl Pts',(207.611113328099,90.3233855504265,336.937524743176));
#26368=CARTESIAN_POINT('Ctrl Pts',(208.004111908485,90.2805574126289,338.188423237859));
#26369=CARTESIAN_POINT('Ctrl Pts',(208.076712527105,90.2597652258056,338.833380030691));
#26370=CARTESIAN_POINT('Ctrl Pts',(208.024640833897,90.2401304777962,339.480882387206));
#26371=CARTESIAN_POINT('Ctrl Pts',(208.024106567416,90.2399339536268,339.487367406785));
#26372=CARTESIAN_POINT('Ctrl Pts',(208.023559697324,90.2397376066219,339.493850750815));
#26373=CARTESIAN_POINT('Ctrl Pts',(208.023559698486,90.4897376097703,339.49385073704));
#26374=CARTESIAN_POINT('Ctrl Pts',(208.074141955547,90.5078985499357,338.894179644854));
#26375=CARTESIAN_POINT('Ctrl Pts',(208.016074048837,90.5272800245765,338.289920020022));
#26376=CARTESIAN_POINT('Ctrl Pts',(207.669976465734,90.5687190538142,337.068707858769));
#26377=CARTESIAN_POINT('Ctrl Pts',(207.36163447278,90.5904121457754,336.469940367169));
#26378=CARTESIAN_POINT('Ctrl Pts',(206.544186638362,90.6303071955841,335.448571824803));
#26379=CARTESIAN_POINT('Ctrl Pts',(206.050790454263,90.6505290328337,335.029574160708));
#26380=CARTESIAN_POINT('Ctrl Pts',(204.910622499034,90.6932276895281,334.388528811024));
#26381=CARTESIAN_POINT('Ctrl Pts',(204.270026250128,90.7149247886381,334.181298843545));
#26382=CARTESIAN_POINT('Ctrl Pts',(202.970578181399,90.7548563028777,334.033140891833));
#26383=CARTESIAN_POINT('Ctrl Pts',(202.325397358095,90.7750201800593,334.083725263663));
#26384=CARTESIAN_POINT('Ctrl Pts',(201.065127762074,90.817702082896,334.432579756435));
#26385=CARTESIAN_POINT('Ctrl Pts',(200.464843293427,90.8394032499985,334.736976355467));
#26386=CARTESIAN_POINT('Ctrl Pts',(199.438838548709,90.8793735388622,335.54746334369));
#26387=CARTESIAN_POINT('Ctrl Pts',(199.016851052484,90.8994768022906,336.037931421971));
#26388=CARTESIAN_POINT('Ctrl Pts',(198.368733749474,90.9421405884771,337.173244318086));
#26389=CARTESIAN_POINT('Ctrl Pts',(198.157383424673,90.9638458522645,337.811993279119));
#26390=CARTESIAN_POINT('Ctrl Pts',(198.000468924039,91.0038573003804,339.109672014915));
#26391=CARTESIAN_POINT('Ctrl Pts',(198.046586531689,91.0238973893563,339.754900134417));
#26392=CARTESIAN_POINT('Ctrl Pts',(198.386441780438,91.0665416006326,341.016826928627));
#26393=CARTESIAN_POINT('Ctrl Pts',(198.686331159239,91.0882509514357,341.618810932091));
#26394=CARTESIAN_POINT('Ctrl Pts',(199.488870313868,91.1283060088851,342.650072663083));
#26395=CARTESIAN_POINT('Ctrl Pts',(199.976007972567,91.1482804968743,343.075463033303));
#26396=CARTESIAN_POINT('Ctrl Pts',(201.10577680151,91.1909035761506,343.731596696223));
#26397=CARTESIAN_POINT('Ctrl Pts',(201.74239434411,91.2126169592302,343.947614337832));
#26398=CARTESIAN_POINT('Ctrl Pts',(203.038028984831,91.2527181305916,344.114470201953));
#26399=CARTESIAN_POINT('Ctrl Pts',(203.683312579226,91.2726247708513,344.073419879154));
#26400=CARTESIAN_POINT('Ctrl Pts',(204.947079311213,91.3152250594544,343.743765396875));
#26401=CARTESIAN_POINT('Ctrl Pts',(205.550950855541,91.3369423678553,343.448995896975));
#26402=CARTESIAN_POINT('Ctrl Pts',(206.588133917363,91.3770921991743,342.655480271349));
#26403=CARTESIAN_POINT('Ctrl Pts',(207.01737412275,91.3969289745741,342.17210754058));
#26404=CARTESIAN_POINT('Ctrl Pts',(207.682534559373,91.4395047102744,341.048633463138));
#26405=CARTESIAN_POINT('Ctrl Pts',(207.90380306619,91.4612257773324,340.414463808285));
#26406=CARTESIAN_POINT('Ctrl Pts',(208.006509858919,91.4844128467684,339.668527023477));
#26407=CARTESIAN_POINT('Ctrl Pts',(208.016187834062,91.4870908320957,339.581246876471));
#26408=CARTESIAN_POINT('Ctrl Pts',(208.023559698486,91.4897376097703,339.49385073704));
#26409=CARTESIAN_POINT('Origin',(203.041252647848,90.7397376070391,339.073593133703));
#26410=CARTESIAN_POINT('',(208.023559698486,92.4897376097702,339.49385073704));
#26411=CARTESIAN_POINT('',(208.023559698486,92.2397376070391,339.49385073704));
#26412=CARTESIAN_POINT('',(208.023559698486,90.7397376070391,339.49385073704));
#26413=CARTESIAN_POINT('Ctrl Pts',(208.023559698486,92.2397376070391,339.49385073704));
#26414=CARTESIAN_POINT('Ctrl Pts',(208.020517464755,92.2386453302613,339.529917526663));
#26415=CARTESIAN_POINT('Ctrl Pts',(208.01708222642,92.2375476467766,339.565967592953));
#26416=CARTESIAN_POINT('Ctrl Pts',(207.942746290427,92.2161345415519,340.265432626658));
#26417=CARTESIAN_POINT('Ctrl Pts',(207.740161534077,92.1944477561335,340.908073257731));
#26418=CARTESIAN_POINT('Ctrl Pts',(207.10708409172,92.151710976134,342.053671221179));
#26419=CARTESIAN_POINT('Ctrl Pts',(206.691441794106,92.1313500577135,342.55035555716));
#26420=CARTESIAN_POINT('Ctrl Pts',(205.675294919245,92.0915402777557,343.375589879006));
#26421=CARTESIAN_POINT('Ctrl Pts',(205.078255886551,92.0698572270972,343.688342569117));
#26422=CARTESIAN_POINT('Ctrl Pts',(203.821153157497,92.0271078935813,344.053930965098));
#26423=CARTESIAN_POINT('Ctrl Pts',(203.176056428841,92.0066988775275,344.112813361286));
#26424=CARTESIAN_POINT('Ctrl Pts',(201.873401967365,91.966917911505,343.980903708258));
#26425=CARTESIAN_POINT('Ctrl Pts',(201.229452748241,91.9452384617902,343.781341263561));
#26426=CARTESIAN_POINT('Ctrl Pts',(200.080346273999,91.9024775497843,343.153445553984));
#26427=CARTESIAN_POINT('Ctrl Pts',(199.581529652041,91.8820231121741,342.739977997404));
#26428=CARTESIAN_POINT('Ctrl Pts',(198.751263233901,91.8422690618329,341.727225699921));
#26429=CARTESIAN_POINT('Ctrl Pts',(198.435661751528,91.820593068766,341.131321431086));
#26430=CARTESIAN_POINT('Ctrl Pts',(198.064352892343,91.7778214818585,339.87532692316));
#26431=CARTESIAN_POINT('Ctrl Pts',(198.002635828441,91.7573242411282,339.230257866364));
#26432=CARTESIAN_POINT('Ctrl Pts',(198.129001201107,91.71759530331,337.926531979726));
#26433=CARTESIAN_POINT('Ctrl Pts',(198.325941075757,91.6959226153422,337.281460906651));
#26434=CARTESIAN_POINT('Ctrl Pts',(198.949341762016,91.6531411900911,336.129325382815));
#26435=CARTESIAN_POINT('Ctrl Pts',(199.360927362183,91.6326036927944,335.628662872083));
#26436=CARTESIAN_POINT('Ctrl Pts',(200.370735785543,91.5928981591464,334.794051266812));
#26437=CARTESIAN_POINT('Ctrl Pts',(200.96564898979,91.5712286202447,334.475991011505));
#26438=CARTESIAN_POINT('Ctrl Pts',(202.22067514398,91.5284381304748,334.099738298842));
#26439=CARTESIAN_POINT('Ctrl Pts',(202.865720698403,91.5078628400418,334.035572104211));
#26440=CARTESIAN_POINT('Ctrl Pts',(204.17036252136,91.4681790959201,334.157150043117));
#26441=CARTESIAN_POINT('Ctrl Pts',(204.816393190638,91.4465125479151,334.351822901032));
#26442=CARTESIAN_POINT('Ctrl Pts',(205.971135663743,91.4037137088727,334.971338879327));
#26443=CARTESIAN_POINT('Ctrl Pts',(206.473390617795,91.3831029970338,335.381301410643));
#26444=CARTESIAN_POINT('Ctrl Pts',(207.311742549463,91.3434395197364,336.388566330041));
#26445=CARTESIAN_POINT('Ctrl Pts',(207.631918410012,91.32177580429,336.982618112728));
#26446=CARTESIAN_POINT('Ctrl Pts',(208.009727367198,91.2792733077146,338.227894422968));
#26447=CARTESIAN_POINT('Ctrl Pts',(208.076760034845,91.2588385378259,338.863141318837));
#26448=CARTESIAN_POINT('Ctrl Pts',(208.023559700817,91.2397376078761,339.493850709401));
#26449=CARTESIAN_POINT('Ctrl Pts',(208.023559698486,91.4897376097703,339.49385073704));
#26450=CARTESIAN_POINT('Ctrl Pts',(208.069899534439,91.5063753605728,338.944475093247));
#26451=CARTESIAN_POINT('Ctrl Pts',(208.025106646621,91.524057614868,338.3905838708));
#26452=CARTESIAN_POINT('Ctrl Pts',(207.728366280364,91.5637413335618,337.210042016603));
#26453=CARTESIAN_POINT('Ctrl Pts',(207.439375153272,91.5854659251838,336.604094720386));
#26454=CARTESIAN_POINT('Ctrl Pts',(206.656038908247,91.6257208023941,335.560291864348));
#26455=CARTESIAN_POINT('Ctrl Pts',(206.176893192756,91.6454129861526,335.126725380969));
#26456=CARTESIAN_POINT('Ctrl Pts',(205.060519967291,91.6879339112991,334.451475871497));
#26457=CARTESIAN_POINT('Ctrl Pts',(204.429146484702,91.7096617181724,334.224345307771));
#26458=CARTESIAN_POINT('Ctrl Pts',(203.138553852397,91.7499729797671,334.033716454067));
#26459=CARTESIAN_POINT('Ctrl Pts',(202.493129519806,91.7695911754353,334.062662906401));
#26460=CARTESIAN_POINT('Ctrl Pts',(201.240944432954,91.8115519979504,334.364187588652));
#26461=CARTESIAN_POINT('Ctrl Pts',(200.646587603271,91.832753304877,334.636789266593));
#26462=CARTESIAN_POINT('Ctrl Pts',(199.588991386876,91.8732164414588,335.397844572337));
#26463=CARTESIAN_POINT('Ctrl Pts',(199.137567346313,91.8931225763546,335.881336658372));
#26464=CARTESIAN_POINT('Ctrl Pts',(198.450585441675,91.9355642053956,336.988916328884));
#26465=CARTESIAN_POINT('Ctrl Pts',(198.21927731355,91.9567932396304,337.600944563771));
#26466=CARTESIAN_POINT('Ctrl Pts',(198.002140728478,91.9973185611848,338.885219174848));
#26467=CARTESIAN_POINT('Ctrl Pts',(198.020754761151,92.0171262599735,339.545562830189));
#26468=CARTESIAN_POINT('Ctrl Pts',(198.309989679854,92.0595313129935,340.815939062172));
#26469=CARTESIAN_POINT('Ctrl Pts',(198.575639313402,92.0807885588379,341.4143091349));
#26470=CARTESIAN_POINT('Ctrl Pts',(199.323444141224,92.121378160502,342.48019223246));
#26471=CARTESIAN_POINT('Ctrl Pts',(199.800000993709,92.1410879524949,342.936405838262));
#26472=CARTESIAN_POINT('Ctrl Pts',(200.897816914169,92.1834538593166,343.637236510666));
#26473=CARTESIAN_POINT('Ctrl Pts',(201.507624368599,92.2047396824536,343.876631250823));
#26474=CARTESIAN_POINT('Ctrl Pts',(202.788192744678,92.2453955333451,344.109648388601));
#26475=CARTESIAN_POINT('Ctrl Pts',(203.446952875112,92.265008647927,344.099656435787));
#26476=CARTESIAN_POINT('Ctrl Pts',(204.72027149577,92.3073327523818,343.827813912942));
#26477=CARTESIAN_POINT('Ctrl Pts',(205.322915410455,92.3286473876907,343.569787711577));
#26478=CARTESIAN_POINT('Ctrl Pts',(206.397717593833,92.3693713073093,342.836425211467));
#26479=CARTESIAN_POINT('Ctrl Pts',(206.859090121511,92.3888897174023,342.367358322678));
#26480=CARTESIAN_POINT('Ctrl Pts',(207.574810597222,92.4311692919078,341.280209575513));
#26481=CARTESIAN_POINT('Ctrl Pts',(207.822934129627,92.4525128324795,340.672922664461));
#26482=CARTESIAN_POINT('Ctrl Pts',(207.983048828277,92.4786231563991,339.855911999456));
#26483=CARTESIAN_POINT('Ctrl Pts',(208.008263172363,92.4842455793272,339.675196629055));
#26484=CARTESIAN_POINT('Ctrl Pts',(208.023559698486,92.4897376097703,339.49385073704));
#26485=CARTESIAN_POINT('Origin',(203.041252647848,90.7397376070391,339.073593133703));
#26486=CARTESIAN_POINT('',(208.023559698486,93.4897376097702,339.49385073704));
#26487=CARTESIAN_POINT('',(208.023559698486,93.2397376070391,339.49385073704));
#26488=CARTESIAN_POINT('',(208.023559698486,90.7397376070391,339.49385073704));
#26489=CARTESIAN_POINT('Ctrl Pts',(208.023559698486,93.2397376070391,339.49385073704));
#26490=CARTESIAN_POINT('Ctrl Pts',(208.016584375434,93.2372332026896,339.576545733987));
#26491=CARTESIAN_POINT('Ctrl Pts',(208.007544240813,93.2347008137002,339.659138336034));
#26492=CARTESIAN_POINT('Ctrl Pts',(207.907560317782,93.211676921936,340.400858899981));
#26493=CARTESIAN_POINT('Ctrl Pts',(207.687990813611,93.1899581719302,341.035826439867));
#26494=CARTESIAN_POINT('Ctrl Pts',(207.025752146929,93.1473669371886,342.161344020006));
#26495=CARTESIAN_POINT('Ctrl Pts',(206.597760178299,93.1274864417577,342.645937109802));
#26496=CARTESIAN_POINT('Ctrl Pts',(205.562493897218,93.0873672065052,343.442382086359));
#26497=CARTESIAN_POINT('Ctrl Pts',(204.959230218942,93.0656523263478,343.73881395107));
#26498=CARTESIAN_POINT('Ctrl Pts',(203.696055976313,93.0230376480925,344.071778028136));
#26499=CARTESIAN_POINT('Ctrl Pts',(203.050790602721,93.0030885138555,344.114472922847));
#26500=CARTESIAN_POINT('Ctrl Pts',(201.754488251591,92.9630163493192,343.95084432293));
#26501=CARTESIAN_POINT('Ctrl Pts',(201.117174804287,92.9413054676046,343.736340576226));
#26502=CARTESIAN_POINT('Ctrl Pts',(199.985602468861,92.8986690434082,343.08280780898));
#26503=CARTESIAN_POINT('Ctrl Pts',(199.497382928909,92.8786534365176,342.658523124953));
#26504=CARTESIAN_POINT('Ctrl Pts',(198.692258383647,92.8386258208235,341.628967190428));
#26505=CARTESIAN_POINT('Ctrl Pts',(198.390902569519,92.8169190111372,341.027532231744));
#26506=CARTESIAN_POINT('Ctrl Pts',(198.048121398057,92.7742624361431,339.766140737552));
#26507=CARTESIAN_POINT('Ctrl Pts',(198.000551155381,92.7541827208717,339.120928161138));
#26508=CARTESIAN_POINT('Ctrl Pts',(198.154617219303,92.7141971819735,337.822670682765));
#26509=CARTESIAN_POINT('Ctrl Pts',(198.364628162582,92.6924944701812,337.183317717646));
#26510=CARTESIAN_POINT('Ctrl Pts',(199.010446143125,92.6498192395829,336.04642260089));
#26511=CARTESIAN_POINT('Ctrl Pts',(199.431460314172,92.6296779310761,335.55500148697));
#26512=CARTESIAN_POINT('Ctrl Pts',(200.455957517435,92.5897320584838,334.742246118233));
#26513=CARTESIAN_POINT('Ctrl Pts',(201.055750561644,92.5680334296138,334.436563575521));
#26514=CARTESIAN_POINT('Ctrl Pts',(202.315540845168,92.5253409418072,334.085138141637));
#26515=CARTESIAN_POINT('Ctrl Pts',(202.96070842996,92.5051406632066,334.033278261959));
#26516=CARTESIAN_POINT('Ctrl Pts',(204.260656162087,92.4652321176993,334.178936982935));
#26517=CARTESIAN_POINT('Ctrl Pts',(204.901774474389,92.4435375223459,334.384989397671));
#26518=CARTESIAN_POINT('Ctrl Pts',(206.043323261248,92.4008290825914,335.024014436143));
#26519=CARTESIAN_POINT('Ctrl Pts',(206.537554260903,92.3805725266765,335.442160013568));
#26520=CARTESIAN_POINT('Ctrl Pts',(207.356982019679,92.3406990481215,336.4622043698));
#26521=CARTESIAN_POINT('Ctrl Pts',(207.666445831867,92.3190084083253,337.060535513476));
#26522=CARTESIAN_POINT('Ctrl Pts',(208.015499581875,92.2774682195176,338.284055932193));
#26523=CARTESIAN_POINT('Ctrl Pts',(208.07438933635,92.2579873662533,338.891246855278));
#26524=CARTESIAN_POINT('Ctrl Pts',(208.023559698486,92.239737607039,339.49385073704));
#26525=CARTESIAN_POINT('Ctrl Pts',(208.023559698486,92.4897376097703,339.49385073704));
#26526=CARTESIAN_POINT('Ctrl Pts',(208.062763029538,92.503813085854,339.029080959744));
#26527=CARTESIAN_POINT('Ctrl Pts',(208.036816019941,92.5186621687676,338.560218780518));
#26528=CARTESIAN_POINT('Ctrl Pts',(207.819237647414,92.5549651861974,337.463074845365));
#26529=CARTESIAN_POINT('Ctrl Pts',(207.56949024203,92.576337573963,336.855936542507));
#26530=CARTESIAN_POINT('Ctrl Pts',(206.85171428554,92.6172023755726,335.771639663891));
#26531=CARTESIAN_POINT('Ctrl Pts',(206.390651310047,92.6365404256281,335.304767332239));
#26532=CARTESIAN_POINT('Ctrl Pts',(205.315040387593,92.6787225624914,334.573212485897));
#26533=CARTESIAN_POINT('Ctrl Pts',(204.710587265591,92.7001235808703,334.315769800306));
#26534=CARTESIAN_POINT('Ctrl Pts',(203.438632779674,92.74106078414,334.047312375077));
#26535=CARTESIAN_POINT('Ctrl Pts',(202.783410504634,92.7603147840207,334.038225280269));
#26536=CARTESIAN_POINT('Ctrl Pts',(201.504028352964,92.8024439697371,334.271393146257));
#26537=CARTESIAN_POINT('Ctrl Pts',(200.892227160201,92.8238732386862,334.512245249282));
#26538=CARTESIAN_POINT('Ctrl Pts',(199.797940959952,92.8648838432939,335.213378888698));
#26539=CARTESIAN_POINT('Ctrl Pts',(199.325269217626,92.8840589473803,335.665985013689));
#26540=CARTESIAN_POINT('Ctrl Pts',(198.577071554176,92.9261323728689,336.729251978811));
#26541=CARTESIAN_POINT('Ctrl Pts',(198.309796155385,92.9475893466673,337.330553540224));
#26542=CARTESIAN_POINT('Ctrl Pts',(198.022018744288,92.9886741004599,338.597611461723));
#26543=CARTESIAN_POINT('Ctrl Pts',(198.002619168953,93.007776237796,339.250907302441));
#26544=CARTESIAN_POINT('Ctrl Pts',(198.214788436499,93.0497911379274,340.53331005053));
#26545=CARTESIAN_POINT('Ctrl Pts',(198.446192384073,93.0712751059638,341.149880227393));
#26546=CARTESIAN_POINT('Ctrl Pts',(199.129759078033,93.1124344915023,342.254546141058));
#26547=CARTESIAN_POINT('Ctrl Pts',(199.573536121332,93.131470324171,342.733263264169));
#26548=CARTESIAN_POINT('Ctrl Pts',(200.623751002207,93.173424007641,343.498738697488));
#26549=CARTESIAN_POINT('Ctrl Pts',(201.221590068503,93.194934098379,343.776259350343));
#26550=CARTESIAN_POINT('Ctrl Pts',(202.483388821072,93.2361683229841,344.084186720265));
#26551=CARTESIAN_POINT('Ctrl Pts',(203.134680304963,93.2551451870716,344.114280628453));
#26552=CARTESIAN_POINT('Ctrl Pts',(204.420025246542,93.2970350674323,343.923946124849));
#26553=CARTESIAN_POINT('Ctrl Pts',(205.04140056564,93.3185702556276,343.702454501577));
#26554=CARTESIAN_POINT('Ctrl Pts',(206.156712318979,93.3598792453007,343.037206727527));
#26555=CARTESIAN_POINT('Ctrl Pts',(206.64165617648,93.3788050750477,342.602532781206));
#26556=CARTESIAN_POINT('Ctrl Pts',(207.424839088953,93.4206287022077,341.56594739536));
#26557=CARTESIAN_POINT('Ctrl Pts',(207.712895253196,93.4421878193285,340.971861730333));
#26558=CARTESIAN_POINT('Ctrl Pts',(207.951094625822,93.4721791769352,340.061455246487));
#26559=CARTESIAN_POINT('Ctrl Pts',(207.999539074984,93.4811132989645,339.778623982982));
#26560=CARTESIAN_POINT('Ctrl Pts',(208.023559698486,93.4897376097702,339.49385073704));
#26561=CARTESIAN_POINT('Origin',(203.041252647848,90.7397376070391,339.073593133703));
#26562=CARTESIAN_POINT('',(208.023559698486,94.4897376097702,339.49385073704));
#26563=CARTESIAN_POINT('',(208.023559698486,94.239737607039,339.49385073704));
#26564=CARTESIAN_POINT('',(208.023559698486,90.7397376070391,339.49385073704));
#26565=CARTESIAN_POINT('Ctrl Pts',(208.023559698486,94.2397376070391,339.49385073704));
#26566=CARTESIAN_POINT('Ctrl Pts',(208.010416806229,94.2350188124707,339.649664514677));
#26567=CARTESIAN_POINT('Ctrl Pts',(207.989949726939,94.2302028827843,339.805041669434));
#26568=CARTESIAN_POINT('Ctrl Pts',(207.847186504248,94.2050486441458,340.598070875467));
#26569=CARTESIAN_POINT('Ctrl Pts',(207.609006140685,94.1837711461655,341.208218819053));
#26570=CARTESIAN_POINT('Ctrl Pts',(206.910251725032,94.1413936065866,342.30750821154));
#26571=CARTESIAN_POINT('Ctrl Pts',(206.45475666335,94.1216554905342,342.785106712135));
#26572=CARTESIAN_POINT('Ctrl Pts',(205.390116506321,94.0810847559065,343.534909180295));
#26573=CARTESIAN_POINT('Ctrl Pts',(204.79234583872,94.0598357420271,343.801609538172));
#26574=CARTESIAN_POINT('Ctrl Pts',(203.52238779423,94.0174198117079,344.093253090569));
#26575=CARTESIAN_POINT('Ctrl Pts',(202.861825332427,93.997583565249,344.113063442553));
#26576=CARTESIAN_POINT('Ctrl Pts',(201.562180369908,93.9566078398427,343.895636535585));
#26577=CARTESIAN_POINT('Ctrl Pts',(200.93639988694,93.9348726148643,343.657184900668));
#26578=CARTESIAN_POINT('Ctrl Pts',(199.833965931474,93.8924634819524,342.962410051128));
#26579=CARTESIAN_POINT('Ctrl Pts',(199.363060303142,93.8730223740733,342.520397591058));
#26580=CARTESIAN_POINT('Ctrl Pts',(198.599711326465,93.8325669773609,341.463781129068));
#26581=CARTESIAN_POINT('Ctrl Pts',(198.322071276732,93.8108332685872,340.853922978363));
#26582=CARTESIAN_POINT('Ctrl Pts',(198.026390289346,93.7683883495924,339.584320308703));
#26583=CARTESIAN_POINT('Ctrl Pts',(198.002254957477,93.7488728393059,338.938836700015));
#26584=CARTESIAN_POINT('Ctrl Pts',(198.202341366308,93.7084797670189,337.65031087724));
#26585=CARTESIAN_POINT('Ctrl Pts',(198.433873038498,93.6867481919507,337.021081219462));
#26586=CARTESIAN_POINT('Ctrl Pts',(199.116706243766,93.6442697891709,335.910091099344));
#26587=CARTESIAN_POINT('Ctrl Pts',(199.553541446658,93.6246796835069,335.434136338493));
#26588=CARTESIAN_POINT('Ctrl Pts',(200.602320962549,93.5843464794912,334.658517829307));
#26589=CARTESIAN_POINT('Ctrl Pts',(201.209804236407,93.5626175563798,334.373909121373));
#26590=CARTESIAN_POINT('Ctrl Pts',(202.47709123836,93.5201078798684,334.064434339146));
#26591=CARTESIAN_POINT('Ctrl Pts',(203.122490723531,93.5004435265117,334.033423393591));
#26592=CARTESIAN_POINT('Ctrl Pts',(204.413959289153,93.4601676700277,334.219995156549));
#26593=CARTESIAN_POINT('Ctrl Pts',(205.046242389075,93.4384418242896,334.445234179375));
#26594=CARTESIAN_POINT('Ctrl Pts',(206.164915447719,93.3959029861141,335.117226760056));
#26595=CARTESIAN_POINT('Ctrl Pts',(206.64542795061,93.3761652142158,335.54939389652));
#26596=CARTESIAN_POINT('Ctrl Pts',(207.432061201653,93.3359441439206,336.591059618701));
#26597=CARTESIAN_POINT('Ctrl Pts',(207.722924153347,93.3142217152644,337.196340812184));
#26598=CARTESIAN_POINT('Ctrl Pts',(208.024304415469,93.274367399161,338.380885456566));
#26599=CARTESIAN_POINT('Ctrl Pts',(208.070307946708,93.2565219932672,338.939633216943));
#26600=CARTESIAN_POINT('Ctrl Pts',(208.023559698486,93.239737607039,339.49385073704));
#26601=CARTESIAN_POINT('Ctrl Pts',(208.023559698486,93.4897376097703,339.49385073704));
#26602=CARTESIAN_POINT('Ctrl Pts',(208.053467706927,93.5004757140647,339.13928039698));
#26603=CARTESIAN_POINT('Ctrl Pts',(208.045509564255,93.5116822219815,338.781728251426));
#26604=CARTESIAN_POINT('Ctrl Pts',(207.914698776637,93.5442095446849,337.778250092893));
#26605=CARTESIAN_POINT('Ctrl Pts',(207.703471833047,93.565791292366,337.152107083396));
#26606=CARTESIAN_POINT('Ctrl Pts',(207.057085527107,93.6072484595061,336.026022407149));
#26607=CARTESIAN_POINT('Ctrl Pts',(206.631676783548,93.6260979455809,335.534743749621));
#26608=CARTESIAN_POINT('Ctrl Pts',(205.609138567905,93.6677824164138,334.733651852745));
#26609=CARTESIAN_POINT('Ctrl Pts',(205.019063155191,93.6893853826483,334.434908324653));
#26610=CARTESIAN_POINT('Ctrl Pts',(203.768687207825,93.7309154070329,334.085139839588));
#26611=CARTESIAN_POINT('Ctrl Pts',(203.121532565595,93.7497402717904,334.033019530661));
#26612=CARTESIAN_POINT('Ctrl Pts',(201.830736440786,93.7913522630566,334.17823605667));
#26613=CARTESIAN_POINT('Ctrl Pts',(201.199936002383,93.8129749406107,334.378976721327));
#26614=CARTESIAN_POINT('Ctrl Pts',(200.063097911448,93.8545766580724,335.006197099869));
#26615=CARTESIAN_POINT('Ctrl Pts',(199.565455788559,93.8733861699124,335.422298491117));
#26616=CARTESIAN_POINT('Ctrl Pts',(198.746493044917,93.9149240864483,336.430554314477));
#26617=CARTESIAN_POINT('Ctrl Pts',(198.43705788505,93.9365648914709,337.016410161944));
#26618=CARTESIAN_POINT('Ctrl Pts',(198.066138750965,93.9782368879476,338.260751574102));
#26619=CARTESIAN_POINT('Ctrl Pts',(198.002966642329,93.9970403544056,338.905830082094));
#26620=CARTESIAN_POINT('Ctrl Pts',(198.125493048056,94.0385028711359,340.199055243097));
#26621=CARTESIAN_POINT('Ctrl Pts',(198.315669239932,94.0601601685294,340.83433527832));
#26622=CARTESIAN_POINT('Ctrl Pts',(198.923674631269,94.1019007900959,341.981760995852));
#26623=CARTESIAN_POINT('Ctrl Pts',(199.33054862406,94.1207074421516,342.485713525102));
#26624=CARTESIAN_POINT('Ctrl Pts',(200.32448278348,94.1620935167283,343.322270439877));
#26625=CARTESIAN_POINT('Ctrl Pts',(200.90596895485,94.1837656404107,343.64225289854));
#26626=CARTESIAN_POINT('Ctrl Pts',(202.14416501544,94.2255730245481,344.034097997918));
#26627=CARTESIAN_POINT('Ctrl Pts',(202.787202018954,94.2443918735921,344.108157061287));
#26628=CARTESIAN_POINT('Ctrl Pts',(204.082621116741,94.2857007687482,344.008001235342));
#26629=CARTESIAN_POINT('Ctrl Pts',(204.722144944031,94.3073860438215,343.828319305139));
#26630=CARTESIAN_POINT('Ctrl Pts',(205.879852883803,94.3492581431384,343.23931938036));
#26631=CARTESIAN_POINT('Ctrl Pts',(206.38998517162,94.3680978628903,342.8414728654));
#26632=CARTESIAN_POINT('Ctrl Pts',(207.243633680452,94.4093291548137,341.861702064357));
#26633=CARTESIAN_POINT('Ctrl Pts',(207.573877783122,94.4310259190769,341.284668113954));
#26634=CARTESIAN_POINT('Ctrl Pts',(207.909525740834,94.4651666382827,340.281623235055));
#26635=CARTESIAN_POINT('Ctrl Pts',(207.990143356593,94.4777398812994,339.890013648779));
#26636=CARTESIAN_POINT('Ctrl Pts',(208.023559698486,94.4897376097703,339.49385073704));
#26637=CARTESIAN_POINT('Origin',(203.041252647848,90.7397376070391,339.073593133703));
#26638=CARTESIAN_POINT('',(208.023559698486,95.4897376097703,339.49385073704));
#26639=CARTESIAN_POINT('',(208.023559698486,95.239737607039,339.49385073704));
#26640=CARTESIAN_POINT('',(208.023559698486,90.7397376070391,339.49385073704));
#26641=CARTESIAN_POINT('Ctrl Pts',(208.023559698486,95.239737607039,339.49385073704));
#26642=CARTESIAN_POINT('Ctrl Pts',(208.002184735619,95.2320631882956,339.747258711949));
#26643=CARTESIAN_POINT('Ctrl Pts',(207.961461981359,95.224140643241,339.99922146964));
#26644=CARTESIAN_POINT('Ctrl Pts',(207.748241493299,95.1953258739236,340.881988667412));
#26645=CARTESIAN_POINT('Ctrl Pts',(207.472228860018,95.1738232666891,341.480348925067));
#26646=CARTESIAN_POINT('Ctrl Pts',(206.709292797331,95.1318515425915,342.532497335783));
#26647=CARTESIAN_POINT('Ctrl Pts',(206.231465939511,95.1127971911816,342.977575255451));
#26648=CARTESIAN_POINT('Ctrl Pts',(205.1283260951,95.0716595022217,343.663742642687));
#26649=CARTESIAN_POINT('Ctrl Pts',(204.512452008966,95.0501832868781,343.896548980516));
#26650=CARTESIAN_POINT('Ctrl Pts',(203.230484038253,95.008151117896,344.111823287934));
#26651=CARTESIAN_POINT('Ctrl Pts',(202.576903215927,94.989028455691,344.093946787673));
#26652=CARTESIAN_POINT('Ctrl Pts',(201.309111357273,94.9479652863878,343.80902975649));
#26653=CARTESIAN_POINT('Ctrl Pts',(200.70733281563,94.9265162883599,343.543209633316));
#26654=CARTESIAN_POINT('Ctrl Pts',(199.642227731743,94.8844263903836,342.797471251603));
#26655=CARTESIAN_POINT('Ctrl Pts',(199.188369040292,94.8652289627601,342.32565784608));
#26656=CARTESIAN_POINT('Ctrl Pts',(198.484759138229,94.8242397523614,341.232848339848));
#26657=CARTESIAN_POINT('Ctrl Pts',(198.2425799626,94.8028186346644,340.621732038546));
#26658=CARTESIAN_POINT('Ctrl Pts',(198.006447420102,94.7606737885907,339.342791610849));
#26659=CARTESIAN_POINT('Ctrl Pts',(198.01407610868,94.7413958878486,338.687297565162));
#26660=CARTESIAN_POINT('Ctrl Pts',(198.279810342739,94.7004798138802,337.414664330447));
#26661=CARTESIAN_POINT('Ctrl Pts',(198.535866571647,94.6790870740884,336.809780215669));
#26662=CARTESIAN_POINT('Ctrl Pts',(199.265069544064,94.6368900963985,335.73244288771));
#26663=CARTESIAN_POINT('Ctrl Pts',(199.73112397612,94.6175267983182,335.270188525124));
#26664=CARTESIAN_POINT('Ctrl Pts',(200.814010005854,94.5766827909723,334.5500824108));
#26665=CARTESIAN_POINT('Ctrl Pts',(201.420484220555,94.5553187613266,334.299094057792));
#26666=CARTESIAN_POINT('Ctrl Pts',(202.696379945475,94.5130724765636,334.043182426579));
#26667=CARTESIAN_POINT('Ctrl Pts',(203.353685010861,94.4936196597669,334.041064225867));
#26668=CARTESIAN_POINT('Ctrl Pts',(204.630767916029,94.4528464191918,334.288658157108));
#26669=CARTESIAN_POINT('Ctrl Pts',(205.238439837012,94.4315112696395,334.535476741688));
#26670=CARTESIAN_POINT('Ctrl Pts',(206.32719185158,94.3892184852296,335.248974915445));
#26671=CARTESIAN_POINT('Ctrl Pts',(206.797378841282,94.3696728341906,335.709576758465));
#26672=CARTESIAN_POINT('Ctrl Pts',(207.532909923555,94.3289688501493,336.783047182977));
#26673=CARTESIAN_POINT('Ctrl Pts',(207.792083799821,94.3076625940288,337.385056061122));
#26674=CARTESIAN_POINT('Ctrl Pts',(208.033463659016,94.2704276874328,338.50455736156));
#26675=CARTESIAN_POINT('Ctrl Pts',(208.065101493989,94.254652680156,339.00135761143));
#26676=CARTESIAN_POINT('Ctrl Pts',(208.023559698486,94.239737607039,339.49385073704));
#26677=CARTESIAN_POINT('Ctrl Pts',(208.023559698486,94.4897376097702,339.49385073704));
#26678=CARTESIAN_POINT('Ctrl Pts',(208.043768367793,94.4969932850888,339.254269597342));
#26679=CARTESIAN_POINT('Ctrl Pts',(208.046713370765,94.504471619991,339.013036344154));
#26680=CARTESIAN_POINT('Ctrl Pts',(207.992401460983,94.5329829269995,338.11421889948));
#26681=CARTESIAN_POINT('Ctrl Pts',(207.822998666388,94.5546895512273,337.470732835158));
#26682=CARTESIAN_POINT('Ctrl Pts',(207.252545517764,94.5966843279668,336.303171643436));
#26683=CARTESIAN_POINT('Ctrl Pts',(206.863417586195,94.6155899329068,335.787063449034));
#26684=CARTESIAN_POINT('Ctrl Pts',(205.897461723054,94.6566660118852,334.917026478739));
#26685=CARTESIAN_POINT('Ctrl Pts',(205.324890950684,94.6783809183672,334.576932970826));
#26686=CARTESIAN_POINT('Ctrl Pts',(204.098967452958,94.7204334190671,334.144982523275));
#26687=CARTESIAN_POINT('Ctrl Pts',(203.45980384356,94.7393828773307,334.050170387513));
#26688=CARTESIAN_POINT('Ctrl Pts',(202.160744370393,94.7803819694335,334.107672237849));
#26689=CARTESIAN_POINT('Ctrl Pts',(201.513609429568,94.8021036483627,334.267144490897));
#26690=CARTESIAN_POINT('Ctrl Pts',(200.336726746597,94.844211349363,334.819735997519));
#26691=CARTESIAN_POINT('Ctrl Pts',(199.814910653824,94.8632110439442,335.200548522953));
#26692=CARTESIAN_POINT('Ctrl Pts',(198.929355509185,94.9041339614367,336.153209740886));
#26693=CARTESIAN_POINT('Ctrl Pts',(198.579930763012,94.9258609848434,336.721377403406));
#26694=CARTESIAN_POINT('Ctrl Pts',(198.129264059369,94.9680213100446,337.9413473242));
#26695=CARTESIAN_POINT('Ctrl Pts',(198.02480881621,94.9870768938179,338.578721474358));
#26696=CARTESIAN_POINT('Ctrl Pts',(198.062504346938,95.0279247298472,339.879233592402));
#26697=CARTESIAN_POINT('Ctrl Pts',(198.212509986815,95.0496557628878,340.529686371043));
#26698=CARTESIAN_POINT('Ctrl Pts',(198.748118246612,95.0918661086761,341.715280275465));
#26699=CARTESIAN_POINT('Ctrl Pts',(199.121094664281,95.1109824755923,342.242483631134));
#26700=CARTESIAN_POINT('Ctrl Pts',(200.061127156013,95.1517565849168,343.142558313204));
#26701=CARTESIAN_POINT('Ctrl Pts',(200.625017830817,95.1734903944396,343.500714594113));
#26702=CARTESIAN_POINT('Ctrl Pts',(201.839260640202,95.2157481529159,343.96896608168));
#26703=CARTESIAN_POINT('Ctrl Pts',(202.474963975221,95.2349294259626,344.082461960223));
#26704=CARTESIAN_POINT('Ctrl Pts',(203.776702189642,95.2756314027013,344.063317889121));
#26705=CARTESIAN_POINT('Ctrl Pts',(204.430137152372,95.2973668631158,343.922222439557));
#26706=CARTESIAN_POINT('Ctrl Pts',(205.623779055288,95.3396694432978,343.402566090827));
#26707=CARTESIAN_POINT('Ctrl Pts',(206.156009434055,95.3589189781057,343.036890373666));
#26708=CARTESIAN_POINT('Ctrl Pts',(207.069517447052,95.3995506311888,342.108706580024));
#26709=CARTESIAN_POINT('Ctrl Pts',(207.435749836129,95.4212867277573,341.548909322898));
#26710=CARTESIAN_POINT('Ctrl Pts',(207.867118588414,95.458981461004,340.47284835785));
#26711=CARTESIAN_POINT('Ctrl Pts',(207.981927662159,95.4747901367899,339.987413700515));
#26712=CARTESIAN_POINT('Ctrl Pts',(208.023559698486,95.4897376097703,339.49385073704));
#26713=CARTESIAN_POINT('Origin',(203.041252647848,90.7397376070391,339.073593133703));
#26714=CARTESIAN_POINT('',(208.023559698486,96.4897376097702,339.49385073704));
#26715=CARTESIAN_POINT('',(208.023559698486,96.2397376070391,339.49385073704));
#26716=CARTESIAN_POINT('',(208.023559698486,90.7397376070391,339.49385073704));
#26717=CARTESIAN_POINT('Ctrl Pts',(208.023559698486,96.239737607039,339.49385073704));
#26718=CARTESIAN_POINT('Ctrl Pts',(207.992788965512,96.2286897520627,339.858648990853));
#26719=CARTESIAN_POINT('Ctrl Pts',(207.92197943703,96.2171481933558,340.219775056907));
#26720=CARTESIAN_POINT('Ctrl Pts',(207.615114011323,96.1841690870811,341.197661696786));
#26721=CARTESIAN_POINT('Ctrl Pts',(207.296647798149,96.1625010943826,341.779788832638));
#26722=CARTESIAN_POINT('Ctrl Pts',(206.462618291474,96.12109274177,342.775796357516));
#26723=CARTESIAN_POINT('Ctrl Pts',(205.959575321926,96.1022879546357,343.183999868238));
#26724=CARTESIAN_POINT('Ctrl Pts',(204.813670409927,96.0605670693968,343.794787058174));
#26725=CARTESIAN_POINT('Ctrl Pts',(204.179027129829,96.0389143884731,343.986495650469));
#26726=CARTESIAN_POINT('Ctrl Pts',(202.886140400462,95.9974298653367,344.112302424058));
#26727=CARTESIAN_POINT('Ctrl Pts',(202.240762010827,95.9786256015654,344.050727383065));
#26728=CARTESIAN_POINT('Ctrl Pts',(200.995535928686,95.9369738439711,343.682870646351));
#26729=CARTESIAN_POINT('Ctrl Pts',(200.409056860537,95.9153381342076,343.374981703873));
#26730=CARTESIAN_POINT('Ctrl Pts',(199.398721120808,95.8737785691662,342.558601039208));
#26731=CARTESIAN_POINT('Ctrl Pts',(198.981270905831,95.8549655572264,342.061880964911));
#26732=CARTESIAN_POINT('Ctrl Pts',(198.351259785361,95.8133845163022,340.926596740914));
#26733=CARTESIAN_POINT('Ctrl Pts',(198.148988889215,95.7917674001189,340.296462727989));
#26734=CARTESIAN_POINT('Ctrl Pts',(198.000470813963,95.7501341935238,339.006037204878));
#26735=CARTESIAN_POINT('Ctrl Pts',(198.050981883652,95.7313031343742,338.358580322264));
#26736=CARTESIAN_POINT('Ctrl Pts',(198.397679001331,95.689794148103,337.107342611361));
#26737=CARTESIAN_POINT('Ctrl Pts',(198.694867641288,95.6681971894426,336.516670935736));
#26738=CARTESIAN_POINT('Ctrl Pts',(199.493357025268,95.6264920180173,335.492074911149));
#26739=CARTESIAN_POINT('Ctrl Pts',(199.983712583493,95.6076336653908,335.065315997816));
#26740=CARTESIAN_POINT('Ctrl Pts',(201.108231479152,95.5661978288938,334.416167513942));
#26741=CARTESIAN_POINT('Ctrl Pts',(201.733687698866,95.5446225092986,334.203433823101));
#26742=CARTESIAN_POINT('Ctrl Pts',(203.021447045494,95.5028473003782,334.032234906729));
#26743=CARTESIAN_POINT('Ctrl Pts',(203.670982588125,95.4839525958251,334.071680876363));
#26744=CARTESIAN_POINT('Ctrl Pts',(204.928029241843,95.442590742841,334.397319762798));
#26745=CARTESIAN_POINT('Ctrl Pts',(205.522676538958,95.4210384431454,334.683834055209));
#26746=CARTESIAN_POINT('Ctrl Pts',(206.561269974001,95.3791953419735,335.464428959567));
#26747=CARTESIAN_POINT('Ctrl Pts',(206.997277895647,95.3602555477126,335.948460603411));
#26748=CARTESIAN_POINT('Ctrl Pts',(207.665223302619,95.3189682353603,337.062216008946));
#26749=CARTESIAN_POINT('Ctrl Pts',(207.88817825794,95.297440217797,337.682894516322));
#26750=CARTESIAN_POINT('Ctrl Pts',(208.043677427071,95.2637698364477,338.715232680993));
#26751=CARTESIAN_POINT('Ctrl Pts',(208.056256739997,95.2514770795136,339.106215393474));
#26752=CARTESIAN_POINT('Ctrl Pts',(208.023559698486,95.239737607039,339.49385073704));
#26753=CARTESIAN_POINT('Ctrl Pts',(208.023559698486,95.4897376097703,339.49385073704));
#26754=CARTESIAN_POINT('Ctrl Pts',(208.035542263805,95.4940398031565,339.351793058128));
#26755=CARTESIAN_POINT('Ctrl Pts',(208.041462561782,95.4984229426763,339.209066621738));
#26756=CARTESIAN_POINT('Ctrl Pts',(208.040247657829,95.523515304071,338.403183597517));
#26757=CARTESIAN_POINT('Ctrl Pts',(207.907438736615,95.5452511338183,337.747095622329));
#26758=CARTESIAN_POINT('Ctrl Pts',(207.402593756487,95.5876357444217,336.546097118296));
#26759=CARTESIAN_POINT('Ctrl Pts',(207.043647495372,95.6070289008787,336.009226080566));
#26760=CARTESIAN_POINT('Ctrl Pts',(206.126452073802,95.6475260610186,335.083418894112));
#26761=CARTESIAN_POINT('Ctrl Pts',(205.570518321967,95.669260831511,334.709796433752));
#26762=CARTESIAN_POINT('Ctrl Pts',(204.366807565089,95.7116827696874,334.21020725588));
#26763=CARTESIAN_POINT('Ctrl Pts',(203.734057619306,95.7311498865385,334.080636839829));
#26764=CARTESIAN_POINT('Ctrl Pts',(202.430459439187,95.7715831732276,334.066857680717));
#26765=CARTESIAN_POINT('Ctrl Pts',(201.772032500655,95.7933161995137,334.192045533994));
#26766=CARTESIAN_POINT('Ctrl Pts',(200.564374593779,95.8357731071012,334.683285324514));
#26767=CARTESIAN_POINT('Ctrl Pts',(200.023262402187,95.8553147591124,335.036090056167));
#26768=CARTESIAN_POINT('Ctrl Pts',(199.086302193444,95.8956865729828,335.943204405379));
#26769=CARTESIAN_POINT('Ctrl Pts',(198.705983574932,95.9174172730076,336.495538568604));
#26770=CARTESIAN_POINT('Ctrl Pts',(198.192743707955,95.9599068792456,337.694528949623));
#26771=CARTESIAN_POINT('Ctrl Pts',(198.056182177743,95.9795230633547,338.326001488763));
#26772=CARTESIAN_POINT('Ctrl Pts',(198.028116087924,96.019835886017,339.63028254547));
#26773=CARTESIAN_POINT('Ctrl Pts',(198.146366380844,96.0415637748267,340.290755597831));
#26774=CARTESIAN_POINT('Ctrl Pts',(198.625232381097,96.08408390344,341.504388797045));
#26775=CARTESIAN_POINT('Ctrl Pts',(198.972483193822,96.1037740964638,342.049341216364));
#26776=CARTESIAN_POINT('Ctrl Pts',(199.870440162225,96.1440304655269,342.996326912094));
#26777=CARTESIAN_POINT('Ctrl Pts',(200.419460273735,96.1657551485722,343.382659145238));
#26778=CARTESIAN_POINT('Ctrl Pts',(201.614125354356,96.2083037228219,343.908204657125));
#26779=CARTESIAN_POINT('Ctrl Pts',(202.244450704624,96.2280669411377,344.051064528939));
#26780=CARTESIAN_POINT('Ctrl Pts',(203.549282441482,96.268269426818,344.091981841699));
#26781=CARTESIAN_POINT('Ctrl Pts',(204.211533659972,96.2899905926433,343.979988270638));
#26782=CARTESIAN_POINT('Ctrl Pts',(205.430486009242,96.3325656385476,343.51227456024));
#26783=CARTESIAN_POINT('Ctrl Pts',(205.97888624372,96.3524004981135,343.170004557191));
#26784=CARTESIAN_POINT('Ctrl Pts',(206.934812909489,96.3925516816892,342.280291170605));
#26785=CARTESIAN_POINT('Ctrl Pts',(207.326502801641,96.4142690942686,341.734289428821));
#26786=CARTESIAN_POINT('Ctrl Pts',(207.832866129487,96.454472222825,340.610535606034));
#26787=CARTESIAN_POINT('Ctrl Pts',(207.975973891469,96.4726525083101,340.057997821903));
#26788=CARTESIAN_POINT('Ctrl Pts',(208.023559698486,96.4897376097703,339.49385073704));
#26789=CARTESIAN_POINT('Origin',(203.041252647848,90.7397376070391,339.073593133703));
#26790=CARTESIAN_POINT('',(208.023559698486,97.4897376097703,339.49385073704));
#26791=CARTESIAN_POINT('',(208.023559698486,97.239737607039,339.49385073704));
#26792=CARTESIAN_POINT('',(208.023559698486,90.7397376070391,339.49385073704));
#26793=CARTESIAN_POINT('',(203.461510341368,97.739737607039,334.091286090672));
#26794=CARTESIAN_POINT('Ctrl Pts',(208.023559698486,97.4897376097703,339.49385073704));
#26795=CARTESIAN_POINT('Ctrl Pts',(208.026122456743,97.4906577367488,339.463468303909));
#26796=CARTESIAN_POINT('Ctrl Pts',(208.028408300908,97.4915817077204,339.43305061537));
#26797=CARTESIAN_POINT('Ctrl Pts',(208.074332770675,97.5127995193416,338.736640391277));
#26798=CARTESIAN_POINT('Ctrl Pts',(207.984466746736,97.5344812925574,338.06860228078));
#26799=CARTESIAN_POINT('Ctrl Pts',(207.5561645317,97.5772347898467,336.831354383881));
#26800=CARTESIAN_POINT('Ctrl Pts',(207.231321281585,97.5976600214372,336.270864071329));
#26801=CARTESIAN_POINT('Ctrl Pts',(206.370658555201,97.6374313462935,335.284041543343));
#26802=CARTESIAN_POINT('Ctrl Pts',(205.835545208142,97.6591095681029,334.873889238233));
#26803=CARTESIAN_POINT('Ctrl Pts',(204.679764352328,97.7011145474933,334.309334586702));
#26804=CARTESIAN_POINT('Ctrl Pts',(204.078139965998,97.7210630803458,334.143298811198));
#26805=CARTESIAN_POINT('Ctrl Pts',(203.461510341367,97.739737607039,334.091286090672));
#26806=CARTESIAN_POINT('',(198.05894559721,97.739737607039,338.653335530367));
#26807=CARTESIAN_POINT('Origin',(203.041252647848,97.739737607039,339.073593133703));
#26808=CARTESIAN_POINT('Ctrl Pts',(198.05894559721,97.739737607039,338.653335530367));
#26809=CARTESIAN_POINT('Ctrl Pts',(198.108214107373,97.7220483516143,338.069239386452));
#26810=CARTESIAN_POINT('Ctrl Pts',(198.259812626742,97.7032083417734,337.498354791864));
#26811=CARTESIAN_POINT('Ctrl Pts',(198.755574421492,97.6648102145717,336.431322092174));
#26812=CARTESIAN_POINT('Ctrl Pts',(199.097269421509,97.6455484329761,335.944110190914));
#26813=CARTESIAN_POINT('Ctrl Pts',(199.969816698936,97.607292294862,335.076622710325));
#26814=CARTESIAN_POINT('Ctrl Pts',(200.506038837376,97.5879204097589,334.716736066367));
#26815=CARTESIAN_POINT('Ctrl Pts',(201.70601300298,97.5455470870172,334.209815220194));
#26816=CARTESIAN_POINT('Ctrl Pts',(202.361735860209,97.5238110933426,334.075844224131));
#26817=CARTESIAN_POINT('Ctrl Pts',(203.664358449214,97.4832281495198,334.071475003247));
#26818=CARTESIAN_POINT('Ctrl Pts',(204.298734616266,97.4639285428047,334.192179097569));
#26819=CARTESIAN_POINT('Ctrl Pts',(205.508309937176,97.4215957040894,334.674473301726));
#26820=CARTESIAN_POINT('Ctrl Pts',(206.068687981791,97.3998596942166,335.039575687551));
#26821=CARTESIAN_POINT('Ctrl Pts',(206.998539556133,97.3592078266473,335.95120373491));
#26822=CARTESIAN_POINT('Ctrl Pts',(207.365240030686,97.3399784069158,336.482728028812));
#26823=CARTESIAN_POINT('Ctrl Pts',(207.887142855589,97.2976885717295,337.675244394378));
#26824=CARTESIAN_POINT('Ctrl Pts',(208.029494077743,97.2759534810375,338.328267227807));
#26825=CARTESIAN_POINT('Ctrl Pts',(208.043369207323,97.2499792315604,339.158452004541));
#26826=CARTESIAN_POINT('Ctrl Pts',(208.037667377192,97.244802796371,339.326599064431));
#26827=CARTESIAN_POINT('Ctrl Pts',(208.023559698486,97.2397376070391,339.49385073704));
#26828=CARTESIAN_POINT('Origin',(203.041252647848,90.7397376070391,339.073593133703));
#26829=CARTESIAN_POINT('Ctrl Pts',(208.023559698486,97.2397376070391,339.49385073704));
#26830=CARTESIAN_POINT('Ctrl Pts',(207.984072407315,97.2255601785509,339.961986965035));
#26831=CARTESIAN_POINT('Ctrl Pts',(207.878733270431,97.2106005068773,340.423058333001));
#26832=CARTESIAN_POINT('Ctrl Pts',(207.473249346603,97.1738244260834,341.480836170954));
#26833=CARTESIAN_POINT('Ctrl Pts',(207.116320666296,97.1520913016813,342.045337432396));
#26834=CARTESIAN_POINT('Ctrl Pts',(206.218287475554,97.1112959462238,342.987156700394));
#26835=CARTESIAN_POINT('Ctrl Pts',(205.691844425507,97.0921976813484,343.361238276784));
#26836=CARTESIAN_POINT('Ctrl Pts',(204.507474627792,97.0500015858584,343.899250516616));
#26837=CARTESIAN_POINT('Ctrl Pts',(203.857482527551,97.0282715850081,344.05059746488));
#26838=CARTESIAN_POINT('Ctrl Pts',(202.557166736546,96.9874020839181,344.091093101459));
#26839=CARTESIAN_POINT('Ctrl Pts',(201.919539958598,96.9683632608377,343.988001630071));
#26840=CARTESIAN_POINT('Ctrl Pts',(200.698718343136,96.9262179431037,343.539984552674));
#26841=CARTESIAN_POINT('Ctrl Pts',(200.129917988798,96.9044923291968,343.19187851264));
#26842=CARTESIAN_POINT('Ctrl Pts',(199.175365484415,96.8635474014795,342.308516192129));
#26843=CARTESIAN_POINT('Ctrl Pts',(198.793374274254,96.8445629039893,341.787509714422));
#26844=CARTESIAN_POINT('Ctrl Pts',(198.238240806987,96.8024709621138,340.611943598142));
#26845=CARTESIAN_POINT('Ctrl Pts',(198.077353598602,96.7807510980283,339.965317957328));
#26846=CARTESIAN_POINT('Ctrl Pts',(198.016882311117,96.7397297302301,338.666489160782));
#26847=CARTESIAN_POINT('Ctrl Pts',(198.110249291279,96.720793689799,338.027056762429));
#26848=CARTESIAN_POINT('Ctrl Pts',(198.539398866779,96.6787576872925,336.800254802914));
#26849=CARTESIAN_POINT('Ctrl Pts',(198.878092804007,96.6570450260351,336.227038361008));
#26850=CARTESIAN_POINT('Ctrl Pts',(199.745801725264,96.6159464905269,335.259105973311));
#26851=CARTESIAN_POINT('Ctrl Pts',(200.261057849086,96.5970523201022,334.868735662898));
#26852=CARTESIAN_POINT('Ctrl Pts',(201.427219829101,96.5550747605428,334.295628248824));
#26853=CARTESIAN_POINT('Ctrl Pts',(202.070149690122,96.5333708331789,334.124752260644));
#26854=CARTESIAN_POINT('Ctrl Pts',(203.367247441408,96.4921947026469,334.043247659781));
#26855=CARTESIAN_POINT('Ctrl Pts',(204.008587493501,96.4733351478506,334.12638067621));
#26856=CARTESIAN_POINT('Ctrl Pts',(205.241507999327,96.4314184484144,334.53572903349));
#26857=CARTESIAN_POINT('Ctrl Pts',(205.81919049922,96.4097248493973,334.86450662431));
#26858=CARTESIAN_POINT('Ctrl Pts',(206.800999585091,96.3684710070079,335.715713801429));
#26859=CARTESIAN_POINT('Ctrl Pts',(207.200139551435,96.349638214465,336.224960207563));
#26860=CARTESIAN_POINT('Ctrl Pts',(207.791875026247,96.3077846788651,337.381199760928));
#26861=CARTESIAN_POINT('Ctrl Pts',(207.973070003739,96.2861030489872,338.02012421056));
#26862=CARTESIAN_POINT('Ctrl Pts',(208.04718331331,96.2564700331562,338.948673262516));
#26863=CARTESIAN_POINT('Ctrl Pts',(208.046467436216,96.2479623498323,339.222271157521));
#26864=CARTESIAN_POINT('Ctrl Pts',(208.023559698486,96.2397376070391,339.49385073704));
#26865=CARTESIAN_POINT('Ctrl Pts',(208.023559698486,96.4897376097703,339.49385073704));
#26866=CARTESIAN_POINT('Ctrl Pts',(208.029723508158,96.4919506501753,339.42077652697));
#26867=CARTESIAN_POINT('Ctrl Pts',(208.034284582085,96.494185613006,339.347508739407));
#26868=CARTESIAN_POINT('Ctrl Pts',(208.063924596539,96.516875971816,338.608972787657));
#26869=CARTESIAN_POINT('Ctrl Pts',(207.957526488708,96.5385894627631,337.945184750735));
#26870=CARTESIAN_POINT('Ctrl Pts',(207.499782065111,96.581211947686,336.721530599689));
#26871=CARTESIAN_POINT('Ctrl Pts',(207.161945349506,96.6011846285669,336.17005856649));
#26872=CARTESIAN_POINT('Ctrl Pts',(206.279592795086,96.6412409005394,335.206214374461));
#26873=CARTESIAN_POINT('Ctrl Pts',(205.736313511846,96.6629503613836,334.809785055021));
#26874=CARTESIAN_POINT('Ctrl Pts',(204.549100349265,96.7055940218374,334.263472632413));
#26875=CARTESIAN_POINT('Ctrl Pts',(203.920702461476,96.7256323670771,334.109989051609));
#26876=CARTESIAN_POINT('Ctrl Pts',(202.615078789907,96.7656449626129,334.047443538443));
#26877=CARTESIAN_POINT('Ctrl Pts',(201.949968540392,96.787350337298,334.148875006118));
#26878=CARTESIAN_POINT('Ctrl Pts',(200.722184066173,96.8300136134775,334.597772957799));
#26879=CARTESIAN_POINT('Ctrl Pts',(200.167994064226,96.8501152007867,334.931690311607));
#26880=CARTESIAN_POINT('Ctrl Pts',(199.197182607504,96.8900865715947,335.807517898597));
#26881=CARTESIAN_POINT('Ctrl Pts',(198.796587014991,96.9117878493224,336.348362849379));
#26882=CARTESIAN_POINT('Ctrl Pts',(198.241665087836,96.9544692803354,337.532429750623));
#26883=CARTESIAN_POINT('Ctrl Pts',(198.083778098994,96.9746315520822,338.160031382078));
#26884=CARTESIAN_POINT('Ctrl Pts',(198.012287620772,97.0145640846887,339.4659334706));
#26885=CARTESIAN_POINT('Ctrl Pts',(198.109339878621,97.0362612931975,340.13217709862));
#26886=CARTESIAN_POINT('Ctrl Pts',(198.550438928581,97.0789595137171,341.36357013281));
#26887=CARTESIAN_POINT('Ctrl Pts',(198.880912065787,97.0991798182293,341.920150291995));
#26888=CARTESIAN_POINT('Ctrl Pts',(199.750992859848,97.1390758249433,342.897058847645));
#26889=CARTESIAN_POINT('Ctrl Pts',(200.289677786506,97.1607690242843,343.301296724813));
#26890=CARTESIAN_POINT('Ctrl Pts',(201.470958966748,97.2034827607414,343.863765735229));
#26891=CARTESIAN_POINT('Ctrl Pts',(202.097863816094,97.2237583890752,344.025512719996));
#26892=CARTESIAN_POINT('Ctrl Pts',(203.403986190896,97.2636201008004,344.104834054828));
#26893=CARTESIAN_POINT('Ctrl Pts',(204.071198444298,97.2853093776467,344.011620455692));
#26894=CARTESIAN_POINT('Ctrl Pts',(205.305729222954,97.3280374440981,343.57735712454));
#26895=CARTESIAN_POINT('Ctrl Pts',(205.864399867483,97.3483656623101,343.249894588557));
#26896=CARTESIAN_POINT('Ctrl Pts',(206.846618092953,97.3881952230552,342.384846483844));
#26897=CARTESIAN_POINT('Ctrl Pts',(207.254024869897,97.4098806855625,341.848065254827));
#26898=CARTESIAN_POINT('Ctrl Pts',(207.809808680381,97.451625474599,340.696719088236));
#26899=CARTESIAN_POINT('Ctrl Pts',(207.972228684743,97.4713078376846,340.102398612571));
#26900=CARTESIAN_POINT('Ctrl Pts',(208.023559698486,97.4897376097703,339.49385073704));
#26901=CARTESIAN_POINT('Origin',(203.041252647848,90.7397376070391,339.073593133703));
#26902=CARTESIAN_POINT('',(213.005866749124,88.7397376070391,339.914108340376));
#26903=CARTESIAN_POINT('Origin',(203.041252647848,88.7397376070391,339.073593133703));
#26904=CARTESIAN_POINT('',(213.005866749124,90.7397376070391,339.914108340376));
#26905=CARTESIAN_POINT('',(213.005866749124,90.7397376070391,339.914108340376));
#26906=CARTESIAN_POINT('Origin',(203.041252647848,90.7397376070391,339.073593133703));
#26907=CARTESIAN_POINT('Origin',(203.041252647848,97.739737607039,339.073593133703));
#26908=CARTESIAN_POINT('',(199.42962580375,97.739737607039,347.299137232417));
#26909=CARTESIAN_POINT('',(205.224003640602,97.739737607039,347.787893007159));
#26910=CARTESIAN_POINT('',(197.436702983495,97.739737607039,347.131034191082));
#26911=CARTESIAN_POINT('',(208.358969375234,97.739737607039,346.314125779038));
#26912=CARTESIAN_POINT('',(206.791486507918,97.739737607039,347.051009393099));
#26913=CARTESIAN_POINT('',(211.679433210834,97.739737607039,341.54042526057));
#26914=CARTESIAN_POINT('',(207.216926460858,97.739737607039,347.955996048494));
#26915=CARTESIAN_POINT('',(211.970596219332,97.739737607039,338.088581680325));
#26916=CARTESIAN_POINT('',(211.825014715083,97.739737607039,339.814503470448));
#26917=CARTESIAN_POINT('',(209.496682218079,97.739737607039,332.826125387114));
#26918=CARTESIAN_POINT('',(212.82147612521,97.739737607039,339.898554991115));
#26919=CARTESIAN_POINT('',(206.652879491945,97.7397376070391,330.84804903499));
#26920=CARTESIAN_POINT('',(208.074780855012,97.739737607039,331.837087211052));
#26921=CARTESIAN_POINT('',(200.858501655094,97.7397376070391,330.359293260247));
#26922=CARTESIAN_POINT('',(208.645802312201,97.7397376070391,331.016152076324));
#26923=CARTESIAN_POINT('',(197.723535920462,97.739737607039,331.833060488368));
#26924=CARTESIAN_POINT('',(199.291018787778,97.7397376070391,331.096176874308));
#26925=CARTESIAN_POINT('',(194.403072084862,97.739737607039,336.606761006836));
#26926=CARTESIAN_POINT('',(198.865578834838,97.7397376070391,330.191190218913));
#26927=CARTESIAN_POINT('',(194.111909076364,97.739737607039,340.058604587082));
#26928=CARTESIAN_POINT('',(194.257490580613,97.739737607039,338.332682796959));
#26929=CARTESIAN_POINT('',(196.585823077617,97.739737607039,345.321060880292));
#26930=CARTESIAN_POINT('',(193.261029170486,97.739737607039,338.248631276292));
#26931=CARTESIAN_POINT('',(198.007724440684,97.739737607039,346.310099056355));
#26932=CARTESIAN_POINT('Ctrl Pts',(204.724000912662,97.739737607039,344.353175103396));
#26933=CARTESIAN_POINT('Ctrl Pts',(204.228206354228,97.739737607039,344.483763605689));
#26934=CARTESIAN_POINT('Ctrl Pts',(203.716680544754,97.7397376070576,344.544816894783));
#26935=CARTESIAN_POINT('Ctrl Pts',(202.823445454301,97.7397376070576,344.527012055876));
#26936=CARTESIAN_POINT('Ctrl Pts',(202.280691335722,97.7397376070391,344.478986669827));
#26937=CARTESIAN_POINT('Ctrl Pts',(200.995881515023,97.7397376070391,344.06556316677));
#26938=CARTESIAN_POINT('Ctrl Pts',(200.383354713341,97.7397376070391,343.725835780105));
#26939=CARTESIAN_POINT('Ctrl Pts',(199.471189684133,97.7397376070391,342.955161691881));
#26940=CARTESIAN_POINT('Ctrl Pts',(198.962966730132,97.7397376070398,342.435039038614));
#26941=CARTESIAN_POINT('Ctrl Pts',(198.336602864625,97.7397376070398,341.211676486358));
#26942=CARTESIAN_POINT('Ctrl Pts',(198.172351502433,97.739737607039,340.718613950579));
#26943=CARTESIAN_POINT('Ctrl Pts',(197.977751507247,97.739737607039,339.584101577175));
#26944=CARTESIAN_POINT('Ctrl Pts',(198.004985132087,97.739737607039,339.046563828707));
#26945=CARTESIAN_POINT('Ctrl Pts',(198.05894559721,97.739737607039,338.653335530367));
#26946=CARTESIAN_POINT('Ctrl Pts',(203.461510341368,97.739737607039,334.091286090672));
#26947=CARTESIAN_POINT('Ctrl Pts',(203.984159147494,97.739737607039,334.107979462843));
#26948=CARTESIAN_POINT('Ctrl Pts',(204.501119720434,97.739737607039,334.204906851929));
#26949=CARTESIAN_POINT('Ctrl Pts',(205.482808994414,97.739737607039,334.550879748362));
#26950=CARTESIAN_POINT('Ctrl Pts',(205.94223007391,97.7397376070383,334.796447456792));
#26951=CARTESIAN_POINT('Ctrl Pts',(207.010186372729,97.7397376070383,335.596363647632));
#26952=CARTESIAN_POINT('Ctrl Pts',(207.443993549644,97.739737607039,336.165426518184));
#26953=CARTESIAN_POINT('Ctrl Pts',(208.075942876397,97.739737607039,337.239425210693));
#26954=CARTESIAN_POINT('Ctrl Pts',(208.307395377785,97.739737607039,337.900716986882));
#26955=CARTESIAN_POINT('Ctrl Pts',(208.478391743638,97.739737607039,339.100710339751));
#26956=CARTESIAN_POINT('Ctrl Pts',(208.47697792236,97.7397376070082,339.621944596309));
#26957=CARTESIAN_POINT('Ctrl Pts',(208.32126756147,97.7397376070082,340.658543246856));
#26958=CARTESIAN_POINT('Ctrl Pts',(208.175600019025,97.739737607039,341.151251001225));
#26959=CARTESIAN_POINT('Ctrl Pts',(207.964363569528,97.739737607039,341.616938637223));
#26960=CARTESIAN_POINT('Origin',(203.041252647848,90.7397376070391,339.073593133703));
#26961=CARTESIAN_POINT('',(197.436702983495,90.7397376070391,347.131034191082));
#26962=CARTESIAN_POINT('',(207.216926460858,90.7397376070391,347.955996048494));
#26963=CARTESIAN_POINT('',(197.436702983495,90.7397376070391,347.131034191082));
#26964=CARTESIAN_POINT('',(193.261029170486,90.7397376070391,338.248631276292));
#26965=CARTESIAN_POINT('',(193.261029170486,90.7397376070391,338.248631276292));
#26966=CARTESIAN_POINT('',(198.865578834838,90.7397376070391,330.191190218913));
#26967=CARTESIAN_POINT('',(198.865578834838,90.7397376070391,330.191190218913));
#26968=CARTESIAN_POINT('',(208.645802312201,90.7397376070391,331.016152076324));
#26969=CARTESIAN_POINT('',(208.645802312201,90.7397376070391,331.016152076324));
#26970=CARTESIAN_POINT('',(212.82147612521,90.7397376070391,339.898554991115));
#26971=CARTESIAN_POINT('',(212.82147612521,90.7397376070391,339.898554991115));
#26972=CARTESIAN_POINT('',(207.216926460858,90.7397376070391,347.955996048494));
#26973=CARTESIAN_POINT('Origin',(203.041252647848,88.7397376070391,339.073593133703));
#26974=CARTESIAN_POINT('Origin',(197.436702983495,97.739737607039,347.131034191082));
#26975=CARTESIAN_POINT('',(207.216926460858,95.7397376070391,347.955996048494));
#26976=CARTESIAN_POINT('',(201.330353312049,101.647214895151,347.459463599121));
#26977=CARTESIAN_POINT('',(197.436702983495,95.7397376070391,347.131034191082));
#26978=CARTESIAN_POINT('',(198.433164393623,96.739737607039,347.21508571175));
#26979=CARTESIAN_POINT('',(197.436702983495,97.739737607039,347.131034191082));
#26980=CARTESIAN_POINT('',(207.216926460858,97.739737607039,347.955996048494));
#26981=CARTESIAN_POINT('Origin',(207.216926460858,97.739737607039,347.955996048494));
#26982=CARTESIAN_POINT('',(207.787947918046,96.7397376070391,347.135060913766));
#26983=CARTESIAN_POINT('',(212.82147612521,95.7397376070391,339.898554991115));
#26984=CARTESIAN_POINT('',(212.82147612521,97.739737607039,339.898554991115));
#26985=CARTESIAN_POINT('',(209.448179835846,101.647214895151,344.748210654532));
#26986=CARTESIAN_POINT('Origin',(212.82147612521,97.739737607039,339.898554991115));
#26987=CARTESIAN_POINT('',(208.645802312201,95.7397376070391,331.016152076324));
#26988=CARTESIAN_POINT('',(211.159079171645,101.647214895151,336.362340189115));
#26989=CARTESIAN_POINT('',(212.396036172271,96.739737607039,338.99356833572));
#26990=CARTESIAN_POINT('',(208.645802312201,97.7397376070391,331.016152076324));
#26991=CARTESIAN_POINT('Origin',(208.645802312201,97.7397376070391,331.016152076324));
#26992=CARTESIAN_POINT('',(207.649340902073,96.7397376070391,330.932100555657));
#26993=CARTESIAN_POINT('',(198.865578834838,95.7397376070391,330.191190218913));
#26994=CARTESIAN_POINT('',(198.865578834838,97.7397376070391,330.191190218913));
#26995=CARTESIAN_POINT('',(204.752151983647,101.647214895151,330.687722668286));
#26996=CARTESIAN_POINT('Origin',(198.865578834838,97.7397376070391,330.191190218913));
#26997=CARTESIAN_POINT('',(193.261029170486,95.7397376070391,338.248631276292));
#26998=CARTESIAN_POINT('',(196.63432545985,101.647214895151,333.398975612875));
#26999=CARTESIAN_POINT('',(198.29455737765,96.7397376070391,331.012125353641));
#27000=CARTESIAN_POINT('',(193.261029170486,97.739737607039,338.248631276292));
#27001=CARTESIAN_POINT('Origin',(193.261029170486,97.739737607039,338.248631276292));
#27002=CARTESIAN_POINT('',(194.923426124051,101.647214895151,341.784846078292));
#27003=CARTESIAN_POINT('',(193.686469123425,96.739737607039,339.153617931687));
#27004=CARTESIAN_POINT('Origin',(197.519595040153,89.3647376084047,338.607841310488));
#27005=CARTESIAN_POINT('',(197.789270318682,89.1459876090874,338.630588420428));
#27006=CARTESIAN_POINT('',(197.789270318682,89.5834876077218,338.630588420428));
#27007=CARTESIAN_POINT('Origin',(203.041252647848,99.3647376084047,339.073593133703));
#27008=CARTESIAN_POINT('Ctrl Pts',(208.562910255543,90.9272376084047,339.539344956919));
#27009=CARTESIAN_POINT('Ctrl Pts',(208.369989533667,90.8647376084047,341.826490424806));
#27010=CARTESIAN_POINT('Ctrl Pts',(206.616317913094,90.8022376084047,343.30733094404));
#27011=CARTESIAN_POINT('Ctrl Pts',(204.86264629252,90.7397376084047,344.788171463274));
#27012=CARTESIAN_POINT('Ctrl Pts',(202.575500824633,90.6772376084047,344.595250741398));
#27013=CARTESIAN_POINT('Ctrl Pts',(200.288355356745,90.6147376084047,344.402330019522));
#27014=CARTESIAN_POINT('Ctrl Pts',(198.807514837511,90.5522376084047,342.648658398949));
#27015=CARTESIAN_POINT('Ctrl Pts',(197.326674318278,90.4897376084047,340.894986778376));
#27016=CARTESIAN_POINT('Ctrl Pts',(197.519595040153,90.4272376084047,338.607841310488));
#27017=CARTESIAN_POINT('Ctrl Pts',(197.712515762029,90.3647376084047,336.320695842601));
#27018=CARTESIAN_POINT('Ctrl Pts',(199.466187382602,90.3022376084047,334.839855323367));
#27019=CARTESIAN_POINT('Ctrl Pts',(201.219859003176,90.2397376084047,333.359014804133));
#27020=CARTESIAN_POINT('Ctrl Pts',(203.507004471063,90.1772376084047,333.551935526009));
#27021=CARTESIAN_POINT('Ctrl Pts',(205.794149938951,90.1147376084047,333.744856247885));
#27022=CARTESIAN_POINT('Ctrl Pts',(207.274990458185,90.0522376084047,335.498527868458));
#27023=CARTESIAN_POINT('Ctrl Pts',(208.755830977418,89.9897376084047,337.252199489031));
#27024=CARTESIAN_POINT('Ctrl Pts',(208.562910255543,89.9272376084047,339.539344956919));
#27025=CARTESIAN_POINT('Ctrl Pts',(208.562910255543,90.8022376084047,339.539344956919));
#27026=CARTESIAN_POINT('Ctrl Pts',(208.369989533667,90.7397376084047,341.826490424806));
#27027=CARTESIAN_POINT('Ctrl Pts',(206.616317913094,90.6772376084047,343.30733094404));
#27028=CARTESIAN_POINT('Ctrl Pts',(204.86264629252,90.6147376084047,344.788171463274));
#27029=CARTESIAN_POINT('Ctrl Pts',(202.575500824633,90.5522376084047,344.595250741398));
#27030=CARTESIAN_POINT('Ctrl Pts',(200.288355356745,90.4897376084047,344.402330019522));
#27031=CARTESIAN_POINT('Ctrl Pts',(198.807514837511,90.4272376084047,342.648658398949));
#27032=CARTESIAN_POINT('Ctrl Pts',(197.326674318278,90.3647376084047,340.894986778376));
#27033=CARTESIAN_POINT('Ctrl Pts',(197.519595040153,90.3022376084047,338.607841310488));
#27034=CARTESIAN_POINT('Ctrl Pts',(197.712515762029,90.2397376084047,336.320695842601));
#27035=CARTESIAN_POINT('Ctrl Pts',(199.466187382602,90.1772376084047,334.839855323367));
#27036=CARTESIAN_POINT('Ctrl Pts',(201.219859003176,90.1147376084047,333.359014804133));
#27037=CARTESIAN_POINT('Ctrl Pts',(203.507004471063,90.0522376084047,333.551935526009));
#27038=CARTESIAN_POINT('Ctrl Pts',(205.794149938951,89.9897376084047,333.744856247885));
#27039=CARTESIAN_POINT('Ctrl Pts',(207.274990458185,89.9272376084047,335.498527868458));
#27040=CARTESIAN_POINT('Ctrl Pts',(208.755830977418,89.8647376084047,337.252199489031));
#27041=CARTESIAN_POINT('Ctrl Pts',(208.562910255543,89.8022376084047,339.539344956919));
#27042=CARTESIAN_POINT('Ctrl Pts',(198.05894559721,99.7397376070391,338.653335530367));
#27043=CARTESIAN_POINT('Ctrl Pts',(198.233021996202,99.677237607039,336.589596378086));
#27044=CARTESIAN_POINT('Ctrl Pts',(199.815396547552,99.614737607039,335.253403031079));
#27045=CARTESIAN_POINT('Ctrl Pts',(201.397771098903,99.5522376070391,333.917209684073));
#27046=CARTESIAN_POINT('Ctrl Pts',(203.461510251184,99.4897376070391,334.091286083065));
#27047=CARTESIAN_POINT('Ctrl Pts',(205.525249403466,99.4272376070391,334.265362482058));
#27048=CARTESIAN_POINT('Ctrl Pts',(206.861442750472,99.364737607039,335.847737033408));
#27049=CARTESIAN_POINT('Ctrl Pts',(208.197636097478,99.3022376070391,337.430111584758));
#27050=CARTESIAN_POINT('Ctrl Pts',(208.023559698486,99.239737607039,339.49385073704));
#27051=CARTESIAN_POINT('Ctrl Pts',(207.849483299494,99.1772376070391,341.557589889321));
#27052=CARTESIAN_POINT('Ctrl Pts',(206.267108748143,99.1147376070391,342.893783236327));
#27053=CARTESIAN_POINT('Ctrl Pts',(204.684734196793,99.0522376070391,344.229976583334));
#27054=CARTESIAN_POINT('Ctrl Pts',(202.620995044512,98.989737607039,344.055900184342));
#27055=CARTESIAN_POINT('Ctrl Pts',(200.55725589223,98.9272376070391,343.881823785349));
#27056=CARTESIAN_POINT('Ctrl Pts',(199.221062545224,98.8647376070391,342.299449233999));
#27057=CARTESIAN_POINT('Ctrl Pts',(197.884869198218,98.8022376070391,340.717074682649));
#27058=CARTESIAN_POINT('Ctrl Pts',(198.05894559721,98.739737607039,338.653335530367));
#27059=CARTESIAN_POINT('Ctrl Pts',(198.233021996202,98.6772376070391,336.589596378086));
#27060=CARTESIAN_POINT('Ctrl Pts',(199.815396547552,98.6147376070391,335.253403031079));
#27061=CARTESIAN_POINT('Ctrl Pts',(201.397771098903,98.5522376070391,333.917209684073));
#27062=CARTESIAN_POINT('Ctrl Pts',(203.461510251184,98.4897376070391,334.091286083065));
#27063=CARTESIAN_POINT('Ctrl Pts',(205.525249403466,98.4272376070391,334.265362482058));
#27064=CARTESIAN_POINT('Ctrl Pts',(206.861442750472,98.3647376070391,335.847737033408));
#27065=CARTESIAN_POINT('Ctrl Pts',(208.197636097478,98.3022376070391,337.430111584758));
#27066=CARTESIAN_POINT('Ctrl Pts',(208.023559698486,98.2397376070391,339.49385073704));
#27067=CARTESIAN_POINT('Ctrl Pts',(207.849483299494,98.1772376070391,341.557589889321));
#27068=CARTESIAN_POINT('Ctrl Pts',(206.267108748143,98.1147376070391,342.893783236327));
#27069=CARTESIAN_POINT('Ctrl Pts',(204.684734196793,98.0522376070391,344.229976583334));
#27070=CARTESIAN_POINT('Ctrl Pts',(202.620995044512,97.989737607039,344.055900184342));
#27071=CARTESIAN_POINT('Ctrl Pts',(200.55725589223,97.9272376070391,343.881823785349));
#27072=CARTESIAN_POINT('Ctrl Pts',(199.221062545224,97.8647376070391,342.299449233999));
#27073=CARTESIAN_POINT('Ctrl Pts',(197.884869198218,97.8022376070391,340.717074682649));
#27074=CARTESIAN_POINT('Ctrl Pts',(198.05894559721,97.739737607039,338.653335530367));
#27075=CARTESIAN_POINT('Ctrl Pts',(198.233021996202,97.6772376070391,336.589596378086));
#27076=CARTESIAN_POINT('Ctrl Pts',(199.815396547552,97.6147376070391,335.253403031079));
#27077=CARTESIAN_POINT('Ctrl Pts',(201.397771098903,97.5522376070391,333.917209684073));
#27078=CARTESIAN_POINT('Ctrl Pts',(203.461510251184,97.489737607039,334.091286083065));
#27079=CARTESIAN_POINT('Ctrl Pts',(205.525249403466,97.4272376070391,334.265362482058));
#27080=CARTESIAN_POINT('Ctrl Pts',(206.861442750472,97.3647376070391,335.847737033408));
#27081=CARTESIAN_POINT('Ctrl Pts',(208.197636097478,97.3022376070391,337.430111584758));
#27082=CARTESIAN_POINT('Ctrl Pts',(208.023559698486,97.2397376070391,339.49385073704));
#27083=CARTESIAN_POINT('Ctrl Pts',(207.849483299494,97.1772376070391,341.557589889321));
#27084=CARTESIAN_POINT('Ctrl Pts',(206.267108748143,97.1147376070391,342.893783236327));
#27085=CARTESIAN_POINT('Ctrl Pts',(204.684734196793,97.0522376070391,344.229976583334));
#27086=CARTESIAN_POINT('Ctrl Pts',(202.620995044512,96.9897376070391,344.055900184342));
#27087=CARTESIAN_POINT('Ctrl Pts',(200.55725589223,96.9272376070391,343.881823785349));
#27088=CARTESIAN_POINT('Ctrl Pts',(199.221062545224,96.8647376070391,342.299449233999));
#27089=CARTESIAN_POINT('Ctrl Pts',(197.884869198218,96.8022376070391,340.717074682649));
#27090=CARTESIAN_POINT('Ctrl Pts',(198.05894559721,96.739737607039,338.653335530367));
#27091=CARTESIAN_POINT('Ctrl Pts',(198.233021996202,96.6772376070391,336.589596378086));
#27092=CARTESIAN_POINT('Ctrl Pts',(199.815396547552,96.6147376070391,335.253403031079));
#27093=CARTESIAN_POINT('Ctrl Pts',(201.397771098903,96.552237607039,333.917209684073));
#27094=CARTESIAN_POINT('Ctrl Pts',(203.461510251184,96.4897376070391,334.091286083065));
#27095=CARTESIAN_POINT('Ctrl Pts',(205.525249403466,96.4272376070391,334.265362482058));
#27096=CARTESIAN_POINT('Ctrl Pts',(206.861442750472,96.3647376070391,335.847737033408));
#27097=CARTESIAN_POINT('Ctrl Pts',(208.197636097478,96.3022376070391,337.430111584758));
#27098=CARTESIAN_POINT('Ctrl Pts',(208.023559698486,96.2397376070391,339.49385073704));
#27099=CARTESIAN_POINT('Ctrl Pts',(207.849483299494,96.1772376070391,341.557589889321));
#27100=CARTESIAN_POINT('Ctrl Pts',(206.267108748143,96.1147376070391,342.893783236327));
#27101=CARTESIAN_POINT('Ctrl Pts',(204.684734196793,96.0522376070391,344.229976583334));
#27102=CARTESIAN_POINT('Ctrl Pts',(202.620995044512,95.9897376070391,344.055900184342));
#27103=CARTESIAN_POINT('Ctrl Pts',(200.55725589223,95.9272376070391,343.881823785349));
#27104=CARTESIAN_POINT('Ctrl Pts',(199.221062545224,95.8647376070391,342.299449233999));
#27105=CARTESIAN_POINT('Ctrl Pts',(197.884869198218,95.8022376070391,340.717074682649));
#27106=CARTESIAN_POINT('Ctrl Pts',(198.05894559721,95.7397376070391,338.653335530367));
#27107=CARTESIAN_POINT('Ctrl Pts',(198.233021996202,95.6772376070391,336.589596378086));
#27108=CARTESIAN_POINT('Ctrl Pts',(199.815396547552,95.6147376070391,335.253403031079));
#27109=CARTESIAN_POINT('Ctrl Pts',(201.397771098903,95.5522376070391,333.917209684073));
#27110=CARTESIAN_POINT('Ctrl Pts',(203.461510251184,95.4897376070391,334.091286083065));
#27111=CARTESIAN_POINT('Ctrl Pts',(205.525249403466,95.4272376070391,334.265362482058));
#27112=CARTESIAN_POINT('Ctrl Pts',(206.861442750472,95.3647376070391,335.847737033408));
#27113=CARTESIAN_POINT('Ctrl Pts',(208.197636097478,95.3022376070391,337.430111584758));
#27114=CARTESIAN_POINT('Ctrl Pts',(208.023559698486,95.2397376070391,339.49385073704));
#27115=CARTESIAN_POINT('Ctrl Pts',(207.849483299494,95.1772376070391,341.557589889321));
#27116=CARTESIAN_POINT('Ctrl Pts',(206.267108748143,95.1147376070391,342.893783236327));
#27117=CARTESIAN_POINT('Ctrl Pts',(204.684734196793,95.0522376070391,344.229976583334));
#27118=CARTESIAN_POINT('Ctrl Pts',(202.620995044512,94.9897376070391,344.055900184342));
#27119=CARTESIAN_POINT('Ctrl Pts',(200.55725589223,94.9272376070391,343.881823785349));
#27120=CARTESIAN_POINT('Ctrl Pts',(199.221062545224,94.8647376070391,342.299449233999));
#27121=CARTESIAN_POINT('Ctrl Pts',(197.884869198218,94.8022376070391,340.717074682649));
#27122=CARTESIAN_POINT('Ctrl Pts',(198.05894559721,94.7397376070391,338.653335530367));
#27123=CARTESIAN_POINT('Ctrl Pts',(198.233021996202,94.6772376070391,336.589596378086));
#27124=CARTESIAN_POINT('Ctrl Pts',(199.815396547552,94.6147376070391,335.253403031079));
#27125=CARTESIAN_POINT('Ctrl Pts',(201.397771098903,94.5522376070391,333.917209684073));
#27126=CARTESIAN_POINT('Ctrl Pts',(203.461510251184,94.4897376070391,334.091286083065));
#27127=CARTESIAN_POINT('Ctrl Pts',(205.525249403466,94.4272376070391,334.265362482058));
#27128=CARTESIAN_POINT('Ctrl Pts',(206.861442750472,94.3647376070391,335.847737033408));
#27129=CARTESIAN_POINT('Ctrl Pts',(208.197636097478,94.3022376070391,337.430111584758));
#27130=CARTESIAN_POINT('Ctrl Pts',(208.023559698486,94.2397376070391,339.49385073704));
#27131=CARTESIAN_POINT('Ctrl Pts',(207.849483299494,94.1772376070391,341.557589889321));
#27132=CARTESIAN_POINT('Ctrl Pts',(206.267108748143,94.1147376070391,342.893783236327));
#27133=CARTESIAN_POINT('Ctrl Pts',(204.684734196793,94.0522376070391,344.229976583334));
#27134=CARTESIAN_POINT('Ctrl Pts',(202.620995044512,93.9897376070391,344.055900184342));
#27135=CARTESIAN_POINT('Ctrl Pts',(200.55725589223,93.9272376070391,343.881823785349));
#27136=CARTESIAN_POINT('Ctrl Pts',(199.221062545224,93.8647376070391,342.299449233999));
#27137=CARTESIAN_POINT('Ctrl Pts',(197.884869198218,93.8022376070391,340.717074682649));
#27138=CARTESIAN_POINT('Ctrl Pts',(198.05894559721,93.7397376070391,338.653335530367));
#27139=CARTESIAN_POINT('Ctrl Pts',(198.233021996202,93.6772376070391,336.589596378086));
#27140=CARTESIAN_POINT('Ctrl Pts',(199.815396547552,93.6147376070391,335.253403031079));
#27141=CARTESIAN_POINT('Ctrl Pts',(201.397771098903,93.5522376070391,333.917209684073));
#27142=CARTESIAN_POINT('Ctrl Pts',(203.461510251184,93.4897376070391,334.091286083065));
#27143=CARTESIAN_POINT('Ctrl Pts',(205.525249403466,93.4272376070391,334.265362482058));
#27144=CARTESIAN_POINT('Ctrl Pts',(206.861442750472,93.3647376070391,335.847737033408));
#27145=CARTESIAN_POINT('Ctrl Pts',(208.197636097478,93.3022376070391,337.430111584758));
#27146=CARTESIAN_POINT('Ctrl Pts',(208.023559698486,93.2397376070391,339.49385073704));
#27147=CARTESIAN_POINT('Ctrl Pts',(207.849483299494,93.1772376070391,341.557589889321));
#27148=CARTESIAN_POINT('Ctrl Pts',(206.267108748143,93.1147376070391,342.893783236327));
#27149=CARTESIAN_POINT('Ctrl Pts',(204.684734196793,93.0522376070391,344.229976583334));
#27150=CARTESIAN_POINT('Ctrl Pts',(202.620995044512,92.9897376070391,344.055900184342));
#27151=CARTESIAN_POINT('Ctrl Pts',(200.55725589223,92.9272376070391,343.881823785349));
#27152=CARTESIAN_POINT('Ctrl Pts',(199.221062545224,92.8647376070391,342.299449233999));
#27153=CARTESIAN_POINT('Ctrl Pts',(197.884869198218,92.8022376070391,340.717074682649));
#27154=CARTESIAN_POINT('Ctrl Pts',(198.05894559721,92.7397376070391,338.653335530367));
#27155=CARTESIAN_POINT('Ctrl Pts',(198.233021996202,92.6772376070391,336.589596378086));
#27156=CARTESIAN_POINT('Ctrl Pts',(199.815396547552,92.6147376070391,335.253403031079));
#27157=CARTESIAN_POINT('Ctrl Pts',(201.397771098903,92.5522376070391,333.917209684073));
#27158=CARTESIAN_POINT('Ctrl Pts',(203.461510251184,92.4897376070391,334.091286083065));
#27159=CARTESIAN_POINT('Ctrl Pts',(205.525249403466,92.4272376070391,334.265362482058));
#27160=CARTESIAN_POINT('Ctrl Pts',(206.861442750472,92.3647376070391,335.847737033408));
#27161=CARTESIAN_POINT('Ctrl Pts',(208.197636097478,92.3022376070391,337.430111584758));
#27162=CARTESIAN_POINT('Ctrl Pts',(208.023559698486,92.2397376070391,339.49385073704));
#27163=CARTESIAN_POINT('Ctrl Pts',(207.849483299494,92.1772376070391,341.557589889321));
#27164=CARTESIAN_POINT('Ctrl Pts',(206.267108748143,92.1147376070391,342.893783236327));
#27165=CARTESIAN_POINT('Ctrl Pts',(204.684734196793,92.0522376070391,344.229976583334));
#27166=CARTESIAN_POINT('Ctrl Pts',(202.620995044512,91.9897376070391,344.055900184342));
#27167=CARTESIAN_POINT('Ctrl Pts',(200.55725589223,91.9272376070391,343.881823785349));
#27168=CARTESIAN_POINT('Ctrl Pts',(199.221062545224,91.8647376070391,342.299449233999));
#27169=CARTESIAN_POINT('Ctrl Pts',(197.884869198218,91.8022376070391,340.717074682649));
#27170=CARTESIAN_POINT('Ctrl Pts',(198.05894559721,91.7397376070391,338.653335530367));
#27171=CARTESIAN_POINT('Ctrl Pts',(198.233021996202,91.6772376070391,336.589596378086));
#27172=CARTESIAN_POINT('Ctrl Pts',(199.815396547552,91.6147376070391,335.253403031079));
#27173=CARTESIAN_POINT('Ctrl Pts',(201.397771098903,91.5522376070391,333.917209684073));
#27174=CARTESIAN_POINT('Ctrl Pts',(203.461510251184,91.4897376070391,334.091286083065));
#27175=CARTESIAN_POINT('Ctrl Pts',(205.525249403466,91.4272376070391,334.265362482058));
#27176=CARTESIAN_POINT('Ctrl Pts',(206.861442750472,91.3647376070391,335.847737033408));
#27177=CARTESIAN_POINT('Ctrl Pts',(208.197636097478,91.3022376070391,337.430111584758));
#27178=CARTESIAN_POINT('Ctrl Pts',(208.023559698486,91.2397376070391,339.49385073704));
#27179=CARTESIAN_POINT('Ctrl Pts',(207.849483299494,91.1772376070391,341.557589889321));
#27180=CARTESIAN_POINT('Ctrl Pts',(206.267108748143,91.1147376070391,342.893783236327));
#27181=CARTESIAN_POINT('Ctrl Pts',(204.684734196793,91.0522376070391,344.229976583334));
#27182=CARTESIAN_POINT('Ctrl Pts',(202.620995044512,90.9897376070391,344.055900184342));
#27183=CARTESIAN_POINT('Ctrl Pts',(200.55725589223,90.9272376070391,343.881823785349));
#27184=CARTESIAN_POINT('Ctrl Pts',(199.221062545224,90.8647376070391,342.299449233999));
#27185=CARTESIAN_POINT('Ctrl Pts',(197.884869198218,90.8022376070391,340.717074682649));
#27186=CARTESIAN_POINT('Ctrl Pts',(198.05894559721,90.7397376070391,338.653335530367));
#27187=CARTESIAN_POINT('Ctrl Pts',(198.233021996202,90.6772376070391,336.589596378086));
#27188=CARTESIAN_POINT('Ctrl Pts',(199.815396547552,90.6147376070391,335.253403031079));
#27189=CARTESIAN_POINT('Ctrl Pts',(201.397771098903,90.5522376070391,333.917209684073));
#27190=CARTESIAN_POINT('Ctrl Pts',(203.461510251184,90.4897376070391,334.091286083065));
#27191=CARTESIAN_POINT('Ctrl Pts',(205.525249403466,90.4272376070391,334.265362482058));
#27192=CARTESIAN_POINT('Ctrl Pts',(206.861442750472,90.3647376070391,335.847737033408));
#27193=CARTESIAN_POINT('Ctrl Pts',(208.197636097478,90.3022376070391,337.430111584758));
#27194=CARTESIAN_POINT('Ctrl Pts',(208.023559698486,90.2397376070391,339.49385073704));
#27195=CARTESIAN_POINT('Ctrl Pts',(207.849483299494,90.1772376070391,341.557589889321));
#27196=CARTESIAN_POINT('Ctrl Pts',(206.267108748143,90.1147376070391,342.893783236327));
#27197=CARTESIAN_POINT('Ctrl Pts',(204.684734196793,90.0522376070391,344.229976583334));
#27198=CARTESIAN_POINT('Ctrl Pts',(202.620995044512,89.9897376070391,344.055900184342));
#27199=CARTESIAN_POINT('Ctrl Pts',(200.55725589223,89.9272376070391,343.881823785349));
#27200=CARTESIAN_POINT('Ctrl Pts',(199.221062545224,89.8647376070391,342.299449233999));
#27201=CARTESIAN_POINT('Ctrl Pts',(197.884869198218,89.8022376070391,340.717074682649));
#27202=CARTESIAN_POINT('Ctrl Pts',(198.05894559721,89.7397376070391,338.653335530367));
#27203=CARTESIAN_POINT('Ctrl Pts',(197.519595040153,99.4272376084047,338.607841310488));
#27204=CARTESIAN_POINT('Ctrl Pts',(197.712515762029,99.3647376084047,336.320695842601));
#27205=CARTESIAN_POINT('Ctrl Pts',(199.466187382602,99.3022376084047,334.839855323367));
#27206=CARTESIAN_POINT('Ctrl Pts',(201.219859003176,99.2397376084047,333.359014804133));
#27207=CARTESIAN_POINT('Ctrl Pts',(203.507004471063,99.1772376084047,333.551935526009));
#27208=CARTESIAN_POINT('Ctrl Pts',(205.794149938951,99.1147376084047,333.744856247885));
#27209=CARTESIAN_POINT('Ctrl Pts',(207.274990458185,99.0522376084047,335.498527868458));
#27210=CARTESIAN_POINT('Ctrl Pts',(208.755830977418,98.9897376084047,337.252199489031));
#27211=CARTESIAN_POINT('Ctrl Pts',(208.562910255543,98.9272376084047,339.539344956919));
#27212=CARTESIAN_POINT('Ctrl Pts',(208.369989533667,98.8647376084047,341.826490424806));
#27213=CARTESIAN_POINT('Ctrl Pts',(206.616317913094,98.8022376084047,343.30733094404));
#27214=CARTESIAN_POINT('Ctrl Pts',(204.86264629252,98.7397376084047,344.788171463274));
#27215=CARTESIAN_POINT('Ctrl Pts',(202.575500824633,98.6772376084047,344.595250741398));
#27216=CARTESIAN_POINT('Ctrl Pts',(200.288355356745,98.6147376084047,344.402330019522));
#27217=CARTESIAN_POINT('Ctrl Pts',(198.807514837511,98.5522376084047,342.648658398949));
#27218=CARTESIAN_POINT('Ctrl Pts',(197.326674318278,98.4897376084047,340.894986778376));
#27219=CARTESIAN_POINT('Ctrl Pts',(197.519595040153,98.4272376084047,338.607841310488));
#27220=CARTESIAN_POINT('Ctrl Pts',(197.712515762029,98.3647376084047,336.320695842601));
#27221=CARTESIAN_POINT('Ctrl Pts',(199.466187382602,98.3022376084047,334.839855323367));
#27222=CARTESIAN_POINT('Ctrl Pts',(201.219859003176,98.2397376084047,333.359014804133));
#27223=CARTESIAN_POINT('Ctrl Pts',(203.507004471063,98.1772376084047,333.551935526009));
#27224=CARTESIAN_POINT('Ctrl Pts',(205.794149938951,98.1147376084047,333.744856247885));
#27225=CARTESIAN_POINT('Ctrl Pts',(207.274990458185,98.0522376084047,335.498527868458));
#27226=CARTESIAN_POINT('Ctrl Pts',(208.755830977418,97.9897376084047,337.252199489031));
#27227=CARTESIAN_POINT('Ctrl Pts',(208.562910255543,97.9272376084047,339.539344956919));
#27228=CARTESIAN_POINT('Ctrl Pts',(208.369989533667,97.8647376084047,341.826490424806));
#27229=CARTESIAN_POINT('Ctrl Pts',(206.616317913094,97.8022376084047,343.30733094404));
#27230=CARTESIAN_POINT('Ctrl Pts',(204.86264629252,97.7397376084047,344.788171463274));
#27231=CARTESIAN_POINT('Ctrl Pts',(202.575500824633,97.6772376084047,344.595250741398));
#27232=CARTESIAN_POINT('Ctrl Pts',(200.288355356745,97.6147376084047,344.402330019522));
#27233=CARTESIAN_POINT('Ctrl Pts',(198.807514837511,97.5522376084047,342.648658398949));
#27234=CARTESIAN_POINT('Ctrl Pts',(197.326674318278,97.4897376084047,340.894986778376));
#27235=CARTESIAN_POINT('Ctrl Pts',(197.519595040153,97.4272376084047,338.607841310488));
#27236=CARTESIAN_POINT('Ctrl Pts',(197.712515762029,97.3647376084047,336.320695842601));
#27237=CARTESIAN_POINT('Ctrl Pts',(199.466187382602,97.3022376084047,334.839855323367));
#27238=CARTESIAN_POINT('Ctrl Pts',(201.219859003176,97.2397376084047,333.359014804133));
#27239=CARTESIAN_POINT('Ctrl Pts',(203.507004471063,97.1772376084047,333.551935526009));
#27240=CARTESIAN_POINT('Ctrl Pts',(205.794149938951,97.1147376084047,333.744856247885));
#27241=CARTESIAN_POINT('Ctrl Pts',(207.274990458185,97.0522376084047,335.498527868458));
#27242=CARTESIAN_POINT('Ctrl Pts',(208.755830977418,96.9897376084047,337.252199489031));
#27243=CARTESIAN_POINT('Ctrl Pts',(208.562910255543,96.9272376084047,339.539344956919));
#27244=CARTESIAN_POINT('Ctrl Pts',(208.369989533667,96.8647376084047,341.826490424806));
#27245=CARTESIAN_POINT('Ctrl Pts',(206.616317913094,96.8022376084046,343.30733094404));
#27246=CARTESIAN_POINT('Ctrl Pts',(204.86264629252,96.7397376084047,344.788171463274));
#27247=CARTESIAN_POINT('Ctrl Pts',(202.575500824633,96.6772376084047,344.595250741398));
#27248=CARTESIAN_POINT('Ctrl Pts',(200.288355356745,96.6147376084047,344.402330019522));
#27249=CARTESIAN_POINT('Ctrl Pts',(198.807514837511,96.5522376084046,342.648658398949));
#27250=CARTESIAN_POINT('Ctrl Pts',(197.326674318278,96.4897376084047,340.894986778376));
#27251=CARTESIAN_POINT('Ctrl Pts',(197.519595040153,96.4272376084047,338.607841310488));
#27252=CARTESIAN_POINT('Ctrl Pts',(197.712515762029,96.3647376084047,336.320695842601));
#27253=CARTESIAN_POINT('Ctrl Pts',(199.466187382602,96.3022376084047,334.839855323367));
#27254=CARTESIAN_POINT('Ctrl Pts',(201.219859003176,96.2397376084047,333.359014804133));
#27255=CARTESIAN_POINT('Ctrl Pts',(203.507004471063,96.1772376084047,333.551935526009));
#27256=CARTESIAN_POINT('Ctrl Pts',(205.794149938951,96.1147376084047,333.744856247885));
#27257=CARTESIAN_POINT('Ctrl Pts',(207.274990458185,96.0522376084047,335.498527868458));
#27258=CARTESIAN_POINT('Ctrl Pts',(208.755830977418,95.9897376084047,337.252199489031));
#27259=CARTESIAN_POINT('Ctrl Pts',(208.562910255543,95.9272376084047,339.539344956919));
#27260=CARTESIAN_POINT('Ctrl Pts',(208.369989533667,95.8647376084047,341.826490424806));
#27261=CARTESIAN_POINT('Ctrl Pts',(206.616317913094,95.8022376084047,343.30733094404));
#27262=CARTESIAN_POINT('Ctrl Pts',(204.86264629252,95.7397376084047,344.788171463274));
#27263=CARTESIAN_POINT('Ctrl Pts',(202.575500824633,95.6772376084046,344.595250741398));
#27264=CARTESIAN_POINT('Ctrl Pts',(200.288355356745,95.6147376084047,344.402330019522));
#27265=CARTESIAN_POINT('Ctrl Pts',(198.807514837511,95.5522376084046,342.648658398949));
#27266=CARTESIAN_POINT('Ctrl Pts',(197.326674318278,95.4897376084047,340.894986778376));
#27267=CARTESIAN_POINT('Ctrl Pts',(197.519595040153,95.4272376084047,338.607841310488));
#27268=CARTESIAN_POINT('Ctrl Pts',(197.712515762029,95.3647376084047,336.320695842601));
#27269=CARTESIAN_POINT('Ctrl Pts',(199.466187382602,95.3022376084047,334.839855323367));
#27270=CARTESIAN_POINT('Ctrl Pts',(201.219859003176,95.2397376084047,333.359014804133));
#27271=CARTESIAN_POINT('Ctrl Pts',(203.507004471063,95.1772376084047,333.551935526009));
#27272=CARTESIAN_POINT('Ctrl Pts',(205.794149938951,95.1147376084047,333.744856247885));
#27273=CARTESIAN_POINT('Ctrl Pts',(207.274990458185,95.0522376084046,335.498527868458));
#27274=CARTESIAN_POINT('Ctrl Pts',(208.755830977418,94.9897376084047,337.252199489031));
#27275=CARTESIAN_POINT('Ctrl Pts',(208.562910255543,94.9272376084047,339.539344956919));
#27276=CARTESIAN_POINT('Ctrl Pts',(208.369989533667,94.8647376084047,341.826490424806));
#27277=CARTESIAN_POINT('Ctrl Pts',(206.616317913094,94.8022376084047,343.30733094404));
#27278=CARTESIAN_POINT('Ctrl Pts',(204.86264629252,94.7397376084047,344.788171463274));
#27279=CARTESIAN_POINT('Ctrl Pts',(202.575500824633,94.6772376084047,344.595250741398));
#27280=CARTESIAN_POINT('Ctrl Pts',(200.288355356745,94.6147376084047,344.402330019522));
#27281=CARTESIAN_POINT('Ctrl Pts',(198.807514837511,94.5522376084047,342.648658398949));
#27282=CARTESIAN_POINT('Ctrl Pts',(197.326674318278,94.4897376084047,340.894986778376));
#27283=CARTESIAN_POINT('Ctrl Pts',(197.519595040153,94.4272376084047,338.607841310488));
#27284=CARTESIAN_POINT('Ctrl Pts',(197.712515762029,94.3647376084047,336.320695842601));
#27285=CARTESIAN_POINT('Ctrl Pts',(199.466187382602,94.3022376084047,334.839855323367));
#27286=CARTESIAN_POINT('Ctrl Pts',(201.219859003176,94.2397376084047,333.359014804133));
#27287=CARTESIAN_POINT('Ctrl Pts',(203.507004471063,94.1772376084047,333.551935526009));
#27288=CARTESIAN_POINT('Ctrl Pts',(205.794149938951,94.1147376084047,333.744856247885));
#27289=CARTESIAN_POINT('Ctrl Pts',(207.274990458185,94.0522376084047,335.498527868458));
#27290=CARTESIAN_POINT('Ctrl Pts',(208.755830977418,93.9897376084047,337.252199489031));
#27291=CARTESIAN_POINT('Ctrl Pts',(208.562910255543,93.9272376084047,339.539344956919));
#27292=CARTESIAN_POINT('Ctrl Pts',(208.369989533667,93.8647376084047,341.826490424806));
#27293=CARTESIAN_POINT('Ctrl Pts',(206.616317913094,93.8022376084047,343.30733094404));
#27294=CARTESIAN_POINT('Ctrl Pts',(204.86264629252,93.7397376084047,344.788171463274));
#27295=CARTESIAN_POINT('Ctrl Pts',(202.575500824633,93.6772376084047,344.595250741398));
#27296=CARTESIAN_POINT('Ctrl Pts',(200.288355356745,93.6147376084047,344.402330019522));
#27297=CARTESIAN_POINT('Ctrl Pts',(198.807514837511,93.5522376084047,342.648658398949));
#27298=CARTESIAN_POINT('Ctrl Pts',(197.326674318278,93.4897376084047,340.894986778376));
#27299=CARTESIAN_POINT('Ctrl Pts',(197.519595040153,93.4272376084047,338.607841310488));
#27300=CARTESIAN_POINT('Ctrl Pts',(197.712515762029,93.3647376084047,336.320695842601));
#27301=CARTESIAN_POINT('Ctrl Pts',(199.466187382602,93.3022376084047,334.839855323367));
#27302=CARTESIAN_POINT('Ctrl Pts',(201.219859003176,93.2397376084047,333.359014804133));
#27303=CARTESIAN_POINT('Ctrl Pts',(203.507004471063,93.1772376084047,333.551935526009));
#27304=CARTESIAN_POINT('Ctrl Pts',(205.794149938951,93.1147376084047,333.744856247885));
#27305=CARTESIAN_POINT('Ctrl Pts',(207.274990458185,93.0522376084047,335.498527868458));
#27306=CARTESIAN_POINT('Ctrl Pts',(208.755830977418,92.9897376084047,337.252199489031));
#27307=CARTESIAN_POINT('Ctrl Pts',(208.562910255543,92.9272376084047,339.539344956919));
#27308=CARTESIAN_POINT('Ctrl Pts',(208.369989533667,92.8647376084047,341.826490424806));
#27309=CARTESIAN_POINT('Ctrl Pts',(206.616317913094,92.8022376084047,343.30733094404));
#27310=CARTESIAN_POINT('Ctrl Pts',(204.86264629252,92.7397376084047,344.788171463274));
#27311=CARTESIAN_POINT('Ctrl Pts',(202.575500824633,92.6772376084047,344.595250741398));
#27312=CARTESIAN_POINT('Ctrl Pts',(200.288355356745,92.6147376084047,344.402330019522));
#27313=CARTESIAN_POINT('Ctrl Pts',(198.807514837511,92.5522376084047,342.648658398949));
#27314=CARTESIAN_POINT('Ctrl Pts',(197.326674318278,92.4897376084047,340.894986778376));
#27315=CARTESIAN_POINT('Ctrl Pts',(197.519595040153,92.4272376084047,338.607841310488));
#27316=CARTESIAN_POINT('Ctrl Pts',(197.712515762029,92.3647376084047,336.320695842601));
#27317=CARTESIAN_POINT('Ctrl Pts',(199.466187382602,92.3022376084047,334.839855323367));
#27318=CARTESIAN_POINT('Ctrl Pts',(201.219859003176,92.2397376084047,333.359014804133));
#27319=CARTESIAN_POINT('Ctrl Pts',(203.507004471063,92.1772376084047,333.551935526009));
#27320=CARTESIAN_POINT('Ctrl Pts',(205.794149938951,92.1147376084047,333.744856247885));
#27321=CARTESIAN_POINT('Ctrl Pts',(207.274990458185,92.0522376084047,335.498527868458));
#27322=CARTESIAN_POINT('Ctrl Pts',(208.755830977418,91.9897376084047,337.252199489031));
#27323=CARTESIAN_POINT('Ctrl Pts',(208.562910255543,91.9272376084047,339.539344956919));
#27324=CARTESIAN_POINT('Ctrl Pts',(208.369989533667,91.8647376084047,341.826490424806));
#27325=CARTESIAN_POINT('Ctrl Pts',(206.616317913094,91.8022376084047,343.30733094404));
#27326=CARTESIAN_POINT('Ctrl Pts',(204.86264629252,91.7397376084047,344.788171463274));
#27327=CARTESIAN_POINT('Ctrl Pts',(202.575500824633,91.6772376084047,344.595250741398));
#27328=CARTESIAN_POINT('Ctrl Pts',(200.288355356745,91.6147376084047,344.402330019522));
#27329=CARTESIAN_POINT('Ctrl Pts',(198.807514837511,91.5522376084047,342.648658398949));
#27330=CARTESIAN_POINT('Ctrl Pts',(197.326674318278,91.4897376084047,340.894986778376));
#27331=CARTESIAN_POINT('Ctrl Pts',(197.519595040153,91.4272376084047,338.607841310488));
#27332=CARTESIAN_POINT('Ctrl Pts',(197.712515762029,91.3647376084047,336.320695842601));
#27333=CARTESIAN_POINT('Ctrl Pts',(199.466187382602,91.3022376084047,334.839855323367));
#27334=CARTESIAN_POINT('Ctrl Pts',(201.219859003176,91.2397376084047,333.359014804133));
#27335=CARTESIAN_POINT('Ctrl Pts',(203.507004471063,91.1772376084047,333.551935526009));
#27336=CARTESIAN_POINT('Ctrl Pts',(205.794149938951,91.1147376084047,333.744856247885));
#27337=CARTESIAN_POINT('Ctrl Pts',(207.274990458185,91.0522376084047,335.498527868458));
#27338=CARTESIAN_POINT('Ctrl Pts',(208.755830977418,90.9897376084047,337.252199489031));
#27339=CARTESIAN_POINT('Ctrl Pts',(208.562910255543,90.9272376084047,339.539344956919));
#27340=CARTESIAN_POINT('Ctrl Pts',(208.369989533667,90.8647376084047,341.826490424806));
#27341=CARTESIAN_POINT('Ctrl Pts',(206.616317913094,90.8022376084047,343.30733094404));
#27342=CARTESIAN_POINT('Ctrl Pts',(204.86264629252,90.7397376084047,344.788171463274));
#27343=CARTESIAN_POINT('Ctrl Pts',(202.575500824633,90.6772376084047,344.595250741398));
#27344=CARTESIAN_POINT('Ctrl Pts',(200.288355356745,90.6147376084047,344.402330019522));
#27345=CARTESIAN_POINT('Ctrl Pts',(198.807514837511,90.5522376084047,342.648658398949));
#27346=CARTESIAN_POINT('Ctrl Pts',(197.326674318278,90.4897376084047,340.894986778376));
#27347=CARTESIAN_POINT('Ctrl Pts',(197.519595040153,90.4272376084047,338.607841310488));
#27348=CARTESIAN_POINT('Ctrl Pts',(197.712515762029,90.3647376084047,336.320695842601));
#27349=CARTESIAN_POINT('Ctrl Pts',(199.466187382602,90.3022376084047,334.839855323367));
#27350=CARTESIAN_POINT('Ctrl Pts',(201.219859003176,90.2397376084047,333.359014804133));
#27351=CARTESIAN_POINT('Ctrl Pts',(203.507004471063,90.1772376084047,333.551935526009));
#27352=CARTESIAN_POINT('Ctrl Pts',(205.794149938951,90.1147376084047,333.744856247885));
#27353=CARTESIAN_POINT('Ctrl Pts',(207.274990458185,90.0522376084047,335.498527868458));
#27354=CARTESIAN_POINT('Ctrl Pts',(208.755830977418,89.9897376084047,337.252199489031));
#27355=CARTESIAN_POINT('Ctrl Pts',(208.562910255543,89.9272376084047,339.539344956919));
#27356=CARTESIAN_POINT('Ctrl Pts',(208.369989533667,89.8647376084047,341.826490424806));
#27357=CARTESIAN_POINT('Ctrl Pts',(206.616317913094,89.8022376084047,343.30733094404));
#27358=CARTESIAN_POINT('Ctrl Pts',(204.86264629252,89.7397376084047,344.788171463274));
#27359=CARTESIAN_POINT('Ctrl Pts',(202.575500824633,89.6772376084047,344.595250741398));
#27360=CARTESIAN_POINT('Ctrl Pts',(200.288355356745,89.6147376084047,344.402330019522));
#27361=CARTESIAN_POINT('Ctrl Pts',(198.807514837511,89.5522376084047,342.648658398949));
#27362=CARTESIAN_POINT('Ctrl Pts',(197.326674318278,89.4897376084047,340.894986778376));
#27363=CARTESIAN_POINT('Ctrl Pts',(197.519595040153,89.4272376084047,338.607841310488));
#27364=CARTESIAN_POINT('Ctrl Pts',(197.519595040153,99.3022376084047,338.607841310488));
#27365=CARTESIAN_POINT('Ctrl Pts',(197.712515762029,99.2397376084047,336.320695842601));
#27366=CARTESIAN_POINT('Ctrl Pts',(199.466187382602,99.1772376084047,334.839855323367));
#27367=CARTESIAN_POINT('Ctrl Pts',(201.219859003176,99.1147376084047,333.359014804133));
#27368=CARTESIAN_POINT('Ctrl Pts',(203.507004471063,99.0522376084047,333.551935526009));
#27369=CARTESIAN_POINT('Ctrl Pts',(205.794149938951,98.9897376084047,333.744856247885));
#27370=CARTESIAN_POINT('Ctrl Pts',(207.274990458185,98.9272376084047,335.498527868458));
#27371=CARTESIAN_POINT('Ctrl Pts',(208.755830977418,98.8647376084047,337.252199489031));
#27372=CARTESIAN_POINT('Ctrl Pts',(208.562910255543,98.8022376084047,339.539344956919));
#27373=CARTESIAN_POINT('Ctrl Pts',(208.369989533667,98.7397376084047,341.826490424806));
#27374=CARTESIAN_POINT('Ctrl Pts',(206.616317913094,98.6772376084047,343.30733094404));
#27375=CARTESIAN_POINT('Ctrl Pts',(204.86264629252,98.6147376084047,344.788171463274));
#27376=CARTESIAN_POINT('Ctrl Pts',(202.575500824633,98.5522376084047,344.595250741398));
#27377=CARTESIAN_POINT('Ctrl Pts',(200.288355356745,98.4897376084047,344.402330019522));
#27378=CARTESIAN_POINT('Ctrl Pts',(198.807514837511,98.4272376084047,342.648658398949));
#27379=CARTESIAN_POINT('Ctrl Pts',(197.326674318278,98.3647376084047,340.894986778376));
#27380=CARTESIAN_POINT('Ctrl Pts',(197.519595040153,98.3022376084047,338.607841310488));
#27381=CARTESIAN_POINT('Ctrl Pts',(197.712515762029,98.2397376084047,336.320695842601));
#27382=CARTESIAN_POINT('Ctrl Pts',(199.466187382602,98.1772376084047,334.839855323367));
#27383=CARTESIAN_POINT('Ctrl Pts',(201.219859003176,98.1147376084047,333.359014804133));
#27384=CARTESIAN_POINT('Ctrl Pts',(203.507004471063,98.0522376084047,333.551935526009));
#27385=CARTESIAN_POINT('Ctrl Pts',(205.794149938951,97.9897376084047,333.744856247885));
#27386=CARTESIAN_POINT('Ctrl Pts',(207.274990458185,97.9272376084047,335.498527868458));
#27387=CARTESIAN_POINT('Ctrl Pts',(208.755830977418,97.8647376084047,337.252199489031));
#27388=CARTESIAN_POINT('Ctrl Pts',(208.562910255543,97.8022376084047,339.539344956919));
#27389=CARTESIAN_POINT('Ctrl Pts',(208.369989533667,97.7397376084047,341.826490424806));
#27390=CARTESIAN_POINT('Ctrl Pts',(206.616317913094,97.6772376084047,343.30733094404));
#27391=CARTESIAN_POINT('Ctrl Pts',(204.86264629252,97.6147376084047,344.788171463274));
#27392=CARTESIAN_POINT('Ctrl Pts',(202.575500824633,97.5522376084047,344.595250741398));
#27393=CARTESIAN_POINT('Ctrl Pts',(200.288355356745,97.4897376084047,344.402330019522));
#27394=CARTESIAN_POINT('Ctrl Pts',(198.807514837511,97.4272376084047,342.648658398949));
#27395=CARTESIAN_POINT('Ctrl Pts',(197.326674318278,97.3647376084047,340.894986778376));
#27396=CARTESIAN_POINT('Ctrl Pts',(197.519595040153,97.3022376084047,338.607841310488));
#27397=CARTESIAN_POINT('Ctrl Pts',(197.712515762029,97.2397376084047,336.320695842601));
#27398=CARTESIAN_POINT('Ctrl Pts',(199.466187382602,97.1772376084047,334.839855323367));
#27399=CARTESIAN_POINT('Ctrl Pts',(201.219859003176,97.1147376084047,333.359014804133));
#27400=CARTESIAN_POINT('Ctrl Pts',(203.507004471063,97.0522376084047,333.551935526009));
#27401=CARTESIAN_POINT('Ctrl Pts',(205.794149938951,96.9897376084047,333.744856247885));
#27402=CARTESIAN_POINT('Ctrl Pts',(207.274990458185,96.9272376084047,335.498527868458));
#27403=CARTESIAN_POINT('Ctrl Pts',(208.755830977418,96.8647376084047,337.252199489031));
#27404=CARTESIAN_POINT('Ctrl Pts',(208.562910255543,96.8022376084046,339.539344956919));
#27405=CARTESIAN_POINT('Ctrl Pts',(208.369989533667,96.7397376084047,341.826490424806));
#27406=CARTESIAN_POINT('Ctrl Pts',(206.616317913094,96.6772376084047,343.30733094404));
#27407=CARTESIAN_POINT('Ctrl Pts',(204.86264629252,96.6147376084047,344.788171463274));
#27408=CARTESIAN_POINT('Ctrl Pts',(202.575500824633,96.5522376084046,344.595250741398));
#27409=CARTESIAN_POINT('Ctrl Pts',(200.288355356745,96.4897376084047,344.402330019522));
#27410=CARTESIAN_POINT('Ctrl Pts',(198.807514837511,96.4272376084047,342.648658398949));
#27411=CARTESIAN_POINT('Ctrl Pts',(197.326674318278,96.3647376084047,340.894986778376));
#27412=CARTESIAN_POINT('Ctrl Pts',(197.519595040153,96.3022376084047,338.607841310488));
#27413=CARTESIAN_POINT('Ctrl Pts',(197.712515762029,96.2397376084047,336.320695842601));
#27414=CARTESIAN_POINT('Ctrl Pts',(199.466187382602,96.1772376084047,334.839855323367));
#27415=CARTESIAN_POINT('Ctrl Pts',(201.219859003176,96.1147376084047,333.359014804133));
#27416=CARTESIAN_POINT('Ctrl Pts',(203.507004471063,96.0522376084047,333.551935526009));
#27417=CARTESIAN_POINT('Ctrl Pts',(205.794149938951,95.9897376084047,333.744856247885));
#27418=CARTESIAN_POINT('Ctrl Pts',(207.274990458185,95.9272376084047,335.498527868458));
#27419=CARTESIAN_POINT('Ctrl Pts',(208.755830977418,95.8647376084047,337.252199489031));
#27420=CARTESIAN_POINT('Ctrl Pts',(208.562910255543,95.8022376084047,339.539344956919));
#27421=CARTESIAN_POINT('Ctrl Pts',(208.369989533667,95.7397376084047,341.826490424806));
#27422=CARTESIAN_POINT('Ctrl Pts',(206.616317913094,95.6772376084046,343.30733094404));
#27423=CARTESIAN_POINT('Ctrl Pts',(204.86264629252,95.6147376084047,344.788171463274));
#27424=CARTESIAN_POINT('Ctrl Pts',(202.575500824633,95.5522376084046,344.595250741398));
#27425=CARTESIAN_POINT('Ctrl Pts',(200.288355356745,95.4897376084047,344.402330019522));
#27426=CARTESIAN_POINT('Ctrl Pts',(198.807514837511,95.4272376084047,342.648658398949));
#27427=CARTESIAN_POINT('Ctrl Pts',(197.326674318278,95.3647376084047,340.894986778376));
#27428=CARTESIAN_POINT('Ctrl Pts',(197.519595040153,95.3022376084046,338.607841310488));
#27429=CARTESIAN_POINT('Ctrl Pts',(197.712515762029,95.2397376084047,336.320695842601));
#27430=CARTESIAN_POINT('Ctrl Pts',(199.466187382602,95.1772376084047,334.839855323367));
#27431=CARTESIAN_POINT('Ctrl Pts',(201.219859003176,95.1147376084047,333.359014804133));
#27432=CARTESIAN_POINT('Ctrl Pts',(203.507004471063,95.0522376084047,333.551935526009));
#27433=CARTESIAN_POINT('Ctrl Pts',(205.794149938951,94.9897376084047,333.744856247885));
#27434=CARTESIAN_POINT('Ctrl Pts',(207.274990458185,94.9272376084047,335.498527868458));
#27435=CARTESIAN_POINT('Ctrl Pts',(208.755830977418,94.8647376084047,337.252199489031));
#27436=CARTESIAN_POINT('Ctrl Pts',(208.562910255543,94.8022376084047,339.539344956919));
#27437=CARTESIAN_POINT('Ctrl Pts',(208.369989533667,94.7397376084047,341.826490424806));
#27438=CARTESIAN_POINT('Ctrl Pts',(206.616317913094,94.6772376084047,343.30733094404));
#27439=CARTESIAN_POINT('Ctrl Pts',(204.86264629252,94.6147376084047,344.788171463274));
#27440=CARTESIAN_POINT('Ctrl Pts',(202.575500824633,94.5522376084047,344.595250741398));
#27441=CARTESIAN_POINT('Ctrl Pts',(200.288355356745,94.4897376084047,344.402330019522));
#27442=CARTESIAN_POINT('Ctrl Pts',(198.807514837511,94.4272376084047,342.648658398949));
#27443=CARTESIAN_POINT('Ctrl Pts',(197.326674318278,94.3647376084047,340.894986778376));
#27444=CARTESIAN_POINT('Ctrl Pts',(197.519595040153,94.3022376084047,338.607841310488));
#27445=CARTESIAN_POINT('Ctrl Pts',(197.712515762029,94.2397376084047,336.320695842601));
#27446=CARTESIAN_POINT('Ctrl Pts',(199.466187382602,94.1772376084047,334.839855323367));
#27447=CARTESIAN_POINT('Ctrl Pts',(201.219859003176,94.1147376084047,333.359014804133));
#27448=CARTESIAN_POINT('Ctrl Pts',(203.507004471063,94.0522376084047,333.551935526009));
#27449=CARTESIAN_POINT('Ctrl Pts',(205.794149938951,93.9897376084047,333.744856247885));
#27450=CARTESIAN_POINT('Ctrl Pts',(207.274990458185,93.9272376084047,335.498527868458));
#27451=CARTESIAN_POINT('Ctrl Pts',(208.755830977418,93.8647376084047,337.252199489031));
#27452=CARTESIAN_POINT('Ctrl Pts',(208.562910255543,93.8022376084047,339.539344956919));
#27453=CARTESIAN_POINT('Ctrl Pts',(208.369989533667,93.7397376084047,341.826490424806));
#27454=CARTESIAN_POINT('Ctrl Pts',(206.616317913094,93.6772376084047,343.30733094404));
#27455=CARTESIAN_POINT('Ctrl Pts',(204.86264629252,93.6147376084047,344.788171463274));
#27456=CARTESIAN_POINT('Ctrl Pts',(202.575500824633,93.5522376084047,344.595250741398));
#27457=CARTESIAN_POINT('Ctrl Pts',(200.288355356745,93.4897376084047,344.402330019522));
#27458=CARTESIAN_POINT('Ctrl Pts',(198.807514837511,93.4272376084047,342.648658398949));
#27459=CARTESIAN_POINT('Ctrl Pts',(197.326674318278,93.3647376084047,340.894986778376));
#27460=CARTESIAN_POINT('Ctrl Pts',(197.519595040153,93.3022376084047,338.607841310488));
#27461=CARTESIAN_POINT('Ctrl Pts',(197.712515762029,93.2397376084047,336.320695842601));
#27462=CARTESIAN_POINT('Ctrl Pts',(199.466187382602,93.1772376084047,334.839855323367));
#27463=CARTESIAN_POINT('Ctrl Pts',(201.219859003176,93.1147376084047,333.359014804133));
#27464=CARTESIAN_POINT('Ctrl Pts',(203.507004471063,93.0522376084047,333.551935526009));
#27465=CARTESIAN_POINT('Ctrl Pts',(205.794149938951,92.9897376084047,333.744856247885));
#27466=CARTESIAN_POINT('Ctrl Pts',(207.274990458185,92.9272376084047,335.498527868458));
#27467=CARTESIAN_POINT('Ctrl Pts',(208.755830977418,92.8647376084047,337.252199489031));
#27468=CARTESIAN_POINT('Ctrl Pts',(208.562910255543,92.8022376084047,339.539344956919));
#27469=CARTESIAN_POINT('Ctrl Pts',(208.369989533667,92.7397376084047,341.826490424806));
#27470=CARTESIAN_POINT('Ctrl Pts',(206.616317913094,92.6772376084047,343.30733094404));
#27471=CARTESIAN_POINT('Ctrl Pts',(204.86264629252,92.6147376084047,344.788171463274));
#27472=CARTESIAN_POINT('Ctrl Pts',(202.575500824633,92.5522376084047,344.595250741398));
#27473=CARTESIAN_POINT('Ctrl Pts',(200.288355356745,92.4897376084047,344.402330019522));
#27474=CARTESIAN_POINT('Ctrl Pts',(198.807514837511,92.4272376084047,342.648658398949));
#27475=CARTESIAN_POINT('Ctrl Pts',(197.326674318278,92.3647376084047,340.894986778376));
#27476=CARTESIAN_POINT('Ctrl Pts',(197.519595040153,92.3022376084047,338.607841310488));
#27477=CARTESIAN_POINT('Ctrl Pts',(197.712515762029,92.2397376084047,336.320695842601));
#27478=CARTESIAN_POINT('Ctrl Pts',(199.466187382602,92.1772376084047,334.839855323367));
#27479=CARTESIAN_POINT('Ctrl Pts',(201.219859003176,92.1147376084047,333.359014804133));
#27480=CARTESIAN_POINT('Ctrl Pts',(203.507004471063,92.0522376084047,333.551935526009));
#27481=CARTESIAN_POINT('Ctrl Pts',(205.794149938951,91.9897376084047,333.744856247885));
#27482=CARTESIAN_POINT('Ctrl Pts',(207.274990458185,91.9272376084047,335.498527868458));
#27483=CARTESIAN_POINT('Ctrl Pts',(208.755830977418,91.8647376084047,337.252199489031));
#27484=CARTESIAN_POINT('Ctrl Pts',(208.562910255543,91.8022376084047,339.539344956919));
#27485=CARTESIAN_POINT('Ctrl Pts',(208.369989533667,91.7397376084047,341.826490424806));
#27486=CARTESIAN_POINT('Ctrl Pts',(206.616317913094,91.6772376084047,343.30733094404));
#27487=CARTESIAN_POINT('Ctrl Pts',(204.86264629252,91.6147376084047,344.788171463274));
#27488=CARTESIAN_POINT('Ctrl Pts',(202.575500824633,91.5522376084047,344.595250741398));
#27489=CARTESIAN_POINT('Ctrl Pts',(200.288355356745,91.4897376084047,344.402330019522));
#27490=CARTESIAN_POINT('Ctrl Pts',(198.807514837511,91.4272376084047,342.648658398949));
#27491=CARTESIAN_POINT('Ctrl Pts',(197.326674318278,91.3647376084047,340.894986778376));
#27492=CARTESIAN_POINT('Ctrl Pts',(197.519595040153,91.3022376084047,338.607841310488));
#27493=CARTESIAN_POINT('Ctrl Pts',(197.712515762029,91.2397376084047,336.320695842601));
#27494=CARTESIAN_POINT('Ctrl Pts',(199.466187382602,91.1772376084047,334.839855323367));
#27495=CARTESIAN_POINT('Ctrl Pts',(201.219859003176,91.1147376084047,333.359014804133));
#27496=CARTESIAN_POINT('Ctrl Pts',(203.507004471063,91.0522376084047,333.551935526009));
#27497=CARTESIAN_POINT('Ctrl Pts',(205.794149938951,90.9897376084047,333.744856247885));
#27498=CARTESIAN_POINT('Ctrl Pts',(207.274990458185,90.9272376084047,335.498527868458));
#27499=CARTESIAN_POINT('Ctrl Pts',(208.755830977418,90.8647376084047,337.252199489031));
#27500=CARTESIAN_POINT('Ctrl Pts',(208.562910255543,90.8022376084047,339.539344956919));
#27501=CARTESIAN_POINT('Ctrl Pts',(208.369989533667,90.7397376084047,341.826490424806));
#27502=CARTESIAN_POINT('Ctrl Pts',(206.616317913094,90.6772376084047,343.30733094404));
#27503=CARTESIAN_POINT('Ctrl Pts',(204.86264629252,90.6147376084047,344.788171463274));
#27504=CARTESIAN_POINT('Ctrl Pts',(202.575500824633,90.5522376084047,344.595250741398));
#27505=CARTESIAN_POINT('Ctrl Pts',(200.288355356745,90.4897376084047,344.402330019522));
#27506=CARTESIAN_POINT('Ctrl Pts',(198.807514837511,90.4272376084047,342.648658398949));
#27507=CARTESIAN_POINT('Ctrl Pts',(197.326674318278,90.3647376084047,340.894986778376));
#27508=CARTESIAN_POINT('Ctrl Pts',(197.519595040153,90.3022376084047,338.607841310488));
#27509=CARTESIAN_POINT('Ctrl Pts',(197.712515762029,90.2397376084047,336.320695842601));
#27510=CARTESIAN_POINT('Ctrl Pts',(199.466187382602,90.1772376084047,334.839855323367));
#27511=CARTESIAN_POINT('Ctrl Pts',(201.219859003176,90.1147376084047,333.359014804133));
#27512=CARTESIAN_POINT('Ctrl Pts',(203.507004471063,90.0522376084047,333.551935526009));
#27513=CARTESIAN_POINT('Ctrl Pts',(205.794149938951,89.9897376084047,333.744856247885));
#27514=CARTESIAN_POINT('Ctrl Pts',(207.274990458185,89.9272376084047,335.498527868458));
#27515=CARTESIAN_POINT('Ctrl Pts',(208.755830977418,89.8647376084047,337.252199489031));
#27516=CARTESIAN_POINT('Ctrl Pts',(208.562910255543,89.8022376084047,339.539344956919));
#27517=CARTESIAN_POINT('Ctrl Pts',(208.369989533667,89.7397376084047,341.826490424806));
#27518=CARTESIAN_POINT('Ctrl Pts',(206.616317913094,89.6772376084047,343.30733094404));
#27519=CARTESIAN_POINT('Ctrl Pts',(204.86264629252,89.6147376084047,344.788171463274));
#27520=CARTESIAN_POINT('Ctrl Pts',(202.575500824633,89.5522376084047,344.595250741398));
#27521=CARTESIAN_POINT('Ctrl Pts',(200.288355356745,89.4897376084047,344.402330019522));
#27522=CARTESIAN_POINT('Ctrl Pts',(198.807514837511,89.4272376084047,342.648658398949));
#27523=CARTESIAN_POINT('Ctrl Pts',(197.326674318278,89.3647376084047,340.894986778376));
#27524=CARTESIAN_POINT('Ctrl Pts',(197.519595040153,89.3022376084047,338.607841310488));
#27525=CARTESIAN_POINT('Ctrl Pts',(198.05894559721,98.9897376097703,338.653335530367));
#27526=CARTESIAN_POINT('Ctrl Pts',(198.233021996202,98.9272376097703,336.589596378086));
#27527=CARTESIAN_POINT('Ctrl Pts',(199.815396547552,98.8647376097703,335.253403031079));
#27528=CARTESIAN_POINT('Ctrl Pts',(201.397771098903,98.8022376097702,333.917209684073));
#27529=CARTESIAN_POINT('Ctrl Pts',(203.461510251184,98.7397376097702,334.091286083065));
#27530=CARTESIAN_POINT('Ctrl Pts',(205.525249403466,98.6772376097703,334.265362482058));
#27531=CARTESIAN_POINT('Ctrl Pts',(206.861442750472,98.6147376097703,335.847737033408));
#27532=CARTESIAN_POINT('Ctrl Pts',(208.197636097478,98.5522376097703,337.430111584758));
#27533=CARTESIAN_POINT('Ctrl Pts',(208.023559698486,98.4897376097702,339.49385073704));
#27534=CARTESIAN_POINT('Ctrl Pts',(207.849483299494,98.4272376097702,341.557589889321));
#27535=CARTESIAN_POINT('Ctrl Pts',(206.267108748143,98.3647376097703,342.893783236327));
#27536=CARTESIAN_POINT('Ctrl Pts',(204.684734196793,98.3022376097703,344.229976583334));
#27537=CARTESIAN_POINT('Ctrl Pts',(202.620995044512,98.2397376097703,344.055900184342));
#27538=CARTESIAN_POINT('Ctrl Pts',(200.55725589223,98.1772376097702,343.881823785349));
#27539=CARTESIAN_POINT('Ctrl Pts',(199.221062545224,98.1147376097702,342.299449233999));
#27540=CARTESIAN_POINT('Ctrl Pts',(197.884869198218,98.0522376097703,340.717074682649));
#27541=CARTESIAN_POINT('Ctrl Pts',(198.05894559721,97.9897376097703,338.653335530367));
#27542=CARTESIAN_POINT('Ctrl Pts',(198.233021996202,97.9272376097703,336.589596378086));
#27543=CARTESIAN_POINT('Ctrl Pts',(199.815396547552,97.8647376097702,335.253403031079));
#27544=CARTESIAN_POINT('Ctrl Pts',(201.397771098903,97.8022376097703,333.917209684073));
#27545=CARTESIAN_POINT('Ctrl Pts',(203.461510251184,97.7397376097703,334.091286083065));
#27546=CARTESIAN_POINT('Ctrl Pts',(205.525249403466,97.6772376097703,334.265362482058));
#27547=CARTESIAN_POINT('Ctrl Pts',(206.861442750472,97.6147376097703,335.847737033408));
#27548=CARTESIAN_POINT('Ctrl Pts',(208.197636097478,97.5522376097702,337.430111584758));
#27549=CARTESIAN_POINT('Ctrl Pts',(208.023559698486,97.4897376097702,339.49385073704));
#27550=CARTESIAN_POINT('Ctrl Pts',(207.849483299494,97.4272376097703,341.557589889321));
#27551=CARTESIAN_POINT('Ctrl Pts',(206.267108748143,97.3647376097703,342.893783236327));
#27552=CARTESIAN_POINT('Ctrl Pts',(204.684734196793,97.3022376097703,344.229976583334));
#27553=CARTESIAN_POINT('Ctrl Pts',(202.620995044512,97.2397376097702,344.055900184342));
#27554=CARTESIAN_POINT('Ctrl Pts',(200.55725589223,97.1772376097702,343.881823785349));
#27555=CARTESIAN_POINT('Ctrl Pts',(199.221062545224,97.1147376097703,342.299449233999));
#27556=CARTESIAN_POINT('Ctrl Pts',(197.884869198218,97.0522376097703,340.717074682649));
#27557=CARTESIAN_POINT('Ctrl Pts',(198.05894559721,96.9897376097703,338.653335530367));
#27558=CARTESIAN_POINT('Ctrl Pts',(198.233021996202,96.9272376097703,336.589596378086));
#27559=CARTESIAN_POINT('Ctrl Pts',(199.815396547552,96.8647376097702,335.253403031079));
#27560=CARTESIAN_POINT('Ctrl Pts',(201.397771098903,96.8022376097703,333.917209684073));
#27561=CARTESIAN_POINT('Ctrl Pts',(203.461510251184,96.7397376097703,334.091286083065));
#27562=CARTESIAN_POINT('Ctrl Pts',(205.525249403466,96.6772376097703,334.265362482058));
#27563=CARTESIAN_POINT('Ctrl Pts',(206.861442750472,96.6147376097702,335.847737033408));
#27564=CARTESIAN_POINT('Ctrl Pts',(208.197636097478,96.5522376097702,337.430111584758));
#27565=CARTESIAN_POINT('Ctrl Pts',(208.023559698486,96.4897376097703,339.49385073704));
#27566=CARTESIAN_POINT('Ctrl Pts',(207.849483299494,96.4272376097703,341.557589889321));
#27567=CARTESIAN_POINT('Ctrl Pts',(206.267108748143,96.3647376097703,342.893783236327));
#27568=CARTESIAN_POINT('Ctrl Pts',(204.684734196793,96.3022376097702,344.229976583334));
#27569=CARTESIAN_POINT('Ctrl Pts',(202.620995044512,96.2397376097702,344.055900184342));
#27570=CARTESIAN_POINT('Ctrl Pts',(200.55725589223,96.1772376097703,343.881823785349));
#27571=CARTESIAN_POINT('Ctrl Pts',(199.221062545224,96.1147376097703,342.299449233999));
#27572=CARTESIAN_POINT('Ctrl Pts',(197.884869198218,96.0522376097703,340.717074682649));
#27573=CARTESIAN_POINT('Ctrl Pts',(198.05894559721,95.9897376097702,338.653335530367));
#27574=CARTESIAN_POINT('Ctrl Pts',(198.233021996202,95.9272376097703,336.589596378086));
#27575=CARTESIAN_POINT('Ctrl Pts',(199.815396547552,95.8647376097703,335.253403031079));
#27576=CARTESIAN_POINT('Ctrl Pts',(201.397771098903,95.8022376097703,333.917209684073));
#27577=CARTESIAN_POINT('Ctrl Pts',(203.461510251184,95.7397376097702,334.091286083065));
#27578=CARTESIAN_POINT('Ctrl Pts',(205.525249403466,95.6772376097702,334.265362482058));
#27579=CARTESIAN_POINT('Ctrl Pts',(206.861442750472,95.6147376097702,335.847737033408));
#27580=CARTESIAN_POINT('Ctrl Pts',(208.197636097478,95.5522376097703,337.430111584758));
#27581=CARTESIAN_POINT('Ctrl Pts',(208.023559698486,95.4897376097703,339.49385073704));
#27582=CARTESIAN_POINT('Ctrl Pts',(207.849483299494,95.4272376097702,341.557589889321));
#27583=CARTESIAN_POINT('Ctrl Pts',(206.267108748143,95.3647376097702,342.893783236327));
#27584=CARTESIAN_POINT('Ctrl Pts',(204.684734196793,95.3022376097702,344.229976583334));
#27585=CARTESIAN_POINT('Ctrl Pts',(202.620995044512,95.2397376097703,344.055900184342));
#27586=CARTESIAN_POINT('Ctrl Pts',(200.55725589223,95.1772376097703,343.881823785349));
#27587=CARTESIAN_POINT('Ctrl Pts',(199.221062545224,95.1147376097702,342.299449233999));
#27588=CARTESIAN_POINT('Ctrl Pts',(197.884869198218,95.0522376097702,340.717074682649));
#27589=CARTESIAN_POINT('Ctrl Pts',(198.05894559721,94.9897376097702,338.653335530367));
#27590=CARTESIAN_POINT('Ctrl Pts',(198.233021996202,94.9272376097703,336.589596378086));
#27591=CARTESIAN_POINT('Ctrl Pts',(199.815396547552,94.8647376097703,335.253403031079));
#27592=CARTESIAN_POINT('Ctrl Pts',(201.397771098903,94.8022376097703,333.917209684073));
#27593=CARTESIAN_POINT('Ctrl Pts',(203.461510251184,94.7397376097702,334.091286083065));
#27594=CARTESIAN_POINT('Ctrl Pts',(205.525249403466,94.6772376097703,334.265362482058));
#27595=CARTESIAN_POINT('Ctrl Pts',(206.861442750472,94.6147376097703,335.847737033408));
#27596=CARTESIAN_POINT('Ctrl Pts',(208.197636097478,94.5522376097703,337.430111584758));
#27597=CARTESIAN_POINT('Ctrl Pts',(208.023559698486,94.4897376097702,339.49385073704));
#27598=CARTESIAN_POINT('Ctrl Pts',(207.849483299494,94.4272376097702,341.557589889321));
#27599=CARTESIAN_POINT('Ctrl Pts',(206.267108748143,94.3647376097702,342.893783236327));
#27600=CARTESIAN_POINT('Ctrl Pts',(204.684734196793,94.3022376097703,344.229976583334));
#27601=CARTESIAN_POINT('Ctrl Pts',(202.620995044512,94.2397376097703,344.055900184342));
#27602=CARTESIAN_POINT('Ctrl Pts',(200.55725589223,94.1772376097702,343.881823785349));
#27603=CARTESIAN_POINT('Ctrl Pts',(199.221062545224,94.1147376097702,342.299449233999));
#27604=CARTESIAN_POINT('Ctrl Pts',(197.884869198218,94.0522376097702,340.717074682649));
#27605=CARTESIAN_POINT('Ctrl Pts',(198.05894559721,93.9897376097703,338.653335530367));
#27606=CARTESIAN_POINT('Ctrl Pts',(198.233021996202,93.9272376097703,336.589596378086));
#27607=CARTESIAN_POINT('Ctrl Pts',(199.815396547552,93.8647376097702,335.253403031079));
#27608=CARTESIAN_POINT('Ctrl Pts',(201.397771098903,93.8022376097703,333.917209684073));
#27609=CARTESIAN_POINT('Ctrl Pts',(203.461510251184,93.7397376097702,334.091286083065));
#27610=CARTESIAN_POINT('Ctrl Pts',(205.525249403466,93.6772376097703,334.265362482058));
#27611=CARTESIAN_POINT('Ctrl Pts',(206.861442750472,93.6147376097702,335.847737033408));
#27612=CARTESIAN_POINT('Ctrl Pts',(208.197636097478,93.5522376097703,337.430111584758));
#27613=CARTESIAN_POINT('Ctrl Pts',(208.023559698486,93.4897376097702,339.49385073704));
#27614=CARTESIAN_POINT('Ctrl Pts',(207.849483299494,93.4272376097703,341.557589889321));
#27615=CARTESIAN_POINT('Ctrl Pts',(206.267108748143,93.3647376097702,342.893783236327));
#27616=CARTESIAN_POINT('Ctrl Pts',(204.684734196793,93.3022376097703,344.229976583334));
#27617=CARTESIAN_POINT('Ctrl Pts',(202.620995044512,93.2397376097702,344.055900184342));
#27618=CARTESIAN_POINT('Ctrl Pts',(200.55725589223,93.1772376097702,343.881823785349));
#27619=CARTESIAN_POINT('Ctrl Pts',(199.221062545224,93.1147376097702,342.299449233999));
#27620=CARTESIAN_POINT('Ctrl Pts',(197.884869198218,93.0522376097703,340.717074682649));
#27621=CARTESIAN_POINT('Ctrl Pts',(198.05894559721,92.9897376097703,338.653335530367));
#27622=CARTESIAN_POINT('Ctrl Pts',(198.233021996202,92.9272376097703,336.589596378086));
#27623=CARTESIAN_POINT('Ctrl Pts',(199.815396547552,92.8647376097702,335.253403031079));
#27624=CARTESIAN_POINT('Ctrl Pts',(201.397771098903,92.8022376097703,333.917209684073));
#27625=CARTESIAN_POINT('Ctrl Pts',(203.461510251184,92.7397376097703,334.091286083065));
#27626=CARTESIAN_POINT('Ctrl Pts',(205.525249403466,92.6772376097703,334.265362482058));
#27627=CARTESIAN_POINT('Ctrl Pts',(206.861442750472,92.6147376097702,335.847737033408));
#27628=CARTESIAN_POINT('Ctrl Pts',(208.197636097478,92.5522376097702,337.430111584758));
#27629=CARTESIAN_POINT('Ctrl Pts',(208.023559698486,92.4897376097702,339.49385073704));
#27630=CARTESIAN_POINT('Ctrl Pts',(207.849483299494,92.4272376097703,341.557589889321));
#27631=CARTESIAN_POINT('Ctrl Pts',(206.267108748143,92.3647376097703,342.893783236327));
#27632=CARTESIAN_POINT('Ctrl Pts',(204.684734196793,92.3022376097702,344.229976583334));
#27633=CARTESIAN_POINT('Ctrl Pts',(202.620995044512,92.2397376097702,344.055900184342));
#27634=CARTESIAN_POINT('Ctrl Pts',(200.55725589223,92.1772376097702,343.881823785349));
#27635=CARTESIAN_POINT('Ctrl Pts',(199.221062545224,92.1147376097703,342.299449233999));
#27636=CARTESIAN_POINT('Ctrl Pts',(197.884869198218,92.0522376097703,340.717074682649));
#27637=CARTESIAN_POINT('Ctrl Pts',(198.05894559721,91.9897376097702,338.653335530367));
#27638=CARTESIAN_POINT('Ctrl Pts',(198.233021996202,91.9272376097703,336.589596378086));
#27639=CARTESIAN_POINT('Ctrl Pts',(199.815396547552,91.8647376097702,335.253403031079));
#27640=CARTESIAN_POINT('Ctrl Pts',(201.397771098903,91.8022376097703,333.917209684073));
#27641=CARTESIAN_POINT('Ctrl Pts',(203.461510251184,91.7397376097703,334.091286083065));
#27642=CARTESIAN_POINT('Ctrl Pts',(205.525249403466,91.6772376097702,334.265362482058));
#27643=CARTESIAN_POINT('Ctrl Pts',(206.861442750472,91.6147376097702,335.847737033408));
#27644=CARTESIAN_POINT('Ctrl Pts',(208.197636097478,91.5522376097703,337.430111584758));
#27645=CARTESIAN_POINT('Ctrl Pts',(208.023559698486,91.4897376097703,339.49385073704));
#27646=CARTESIAN_POINT('Ctrl Pts',(207.849483299494,91.4272376097703,341.557589889321));
#27647=CARTESIAN_POINT('Ctrl Pts',(206.267108748143,91.3647376097702,342.893783236327));
#27648=CARTESIAN_POINT('Ctrl Pts',(204.684734196793,91.3022376097702,344.229976583334));
#27649=CARTESIAN_POINT('Ctrl Pts',(202.620995044512,91.2397376097702,344.055900184342));
#27650=CARTESIAN_POINT('Ctrl Pts',(200.55725589223,91.1772376097703,343.881823785349));
#27651=CARTESIAN_POINT('Ctrl Pts',(199.221062545224,91.1147376097703,342.299449233999));
#27652=CARTESIAN_POINT('Ctrl Pts',(197.884869198218,91.0522376097702,340.717074682649));
#27653=CARTESIAN_POINT('Ctrl Pts',(198.05894559721,90.9897376097702,338.653335530367));
#27654=CARTESIAN_POINT('Ctrl Pts',(198.233021996202,90.9272376097703,336.589596378086));
#27655=CARTESIAN_POINT('Ctrl Pts',(199.815396547552,90.8647376097703,335.253403031079));
#27656=CARTESIAN_POINT('Ctrl Pts',(201.397771098903,90.8022376097703,333.917209684073));
#27657=CARTESIAN_POINT('Ctrl Pts',(203.461510251184,90.7397376097702,334.091286083065));
#27658=CARTESIAN_POINT('Ctrl Pts',(205.525249403466,90.6772376097702,334.265362482058));
#27659=CARTESIAN_POINT('Ctrl Pts',(206.861442750472,90.6147376097702,335.847737033408));
#27660=CARTESIAN_POINT('Ctrl Pts',(208.197636097478,90.5522376097703,337.430111584758));
#27661=CARTESIAN_POINT('Ctrl Pts',(208.023559698486,90.4897376097703,339.49385073704));
#27662=CARTESIAN_POINT('Ctrl Pts',(207.849483299494,90.4272376097703,341.557589889321));
#27663=CARTESIAN_POINT('Ctrl Pts',(206.267108748143,90.3647376097702,342.893783236327));
#27664=CARTESIAN_POINT('Ctrl Pts',(204.684734196793,90.3022376097702,344.229976583334));
#27665=CARTESIAN_POINT('Ctrl Pts',(202.620995044512,90.2397376097703,344.055900184342));
#27666=CARTESIAN_POINT('Ctrl Pts',(200.55725589223,90.1772376097703,343.881823785349));
#27667=CARTESIAN_POINT('Ctrl Pts',(199.221062545224,90.1147376097702,342.299449233999));
#27668=CARTESIAN_POINT('Ctrl Pts',(197.884869198218,90.0522376097702,340.717074682649));
#27669=CARTESIAN_POINT('Ctrl Pts',(198.05894559721,89.9897376097702,338.653335530367));
#27670=CARTESIAN_POINT('Ctrl Pts',(198.233021996202,89.9272376097703,336.589596378086));
#27671=CARTESIAN_POINT('Ctrl Pts',(199.815396547552,89.8647376097703,335.253403031079));
#27672=CARTESIAN_POINT('Ctrl Pts',(201.397771098903,89.8022376097703,333.917209684073));
#27673=CARTESIAN_POINT('Ctrl Pts',(203.461510251184,89.7397376097702,334.091286083065));
#27674=CARTESIAN_POINT('Ctrl Pts',(205.525249403466,89.6772376097703,334.265362482058));
#27675=CARTESIAN_POINT('Ctrl Pts',(206.861442750472,89.6147376097703,335.847737033408));
#27676=CARTESIAN_POINT('Ctrl Pts',(208.197636097478,89.5522376097703,337.430111584758));
#27677=CARTESIAN_POINT('Ctrl Pts',(208.023559698486,89.4897376097702,339.49385073704));
#27678=CARTESIAN_POINT('Ctrl Pts',(207.849483299494,89.4272376097702,341.557589889321));
#27679=CARTESIAN_POINT('Ctrl Pts',(206.267108748143,89.3647376097702,342.893783236327));
#27680=CARTESIAN_POINT('Ctrl Pts',(204.684734196793,89.3022376097703,344.229976583334));
#27681=CARTESIAN_POINT('Ctrl Pts',(202.620995044512,89.2397376097703,344.055900184342));
#27682=CARTESIAN_POINT('Ctrl Pts',(200.55725589223,89.1772376097702,343.881823785349));
#27683=CARTESIAN_POINT('Ctrl Pts',(199.221062545224,89.1147376097702,342.299449233999));
#27684=CARTESIAN_POINT('Ctrl Pts',(197.884869198218,89.0522376097702,340.717074682649));
#27685=CARTESIAN_POINT('Ctrl Pts',(198.05894559721,88.9897376097703,338.653335530367));
#27686=CARTESIAN_POINT('Origin',(198.50948172921,94.0657194375285,329.433708166765));
#27687=CARTESIAN_POINT('Origin',(213.655523378095,94.0657194375285,339.968906877501));
#27688=CARTESIAN_POINT('Origin',(209.123752459458,94.0657194375285,330.329021910562));
#27689=CARTESIAN_POINT('Origin',(192.426981917601,94.0657194375285,338.178279389906));
#27690=CARTESIAN_POINT('Origin',(196.958752836238,94.0657194375285,347.818164356844));
#27691=CARTESIAN_POINT('Origin',(207.573023566486,94.0657194375285,348.713478100642));
#27775=UNCERTAINTY_MEASURE_WITH_UNIT(LENGTH_MEASURE(0.01),#27808,
'DISTANCE_ACCURACY_VALUE',
'Maximum model space distance between geometric entities at asserted c
onnectivities');
#27778=UNCERTAINTY_MEASURE_WITH_UNIT(LENGTH_MEASURE(0.01),#27808,
'DISTANCE_ACCURACY_VALUE',
'Maximum model space distance between geometric entities at asserted c
onnectivities');
#27804=(
GEOMETRIC_REPRESENTATION_CONTEXT(3)
GLOBAL_UNCERTAINTY_ASSIGNED_CONTEXT((#27775))
GLOBAL_UNIT_ASSIGNED_CONTEXT((#27808,#27810,#27811))
REPRESENTATION_CONTEXT('','3D')
);
#27807=(
GEOMETRIC_REPRESENTATION_CONTEXT(3)
GLOBAL_UNCERTAINTY_ASSIGNED_CONTEXT((#27778))
GLOBAL_UNIT_ASSIGNED_CONTEXT((#27808,#27810,#27811))
REPRESENTATION_CONTEXT('','3D')
);
#27808=(
LENGTH_UNIT()
NAMED_UNIT(*)
SI_UNIT(.MILLI.,.METRE.)
);
#27810=(
NAMED_UNIT(*)
PLANE_ANGLE_UNIT()
SI_UNIT($,.RADIAN.)
);
#27811=(
NAMED_UNIT(*)
SI_UNIT($,.STERADIAN.)
SOLID_ANGLE_UNIT()
);
#27837=SHAPE_DEFINITION_REPRESENTATION(#27883,#27924);
#27883=PRODUCT_DEFINITION_SHAPE('',$,#27953);
#27924=SHAPE_REPRESENTATION('',(#13515),#27804);
#27927=PRODUCT_DEFINITION_CONTEXT('part definition',#28013,'design');
#27953=PRODUCT_DEFINITION('Rear Caster Wheel','Rear Caster Wheel',#27981,
#27927);
#27981=PRODUCT_DEFINITION_FORMATION('',$,#28040);
#28013=APPLICATION_CONTEXT('Managed model based 3d engineering');
#28014=PRODUCT_CONTEXT('part definition',#28013,'mechanical');
#28040=PRODUCT('Rear Caster Wheel','Rear Caster Wheel',$,(#28014));
#28085=COLOUR_RGB('Off White',0.89,0.88,0.83);
#28086=FILL_AREA_STYLE_COLOUR('',#28085);
#28087=FILL_AREA_STYLE('',(#28086));
#28088=SURFACE_STYLE_FILL_AREA(#28087);
#28089=SURFACE_SIDE_STYLE('',(#28088));
#28090=SURFACE_STYLE_USAGE(.BOTH.,#28089);
#28091=PRESENTATION_STYLE_ASSIGNMENT((#28090));
ENDSEC;
END-ISO-10303-21;
